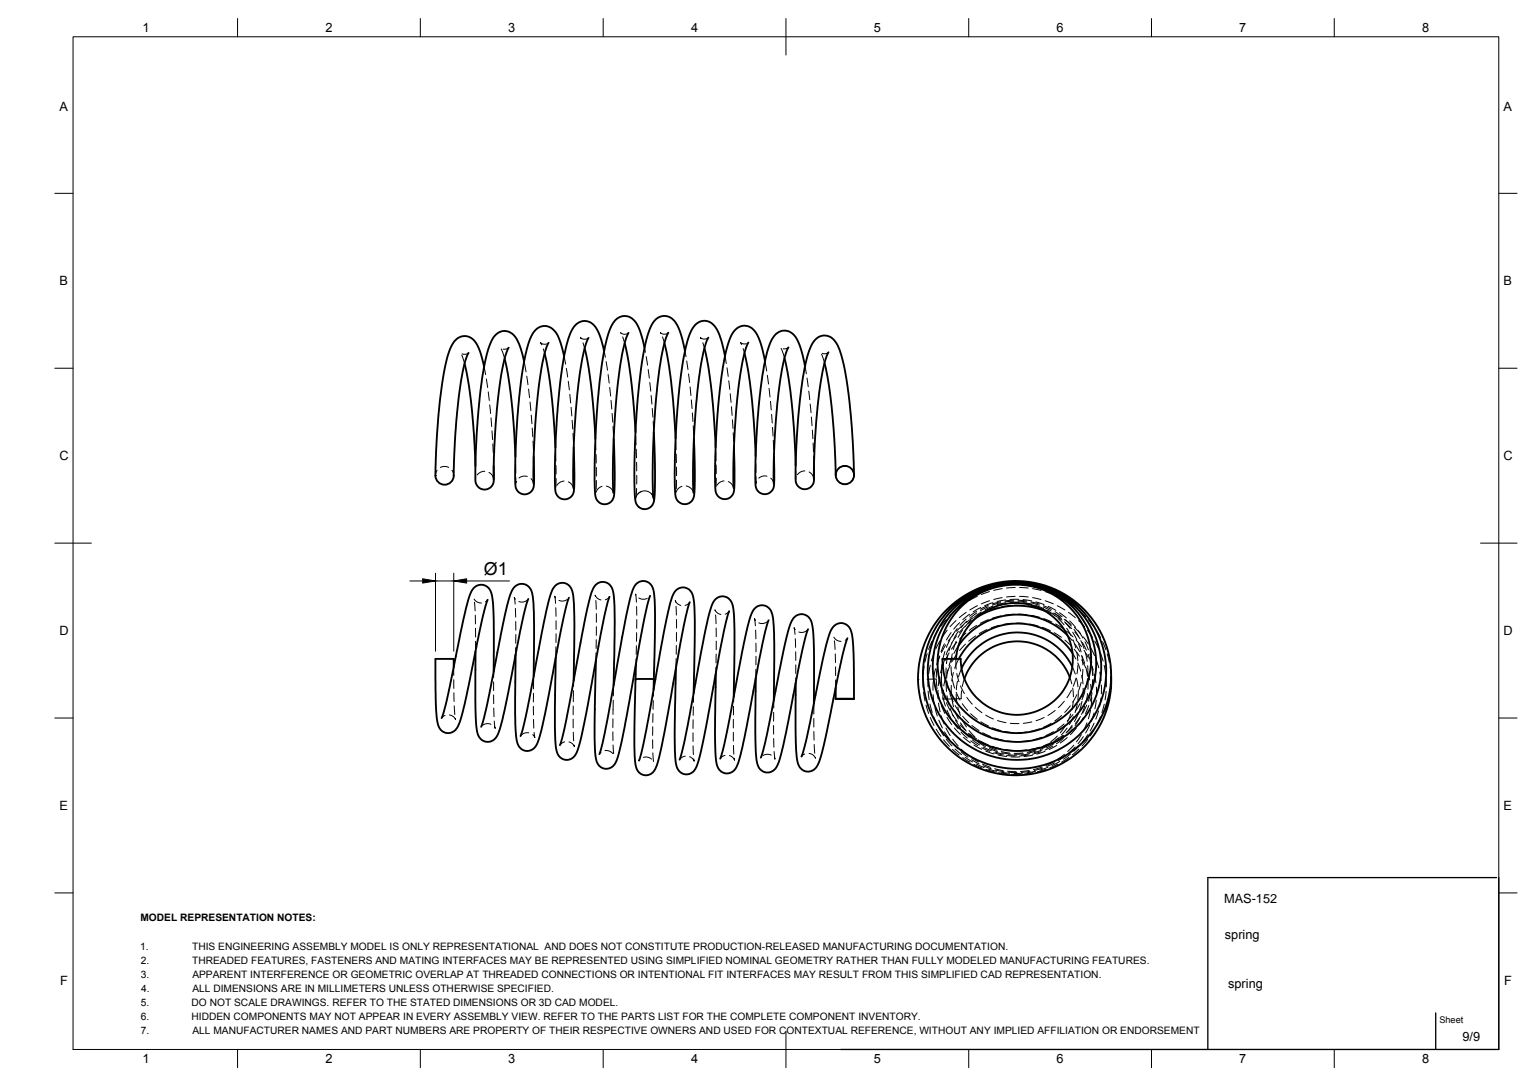
ISO-10303-21;
HEADER;
/* Generated by software containing ST-Developer
 * from STEP Tools, Inc. (www.steptools.com) 
 */

FILE_DESCRIPTION(
/* description */ ('STEP AP214'),
/* implementation_level */ '2;1');

FILE_NAME(
/* name */ 'spring.step',
/* time_stamp */ '2026-11-04T19:18:53-08:00',
/* author */ (''),
/* organization */ (''),
/* preprocessor_version */ 'ST-DEVELOPER v20.2',
/* originating_system */ 'Autodesk Translation Framework v15.17.0.0',
/* authorisation */ '');

FILE_SCHEMA (('AUTOMOTIVE_DESIGN { 1 0 10303 214 3 1 1 }'));
ENDSEC;

DATA;
#10=MECHANICAL_DESIGN_GEOMETRIC_PRESENTATION_REPRESENTATION('',(#80),#5942);
#55=B_SPLINE_CURVE_WITH_KNOTS('',3,(#2155,#2156,#2157,#2158,#2159,#2160,
#2161,#2162,#2163,#2164,#2165,#2166,#2167,#2168,#2169,#2170,#2171,#2172,
#2173,#2174,#2175,#2176,#2177,#2178,#2179,#2180,#2181,#2182,#2183,#2184,
#2185,#2186,#2187,#2188,#2189,#2190,#2191,#2192,#2193,#2194,#2195,#2196,
#2197,#2198,#2199,#2200,#2201,#2202,#2203,#2204,#2205,#2206,#2207,#2208,
#2209,#2210,#2211,#2212,#2213,#2214,#2215,#2216,#2217,#2218,#2219,#2220,
#2221,#2222,#2223,#2224,#2225,#2226,#2227,#2228,#2229,#2230,#2231,#2232,
#2233,#2234,#2235,#2236,#2237,#2238,#2239,#2240,#2241,#2242,#2243,#2244,
#2245,#2246,#2247,#2248,#2249,#2250,#2251,#2252,#2253,#2254,#2255,#2256,
#2257,#2258,#2259,#2260,#2261,#2262,#2263,#2264,#2265,#2266,#2267,#2268,
#2269,#2270,#2271,#2272,#2273,#2274,#2275,#2276,#2277,#2278,#2279,#2280,
#2281,#2282,#2283,#2284,#2285,#2286,#2287,#2288,#2289,#2290,#2291,#2292,
#2293,#2294,#2295,#2296,#2297,#2298,#2299,#2300,#2301,#2302,#2303,#2304,
#2305,#2306,#2307,#2308),.UNSPECIFIED.,.F.,.F.,(4,3,3,3,3,3,3,3,3,3,3,3,
3,3,3,3,3,3,3,3,3,3,3,3,3,3,3,3,3,3,3,3,3,3,3,3,3,3,3,3,3,3,3,3,3,3,3,3,
3,3,3,4),(8.16441129645516E-18,0.0155213821795324,0.0465641465385971,0.0776069108976618,
0.108649675256726,0.139692439615791,0.170735203974856,0.201777968333921,
0.232820732692985,0.26386349705205,0.294906261411162,0.325949025770274,
0.356991790129291,0.388034554488308,0.419077318847373,0.450120083206437,
0.46564146538597,0.481162847565502,0.496684229745034,0.512205611924566,
0.527726994104099,0.543248376283631,0.558769758463163,0.574291140642696,
0.589812522822228,0.605333905001761,0.620855287181293,0.636376669360825,
0.651898051540357,0.66741943371989,0.682940815899422,0.698462198078954,
0.713983580258487,0.729504962438019,0.745026344617551,0.760547726797084,
0.776069108976616,0.791590491156148,0.807111873335681,0.822633255515213,
0.838154637694745,0.853676019874278,0.86919740205381,0.884718784233342,
0.900240166412875,0.915761548592407,0.931282930771939,0.946804312951471,
0.973402156475736,0.986701078237868,0.993350539118934,0.993460673612188),
 .UNSPECIFIED.);
#56=B_SPLINE_CURVE_WITH_KNOTS('',3,(#2313,#2314,#2315,#2316,#2317,#2318,
#2319,#2320,#2321,#2322,#2323,#2324,#2325,#2326,#2327,#2328,#2329,#2330,
#2331,#2332,#2333,#2334,#2335,#2336,#2337,#2338,#2339,#2340,#2341,#2342,
#2343,#2344,#2345,#2346,#2347,#2348,#2349,#2350,#2351,#2352,#2353,#2354,
#2355,#2356,#2357,#2358,#2359,#2360,#2361,#2362,#2363,#2364,#2365,#2366,
#2367,#2368,#2369,#2370,#2371,#2372,#2373,#2374,#2375,#2376,#2377,#2378,
#2379,#2380,#2381,#2382,#2383,#2384,#2385,#2386,#2387,#2388,#2389,#2390,
#2391,#2392,#2393,#2394,#2395,#2396,#2397,#2398,#2399,#2400,#2401,#2402,
#2403,#2404,#2405,#2406,#2407,#2408,#2409,#2410,#2411,#2412,#2413,#2414,
#2415,#2416,#2417,#2418,#2419,#2420,#2421,#2422,#2423,#2424,#2425,#2426,
#2427,#2428,#2429,#2430,#2431,#2432,#2433,#2434,#2435,#2436,#2437,#2438,
#2439,#2440,#2441,#2442,#2443,#2444,#2445,#2446,#2447,#2448,#2449,#2450,
#2451,#2452,#2453,#2454,#2455,#2456,#2457,#2458,#2459,#2460,#2461,#2462,
#2463),.UNSPECIFIED.,.F.,.F.,(4,3,3,3,3,3,3,3,3,3,3,3,3,3,3,3,3,3,3,3,3,
3,3,3,3,3,3,3,3,3,3,3,3,3,3,3,3,3,3,3,3,3,3,3,3,3,3,3,3,3,4),(0.,0.0155213821795324,
0.0465641465385971,0.0776069108976618,0.108649675256726,0.139692439615791,
0.170735203974856,0.201777968333921,0.232820732692985,0.26386349705205,
0.294906261411162,0.325949025770274,0.356991790129291,0.388034554488308,
0.419077318847373,0.450120083206437,0.46564146538597,0.481162847565502,
0.496684229745034,0.512205611924566,0.527726994104099,0.543248376283631,
0.558769758463163,0.574291140642696,0.589812522822228,0.605333905001761,
0.620855287181293,0.636376669360825,0.651898051540357,0.66741943371989,
0.682940815899422,0.698462198078954,0.713983580258487,0.729504962438019,
0.745026344617551,0.760547726797084,0.776069108976616,0.791590491156148,
0.807111873335681,0.822633255515213,0.838154637694745,0.853676019874278,
0.86919740205381,0.884718784233342,0.900240166412875,0.915761548592407,
0.931282930771939,0.946804312951471,0.973402156475736,0.986701078237868,
0.993275477626297),.UNSPECIFIED.);
#57=B_SPLINE_CURVE_WITH_KNOTS('',3,(#3378,#3379,#3380,#3381,#3382,#3383,
#3384,#3385,#3386,#3387,#3388,#3389,#3390,#3391,#3392,#3393,#3394,#3395,
#3396,#3397,#3398,#3399,#3400,#3401,#3402,#3403,#3404,#3405,#3406,#3407,
#3408,#3409,#3410,#3411,#3412,#3413,#3414,#3415,#3416,#3417,#3418,#3419,
#3420,#3421,#3422,#3423,#3424,#3425,#3426,#3427,#3428,#3429,#3430,#3431,
#3432,#3433,#3434,#3435,#3436,#3437,#3438,#3439,#3440,#3441,#3442,#3443,
#3444,#3445,#3446,#3447,#3448,#3449,#3450,#3451,#3452,#3453,#3454,#3455,
#3456,#3457,#3458,#3459,#3460,#3461,#3462,#3463,#3464,#3465,#3466,#3467,
#3468,#3469,#3470,#3471,#3472,#3473,#3474,#3475,#3476,#3477,#3478,#3479,
#3480,#3481,#3482,#3483,#3484,#3485,#3486,#3487,#3488,#3489,#3490,#3491,
#3492,#3493,#3494,#3495,#3496,#3497,#3498,#3499,#3500,#3501,#3502,#3503,
#3504,#3505,#3506,#3507,#3508,#3509,#3510,#3511,#3512,#3513,#3514,#3515,
#3516,#3517,#3518,#3519,#3520,#3521,#3522,#3523,#3524,#3525,#3526,#3527,
#3528,#3529,#3530,#3531,#3532,#3533,#3534,#3535,#3536,#3537,#3538,#3539,
#3540,#3541,#3542,#3543,#3544,#3545,#3546,#3547,#3548,#3549,#3550,#3551,
#3552,#3553,#3554,#3555,#3556,#3557,#3558,#3559,#3560,#3561,#3562,#3563,
#3564,#3565,#3566,#3567,#3568,#3569,#3570),.UNSPECIFIED.,.F.,.F.,(4,3,3,
3,3,3,3,3,3,3,3,3,3,3,3,3,3,3,3,3,3,3,3,3,3,3,3,3,3,3,3,3,3,3,3,3,3,3,3,
3,3,3,3,3,3,3,3,3,3,3,3,3,3,3,3,3,3,3,3,3,3,3,3,3,4),(-3.92493609792139E-18,
0.015625,0.03125,0.046875,0.0625,0.078125,0.09375,0.109375,0.125,0.140625,
0.15625,0.171875,0.1875,0.203125,0.21875,0.234375,0.25,0.265625,0.28125,
0.296875,0.3125,0.328125,0.34375,0.359375,0.375,0.390625,0.40625,0.421875,
0.4375,0.453125,0.46875,0.484375,0.5,0.515625,0.53125,0.546875,0.5625,0.578125,
0.59375,0.609375,0.625,0.640625,0.65625,0.671875,0.6875,0.703125,0.71875,
0.734375,0.75,0.765625,0.78125,0.796875,0.8125,0.828125,0.84375,0.859375,
0.875,0.890625,0.90625,0.921875,0.9375,0.953125,0.96875,0.984375,1.),
 .UNSPECIFIED.);
#58=B_SPLINE_CURVE_WITH_KNOTS('',3,(#3572,#3573,#3574,#3575,#3576,#3577,
#3578,#3579,#3580,#3581,#3582,#3583,#3584,#3585,#3586,#3587,#3588,#3589,
#3590,#3591,#3592,#3593,#3594,#3595,#3596,#3597,#3598,#3599,#3600,#3601,
#3602,#3603,#3604,#3605,#3606,#3607,#3608,#3609,#3610,#3611,#3612,#3613,
#3614,#3615,#3616,#3617,#3618,#3619,#3620,#3621,#3622,#3623,#3624,#3625,
#3626,#3627,#3628,#3629,#3630,#3631,#3632,#3633,#3634,#3635,#3636,#3637,
#3638,#3639,#3640,#3641,#3642,#3643,#3644,#3645,#3646,#3647,#3648,#3649,
#3650,#3651,#3652,#3653,#3654,#3655,#3656,#3657,#3658,#3659,#3660,#3661,
#3662,#3663,#3664,#3665,#3666,#3667,#3668,#3669,#3670,#3671,#3672,#3673,
#3674,#3675,#3676,#3677,#3678,#3679,#3680,#3681,#3682,#3683,#3684,#3685,
#3686,#3687,#3688,#3689,#3690,#3691,#3692,#3693,#3694,#3695,#3696,#3697,
#3698,#3699,#3700,#3701,#3702,#3703,#3704,#3705,#3706,#3707,#3708,#3709,
#3710,#3711,#3712,#3713,#3714,#3715,#3716,#3717,#3718,#3719,#3720,#3721,
#3722,#3723,#3724,#3725,#3726,#3727,#3728,#3729,#3730,#3731,#3732,#3733,
#3734,#3735,#3736,#3737,#3738,#3739,#3740,#3741,#3742,#3743,#3744,#3745,
#3746,#3747,#3748,#3749,#3750,#3751,#3752,#3753,#3754,#3755,#3756,#3757,
#3758,#3759,#3760,#3761,#3762,#3763,#3764),.UNSPECIFIED.,.F.,.F.,(4,3,3,
3,3,3,3,3,3,3,3,3,3,3,3,3,3,3,3,3,3,3,3,3,3,3,3,3,3,3,3,3,3,3,3,3,3,3,3,
3,3,3,3,3,3,3,3,3,3,3,3,3,3,3,3,3,3,3,3,3,3,3,3,3,4),(0.,0.015625,0.03125,
0.046875,0.0625,0.078125,0.09375,0.109375,0.125,0.140625,0.15625,0.171875,
0.1875,0.203125,0.21875,0.234375,0.25,0.265625,0.28125,0.296875,0.3125,
0.328125,0.34375,0.359375,0.375,0.390625,0.40625,0.421875,0.4375,0.453125,
0.46875,0.484375,0.5,0.515625,0.53125,0.546875,0.5625,0.578125,0.59375,
0.609375,0.625,0.640625,0.65625,0.671875,0.6875,0.703125,0.71875,0.734375,
0.75,0.765625,0.78125,0.796875,0.8125,0.828125,0.84375,0.859375,0.875,0.890625,
0.90625,0.921875,0.9375,0.953125,0.96875,0.984375,1.),.UNSPECIFIED.);
#59=(
BOUNDED_SURFACE()
B_SPLINE_SURFACE(3,3,((#1423,#1424,#1425,#1426,#1427,#1428,#1429,#1430,
#1431,#1432,#1433,#1434,#1435,#1436,#1437,#1438,#1439,#1440,#1441,#1442,
#1443,#1444,#1445,#1446,#1447,#1448,#1449,#1450,#1451,#1452,#1453,#1454,
#1455,#1456,#1457,#1458,#1459,#1460,#1461,#1462,#1463,#1464,#1465,#1466,
#1467,#1468,#1469,#1470,#1471,#1472,#1473,#1474,#1475,#1476,#1477,#1478,
#1479,#1480,#1481,#1482,#1483,#1484,#1485,#1486,#1487,#1488,#1489,#1490,
#1491,#1492,#1493,#1494,#1495,#1496,#1497,#1498,#1499,#1500,#1501,#1502,
#1503,#1504,#1505,#1506,#1507,#1508,#1509,#1510,#1511,#1512,#1513,#1514,
#1515,#1516,#1517,#1518,#1519,#1520,#1521,#1522,#1523,#1524,#1525,#1526),
(#1527,#1528,#1529,#1530,#1531,#1532,#1533,#1534,#1535,#1536,#1537,#1538,
#1539,#1540,#1541,#1542,#1543,#1544,#1545,#1546,#1547,#1548,#1549,#1550,
#1551,#1552,#1553,#1554,#1555,#1556,#1557,#1558,#1559,#1560,#1561,#1562,
#1563,#1564,#1565,#1566,#1567,#1568,#1569,#1570,#1571,#1572,#1573,#1574,
#1575,#1576,#1577,#1578,#1579,#1580,#1581,#1582,#1583,#1584,#1585,#1586,
#1587,#1588,#1589,#1590,#1591,#1592,#1593,#1594,#1595,#1596,#1597,#1598,
#1599,#1600,#1601,#1602,#1603,#1604,#1605,#1606,#1607,#1608,#1609,#1610,
#1611,#1612,#1613,#1614,#1615,#1616,#1617,#1618,#1619,#1620,#1621,#1622,
#1623,#1624,#1625,#1626,#1627,#1628,#1629,#1630),(#1631,#1632,#1633,#1634,
#1635,#1636,#1637,#1638,#1639,#1640,#1641,#1642,#1643,#1644,#1645,#1646,
#1647,#1648,#1649,#1650,#1651,#1652,#1653,#1654,#1655,#1656,#1657,#1658,
#1659,#1660,#1661,#1662,#1663,#1664,#1665,#1666,#1667,#1668,#1669,#1670,
#1671,#1672,#1673,#1674,#1675,#1676,#1677,#1678,#1679,#1680,#1681,#1682,
#1683,#1684,#1685,#1686,#1687,#1688,#1689,#1690,#1691,#1692,#1693,#1694,
#1695,#1696,#1697,#1698,#1699,#1700,#1701,#1702,#1703,#1704,#1705,#1706,
#1707,#1708,#1709,#1710,#1711,#1712,#1713,#1714,#1715,#1716,#1717,#1718,
#1719,#1720,#1721,#1722,#1723,#1724,#1725,#1726,#1727,#1728,#1729,#1730,
#1731,#1732,#1733,#1734),(#1735,#1736,#1737,#1738,#1739,#1740,#1741,#1742,
#1743,#1744,#1745,#1746,#1747,#1748,#1749,#1750,#1751,#1752,#1753,#1754,
#1755,#1756,#1757,#1758,#1759,#1760,#1761,#1762,#1763,#1764,#1765,#1766,
#1767,#1768,#1769,#1770,#1771,#1772,#1773,#1774,#1775,#1776,#1777,#1778,
#1779,#1780,#1781,#1782,#1783,#1784,#1785,#1786,#1787,#1788,#1789,#1790,
#1791,#1792,#1793,#1794,#1795,#1796,#1797,#1798,#1799,#1800,#1801,#1802,
#1803,#1804,#1805,#1806,#1807,#1808,#1809,#1810,#1811,#1812,#1813,#1814,
#1815,#1816,#1817,#1818,#1819,#1820,#1821,#1822,#1823,#1824,#1825,#1826,
#1827,#1828,#1829,#1830,#1831,#1832,#1833,#1834,#1835,#1836,#1837,#1838),
(#1839,#1840,#1841,#1842,#1843,#1844,#1845,#1846,#1847,#1848,#1849,#1850,
#1851,#1852,#1853,#1854,#1855,#1856,#1857,#1858,#1859,#1860,#1861,#1862,
#1863,#1864,#1865,#1866,#1867,#1868,#1869,#1870,#1871,#1872,#1873,#1874,
#1875,#1876,#1877,#1878,#1879,#1880,#1881,#1882,#1883,#1884,#1885,#1886,
#1887,#1888,#1889,#1890,#1891,#1892,#1893,#1894,#1895,#1896,#1897,#1898,
#1899,#1900,#1901,#1902,#1903,#1904,#1905,#1906,#1907,#1908,#1909,#1910,
#1911,#1912,#1913,#1914,#1915,#1916,#1917,#1918,#1919,#1920,#1921,#1922,
#1923,#1924,#1925,#1926,#1927,#1928,#1929,#1930,#1931,#1932,#1933,#1934,
#1935,#1936,#1937,#1938,#1939,#1940,#1941,#1942),(#1943,#1944,#1945,#1946,
#1947,#1948,#1949,#1950,#1951,#1952,#1953,#1954,#1955,#1956,#1957,#1958,
#1959,#1960,#1961,#1962,#1963,#1964,#1965,#1966,#1967,#1968,#1969,#1970,
#1971,#1972,#1973,#1974,#1975,#1976,#1977,#1978,#1979,#1980,#1981,#1982,
#1983,#1984,#1985,#1986,#1987,#1988,#1989,#1990,#1991,#1992,#1993,#1994,
#1995,#1996,#1997,#1998,#1999,#2000,#2001,#2002,#2003,#2004,#2005,#2006,
#2007,#2008,#2009,#2010,#2011,#2012,#2013,#2014,#2015,#2016,#2017,#2018,
#2019,#2020,#2021,#2022,#2023,#2024,#2025,#2026,#2027,#2028,#2029,#2030,
#2031,#2032,#2033,#2034,#2035,#2036,#2037,#2038,#2039,#2040,#2041,#2042,
#2043,#2044,#2045,#2046),(#2047,#2048,#2049,#2050,#2051,#2052,#2053,#2054,
#2055,#2056,#2057,#2058,#2059,#2060,#2061,#2062,#2063,#2064,#2065,#2066,
#2067,#2068,#2069,#2070,#2071,#2072,#2073,#2074,#2075,#2076,#2077,#2078,
#2079,#2080,#2081,#2082,#2083,#2084,#2085,#2086,#2087,#2088,#2089,#2090,
#2091,#2092,#2093,#2094,#2095,#2096,#2097,#2098,#2099,#2100,#2101,#2102,
#2103,#2104,#2105,#2106,#2107,#2108,#2109,#2110,#2111,#2112,#2113,#2114,
#2115,#2116,#2117,#2118,#2119,#2120,#2121,#2122,#2123,#2124,#2125,#2126,
#2127,#2128,#2129,#2130,#2131,#2132,#2133,#2134,#2135,#2136,#2137,#2138,
#2139,#2140,#2141,#2142,#2143,#2144,#2145,#2146,#2147,#2148,#2149,#2150)),
 .UNSPECIFIED.,.T.,.F.,.F.)
B_SPLINE_SURFACE_WITH_KNOTS((4,3,4),(4,2,2,2,2,2,2,2,2,2,2,2,2,2,2,2,2,
2,2,2,2,2,2,2,2,2,2,2,2,2,2,2,2,2,2,2,2,2,2,2,2,2,2,2,2,2,2,2,2,2,2,4),
(0.,0.5,1.),(0.,0.0155213821795324,0.0465641465385971,0.0776069108976618,
0.108649675256726,0.139692439615791,0.170735203974856,0.201777968333921,
0.232820732692985,0.26386349705205,0.294906261411162,0.325949025770274,
0.356991790129291,0.388034554488308,0.419077318847373,0.450120083206437,
0.46564146538597,0.481162847565502,0.496684229745034,0.512205611924566,
0.527726994104099,0.543248376283631,0.558769758463163,0.574291140642696,
0.589812522822228,0.605333905001761,0.620855287181293,0.636376669360825,
0.651898051540357,0.66741943371989,0.682940815899422,0.698462198078954,
0.713983580258487,0.729504962438019,0.745026344617551,0.760547726797084,
0.776069108976616,0.791590491156148,0.807111873335681,0.822633255515213,
0.838154637694745,0.853676019874278,0.86919740205381,0.884718784233342,
0.900240166412875,0.915761548592407,0.931282930771939,0.946804312951471,
0.973402156475736,0.986701078237868,0.993350539118934,1.),.UNSPECIFIED.)
GEOMETRIC_REPRESENTATION_ITEM()
RATIONAL_B_SPLINE_SURFACE(((1.,1.,1.,1.,1.,1.,1.,1.,1.,1.,1.,1.,1.,1.,1.,
1.,1.,1.,1.,1.,1.,1.,1.,1.,1.,1.,1.,1.,1.,1.,1.,1.,1.,1.,1.,1.,1.,1.,1.,
1.,1.,1.,1.,1.,1.,1.,1.,1.,1.,1.,1.,1.,1.,1.,1.,1.,1.,1.,1.,1.,1.,1.,1.,
1.,1.,1.,1.,1.,1.,1.,1.,1.,1.,1.,1.,1.,1.,1.,1.,1.,1.,1.,1.,1.,1.,1.,1.,
1.,1.,1.,1.,1.,1.,1.,1.,1.,1.,1.,1.,1.,1.,1.,1.,1.),(0.333333333333333,
0.333333333333333,0.333333333333333,0.333333333333333,0.333333333333333,
0.333333333333333,0.333333333333333,0.333333333333333,0.333333333333333,
0.333333333333333,0.333333333333333,0.333333333333333,0.333333333333333,
0.333333333333333,0.333333333333333,0.333333333333333,0.333333333333333,
0.333333333333333,0.333333333333333,0.333333333333333,0.333333333333333,
0.333333333333333,0.333333333333333,0.333333333333333,0.333333333333333,
0.333333333333333,0.333333333333333,0.333333333333333,0.333333333333333,
0.333333333333333,0.333333333333333,0.333333333333333,0.333333333333333,
0.333333333333333,0.333333333333333,0.333333333333333,0.333333333333333,
0.333333333333333,0.333333333333333,0.333333333333333,0.333333333333333,
0.333333333333333,0.333333333333333,0.333333333333333,0.333333333333333,
0.333333333333333,0.333333333333333,0.333333333333333,0.333333333333333,
0.333333333333333,0.333333333333333,0.333333333333333,0.333333333333333,
0.333333333333333,0.333333333333333,0.333333333333333,0.333333333333333,
0.333333333333333,0.333333333333333,0.333333333333333,0.333333333333333,
0.333333333333333,0.333333333333333,0.333333333333333,0.333333333333333,
0.333333333333333,0.333333333333333,0.333333333333333,0.333333333333333,
0.333333333333333,0.333333333333333,0.333333333333333,0.333333333333333,
0.333333333333333,0.333333333333333,0.333333333333333,0.333333333333333,
0.333333333333333,0.333333333333333,0.333333333333333,0.333333333333333,
0.333333333333333,0.333333333333333,0.333333333333333,0.333333333333333,
0.333333333333333,0.333333333333333,0.333333333333333,0.333333333333333,
0.333333333333333,0.333333333333333,0.333333333333333,0.333333333333333,
0.333333333333333,0.333333333333333,0.333333333333333,0.333333333333333,
0.333333333333333,0.333333333333333,0.333333333333333,0.333333333333333,
0.333333333333333,0.333333333333333,0.333333333333333),(0.333333333333333,
0.333333333333333,0.333333333333333,0.333333333333333,0.333333333333333,
0.333333333333333,0.333333333333333,0.333333333333333,0.333333333333333,
0.333333333333333,0.333333333333333,0.333333333333333,0.333333333333333,
0.333333333333333,0.333333333333333,0.333333333333333,0.333333333333333,
0.333333333333333,0.333333333333333,0.333333333333333,0.333333333333333,
0.333333333333333,0.333333333333333,0.333333333333333,0.333333333333333,
0.333333333333333,0.333333333333333,0.333333333333333,0.333333333333333,
0.333333333333333,0.333333333333333,0.333333333333333,0.333333333333333,
0.333333333333333,0.333333333333333,0.333333333333333,0.333333333333333,
0.333333333333333,0.333333333333333,0.333333333333333,0.333333333333333,
0.333333333333333,0.333333333333333,0.333333333333333,0.333333333333333,
0.333333333333333,0.333333333333333,0.333333333333333,0.333333333333333,
0.333333333333333,0.333333333333333,0.333333333333333,0.333333333333333,
0.333333333333333,0.333333333333333,0.333333333333333,0.333333333333333,
0.333333333333333,0.333333333333333,0.333333333333333,0.333333333333333,
0.333333333333333,0.333333333333333,0.333333333333333,0.333333333333333,
0.333333333333333,0.333333333333333,0.333333333333333,0.333333333333333,
0.333333333333333,0.333333333333333,0.333333333333333,0.333333333333333,
0.333333333333333,0.333333333333333,0.333333333333333,0.333333333333333,
0.333333333333333,0.333333333333333,0.333333333333333,0.333333333333333,
0.333333333333333,0.333333333333333,0.333333333333333,0.333333333333333,
0.333333333333333,0.333333333333333,0.333333333333333,0.333333333333333,
0.333333333333333,0.333333333333333,0.333333333333333,0.333333333333333,
0.333333333333333,0.333333333333333,0.333333333333333,0.333333333333333,
0.333333333333333,0.333333333333333,0.333333333333333,0.333333333333333,
0.333333333333333,0.333333333333333,0.333333333333333),(1.,1.,1.,1.,1.,
1.,1.,1.,1.,1.,1.,1.,1.,1.,1.,1.,1.,1.,1.,1.,1.,1.,1.,1.,1.,1.,1.,1.,1.,
1.,1.,1.,1.,1.,1.,1.,1.,1.,1.,1.,1.,1.,1.,1.,1.,1.,1.,1.,1.,1.,1.,1.,1.,
1.,1.,1.,1.,1.,1.,1.,1.,1.,1.,1.,1.,1.,1.,1.,1.,1.,1.,1.,1.,1.,1.,1.,1.,
1.,1.,1.,1.,1.,1.,1.,1.,1.,1.,1.,1.,1.,1.,1.,1.,1.,1.,1.,1.,1.,1.,1.,1.,
1.,1.,1.),(0.333333333333333,0.333333333333333,0.333333333333333,0.333333333333333,
0.333333333333333,0.333333333333333,0.333333333333333,0.333333333333333,
0.333333333333333,0.333333333333333,0.333333333333333,0.333333333333333,
0.333333333333333,0.333333333333333,0.333333333333333,0.333333333333333,
0.333333333333333,0.333333333333333,0.333333333333333,0.333333333333333,
0.333333333333333,0.333333333333333,0.333333333333333,0.333333333333333,
0.333333333333333,0.333333333333333,0.333333333333333,0.333333333333333,
0.333333333333333,0.333333333333333,0.333333333333333,0.333333333333333,
0.333333333333333,0.333333333333333,0.333333333333333,0.333333333333333,
0.333333333333333,0.333333333333333,0.333333333333333,0.333333333333333,
0.333333333333333,0.333333333333333,0.333333333333333,0.333333333333333,
0.333333333333333,0.333333333333333,0.333333333333333,0.333333333333333,
0.333333333333333,0.333333333333333,0.333333333333333,0.333333333333333,
0.333333333333333,0.333333333333333,0.333333333333333,0.333333333333333,
0.333333333333333,0.333333333333333,0.333333333333333,0.333333333333333,
0.333333333333333,0.333333333333333,0.333333333333333,0.333333333333333,
0.333333333333333,0.333333333333333,0.333333333333333,0.333333333333333,
0.333333333333333,0.333333333333333,0.333333333333333,0.333333333333333,
0.333333333333333,0.333333333333333,0.333333333333333,0.333333333333333,
0.333333333333333,0.333333333333333,0.333333333333333,0.333333333333333,
0.333333333333333,0.333333333333333,0.333333333333333,0.333333333333333,
0.333333333333333,0.333333333333333,0.333333333333333,0.333333333333333,
0.333333333333333,0.333333333333333,0.333333333333333,0.333333333333333,
0.333333333333333,0.333333333333333,0.333333333333333,0.333333333333333,
0.333333333333333,0.333333333333333,0.333333333333333,0.333333333333333,
0.333333333333333,0.333333333333333,0.333333333333333,0.333333333333333),
(0.333333333333333,0.333333333333333,0.333333333333333,0.333333333333333,
0.333333333333333,0.333333333333333,0.333333333333333,0.333333333333333,
0.333333333333333,0.333333333333333,0.333333333333333,0.333333333333333,
0.333333333333333,0.333333333333333,0.333333333333333,0.333333333333333,
0.333333333333333,0.333333333333333,0.333333333333333,0.333333333333333,
0.333333333333333,0.333333333333333,0.333333333333333,0.333333333333333,
0.333333333333333,0.333333333333333,0.333333333333333,0.333333333333333,
0.333333333333333,0.333333333333333,0.333333333333333,0.333333333333333,
0.333333333333333,0.333333333333333,0.333333333333333,0.333333333333333,
0.333333333333333,0.333333333333333,0.333333333333333,0.333333333333333,
0.333333333333333,0.333333333333333,0.333333333333333,0.333333333333333,
0.333333333333333,0.333333333333333,0.333333333333333,0.333333333333333,
0.333333333333333,0.333333333333333,0.333333333333333,0.333333333333333,
0.333333333333333,0.333333333333333,0.333333333333333,0.333333333333333,
0.333333333333333,0.333333333333333,0.333333333333333,0.333333333333333,
0.333333333333333,0.333333333333333,0.333333333333333,0.333333333333333,
0.333333333333333,0.333333333333333,0.333333333333333,0.333333333333333,
0.333333333333333,0.333333333333333,0.333333333333333,0.333333333333333,
0.333333333333333,0.333333333333333,0.333333333333333,0.333333333333333,
0.333333333333333,0.333333333333333,0.333333333333333,0.333333333333333,
0.333333333333333,0.333333333333333,0.333333333333333,0.333333333333333,
0.333333333333333,0.333333333333333,0.333333333333333,0.333333333333333,
0.333333333333333,0.333333333333333,0.333333333333333,0.333333333333333,
0.333333333333333,0.333333333333333,0.333333333333333,0.333333333333333,
0.333333333333333,0.333333333333333,0.333333333333333,0.333333333333333,
0.333333333333333,0.333333333333333,0.333333333333333,0.333333333333333),
(1.,1.,1.,1.,1.,1.,1.,1.,1.,1.,1.,1.,1.,1.,1.,1.,1.,1.,1.,1.,1.,1.,1.,1.,
1.,1.,1.,1.,1.,1.,1.,1.,1.,1.,1.,1.,1.,1.,1.,1.,1.,1.,1.,1.,1.,1.,1.,1.,
1.,1.,1.,1.,1.,1.,1.,1.,1.,1.,1.,1.,1.,1.,1.,1.,1.,1.,1.,1.,1.,1.,1.,1.,
1.,1.,1.,1.,1.,1.,1.,1.,1.,1.,1.,1.,1.,1.,1.,1.,1.,1.,1.,1.,1.,1.,1.,1.,
1.,1.,1.,1.,1.,1.,1.,1.)))
REPRESENTATION_ITEM('')
SURFACE()
);
#60=(
BOUNDED_SURFACE()
B_SPLINE_SURFACE(3,3,((#2464,#2465,#2466,#2467,#2468,#2469,#2470,#2471,
#2472,#2473,#2474,#2475,#2476,#2477,#2478,#2479,#2480,#2481,#2482,#2483,
#2484,#2485,#2486,#2487,#2488,#2489,#2490,#2491,#2492,#2493,#2494,#2495,
#2496,#2497,#2498,#2499,#2500,#2501,#2502,#2503,#2504,#2505,#2506,#2507,
#2508,#2509,#2510,#2511,#2512,#2513,#2514,#2515,#2516,#2517,#2518,#2519,
#2520,#2521,#2522,#2523,#2524,#2525,#2526,#2527,#2528,#2529,#2530,#2531,
#2532,#2533,#2534,#2535,#2536,#2537,#2538,#2539,#2540,#2541,#2542,#2543,
#2544,#2545,#2546,#2547,#2548,#2549,#2550,#2551,#2552,#2553,#2554,#2555,
#2556,#2557,#2558,#2559,#2560,#2561,#2562,#2563,#2564,#2565,#2566,#2567,
#2568,#2569,#2570,#2571,#2572,#2573,#2574,#2575,#2576,#2577,#2578,#2579,
#2580,#2581,#2582,#2583,#2584,#2585,#2586,#2587,#2588,#2589,#2590,#2591,
#2592,#2593),(#2594,#2595,#2596,#2597,#2598,#2599,#2600,#2601,#2602,#2603,
#2604,#2605,#2606,#2607,#2608,#2609,#2610,#2611,#2612,#2613,#2614,#2615,
#2616,#2617,#2618,#2619,#2620,#2621,#2622,#2623,#2624,#2625,#2626,#2627,
#2628,#2629,#2630,#2631,#2632,#2633,#2634,#2635,#2636,#2637,#2638,#2639,
#2640,#2641,#2642,#2643,#2644,#2645,#2646,#2647,#2648,#2649,#2650,#2651,
#2652,#2653,#2654,#2655,#2656,#2657,#2658,#2659,#2660,#2661,#2662,#2663,
#2664,#2665,#2666,#2667,#2668,#2669,#2670,#2671,#2672,#2673,#2674,#2675,
#2676,#2677,#2678,#2679,#2680,#2681,#2682,#2683,#2684,#2685,#2686,#2687,
#2688,#2689,#2690,#2691,#2692,#2693,#2694,#2695,#2696,#2697,#2698,#2699,
#2700,#2701,#2702,#2703,#2704,#2705,#2706,#2707,#2708,#2709,#2710,#2711,
#2712,#2713,#2714,#2715,#2716,#2717,#2718,#2719,#2720,#2721,#2722,#2723),
(#2724,#2725,#2726,#2727,#2728,#2729,#2730,#2731,#2732,#2733,#2734,#2735,
#2736,#2737,#2738,#2739,#2740,#2741,#2742,#2743,#2744,#2745,#2746,#2747,
#2748,#2749,#2750,#2751,#2752,#2753,#2754,#2755,#2756,#2757,#2758,#2759,
#2760,#2761,#2762,#2763,#2764,#2765,#2766,#2767,#2768,#2769,#2770,#2771,
#2772,#2773,#2774,#2775,#2776,#2777,#2778,#2779,#2780,#2781,#2782,#2783,
#2784,#2785,#2786,#2787,#2788,#2789,#2790,#2791,#2792,#2793,#2794,#2795,
#2796,#2797,#2798,#2799,#2800,#2801,#2802,#2803,#2804,#2805,#2806,#2807,
#2808,#2809,#2810,#2811,#2812,#2813,#2814,#2815,#2816,#2817,#2818,#2819,
#2820,#2821,#2822,#2823,#2824,#2825,#2826,#2827,#2828,#2829,#2830,#2831,
#2832,#2833,#2834,#2835,#2836,#2837,#2838,#2839,#2840,#2841,#2842,#2843,
#2844,#2845,#2846,#2847,#2848,#2849,#2850,#2851,#2852,#2853),(#2854,#2855,
#2856,#2857,#2858,#2859,#2860,#2861,#2862,#2863,#2864,#2865,#2866,#2867,
#2868,#2869,#2870,#2871,#2872,#2873,#2874,#2875,#2876,#2877,#2878,#2879,
#2880,#2881,#2882,#2883,#2884,#2885,#2886,#2887,#2888,#2889,#2890,#2891,
#2892,#2893,#2894,#2895,#2896,#2897,#2898,#2899,#2900,#2901,#2902,#2903,
#2904,#2905,#2906,#2907,#2908,#2909,#2910,#2911,#2912,#2913,#2914,#2915,
#2916,#2917,#2918,#2919,#2920,#2921,#2922,#2923,#2924,#2925,#2926,#2927,
#2928,#2929,#2930,#2931,#2932,#2933,#2934,#2935,#2936,#2937,#2938,#2939,
#2940,#2941,#2942,#2943,#2944,#2945,#2946,#2947,#2948,#2949,#2950,#2951,
#2952,#2953,#2954,#2955,#2956,#2957,#2958,#2959,#2960,#2961,#2962,#2963,
#2964,#2965,#2966,#2967,#2968,#2969,#2970,#2971,#2972,#2973,#2974,#2975,
#2976,#2977,#2978,#2979,#2980,#2981,#2982,#2983),(#2984,#2985,#2986,#2987,
#2988,#2989,#2990,#2991,#2992,#2993,#2994,#2995,#2996,#2997,#2998,#2999,
#3000,#3001,#3002,#3003,#3004,#3005,#3006,#3007,#3008,#3009,#3010,#3011,
#3012,#3013,#3014,#3015,#3016,#3017,#3018,#3019,#3020,#3021,#3022,#3023,
#3024,#3025,#3026,#3027,#3028,#3029,#3030,#3031,#3032,#3033,#3034,#3035,
#3036,#3037,#3038,#3039,#3040,#3041,#3042,#3043,#3044,#3045,#3046,#3047,
#3048,#3049,#3050,#3051,#3052,#3053,#3054,#3055,#3056,#3057,#3058,#3059,
#3060,#3061,#3062,#3063,#3064,#3065,#3066,#3067,#3068,#3069,#3070,#3071,
#3072,#3073,#3074,#3075,#3076,#3077,#3078,#3079,#3080,#3081,#3082,#3083,
#3084,#3085,#3086,#3087,#3088,#3089,#3090,#3091,#3092,#3093,#3094,#3095,
#3096,#3097,#3098,#3099,#3100,#3101,#3102,#3103,#3104,#3105,#3106,#3107,
#3108,#3109,#3110,#3111,#3112,#3113),(#3114,#3115,#3116,#3117,#3118,#3119,
#3120,#3121,#3122,#3123,#3124,#3125,#3126,#3127,#3128,#3129,#3130,#3131,
#3132,#3133,#3134,#3135,#3136,#3137,#3138,#3139,#3140,#3141,#3142,#3143,
#3144,#3145,#3146,#3147,#3148,#3149,#3150,#3151,#3152,#3153,#3154,#3155,
#3156,#3157,#3158,#3159,#3160,#3161,#3162,#3163,#3164,#3165,#3166,#3167,
#3168,#3169,#3170,#3171,#3172,#3173,#3174,#3175,#3176,#3177,#3178,#3179,
#3180,#3181,#3182,#3183,#3184,#3185,#3186,#3187,#3188,#3189,#3190,#3191,
#3192,#3193,#3194,#3195,#3196,#3197,#3198,#3199,#3200,#3201,#3202,#3203,
#3204,#3205,#3206,#3207,#3208,#3209,#3210,#3211,#3212,#3213,#3214,#3215,
#3216,#3217,#3218,#3219,#3220,#3221,#3222,#3223,#3224,#3225,#3226,#3227,
#3228,#3229,#3230,#3231,#3232,#3233,#3234,#3235,#3236,#3237,#3238,#3239,
#3240,#3241,#3242,#3243),(#3244,#3245,#3246,#3247,#3248,#3249,#3250,#3251,
#3252,#3253,#3254,#3255,#3256,#3257,#3258,#3259,#3260,#3261,#3262,#3263,
#3264,#3265,#3266,#3267,#3268,#3269,#3270,#3271,#3272,#3273,#3274,#3275,
#3276,#3277,#3278,#3279,#3280,#3281,#3282,#3283,#3284,#3285,#3286,#3287,
#3288,#3289,#3290,#3291,#3292,#3293,#3294,#3295,#3296,#3297,#3298,#3299,
#3300,#3301,#3302,#3303,#3304,#3305,#3306,#3307,#3308,#3309,#3310,#3311,
#3312,#3313,#3314,#3315,#3316,#3317,#3318,#3319,#3320,#3321,#3322,#3323,
#3324,#3325,#3326,#3327,#3328,#3329,#3330,#3331,#3332,#3333,#3334,#3335,
#3336,#3337,#3338,#3339,#3340,#3341,#3342,#3343,#3344,#3345,#3346,#3347,
#3348,#3349,#3350,#3351,#3352,#3353,#3354,#3355,#3356,#3357,#3358,#3359,
#3360,#3361,#3362,#3363,#3364,#3365,#3366,#3367,#3368,#3369,#3370,#3371,
#3372,#3373)),.UNSPECIFIED.,.T.,.F.,.F.)
B_SPLINE_SURFACE_WITH_KNOTS((4,3,4),(4,2,2,2,2,2,2,2,2,2,2,2,2,2,2,2,2,
2,2,2,2,2,2,2,2,2,2,2,2,2,2,2,2,2,2,2,2,2,2,2,2,2,2,2,2,2,2,2,2,2,2,2,2,
2,2,2,2,2,2,2,2,2,2,2,4),(-6.51498550334715E-7,0.5,0.99999934850145),(0.,
0.015625,0.03125,0.046875,0.0625,0.078125,0.09375,0.109375,0.125,0.140625,
0.15625,0.171875,0.1875,0.203125,0.21875,0.234375,0.25,0.265625,0.28125,
0.296875,0.3125,0.328125,0.34375,0.359375,0.375,0.390625,0.40625,0.421875,
0.4375,0.453125,0.46875,0.484375,0.5,0.515625,0.53125,0.546875,0.5625,0.578125,
0.59375,0.609375,0.625,0.640625,0.65625,0.671875,0.6875,0.703125,0.71875,
0.734375,0.75,0.765625,0.78125,0.796875,0.8125,0.828125,0.84375,0.859375,
0.875,0.890625,0.90625,0.921875,0.9375,0.953125,0.96875,0.984375,1.),
 .UNSPECIFIED.)
GEOMETRIC_REPRESENTATION_ITEM()
RATIONAL_B_SPLINE_SURFACE(((0.999997394009194,0.999997394009194,0.999997394009194,
0.999997394009194,0.999997394009194,0.999997394009194,0.999997394009194,
0.999997394009194,0.999997394009194,0.999997394009194,0.999997394009194,
0.999997394009194,0.999997394009194,0.999997394009194,0.999997394009194,
0.999997394009194,0.999997394009194,0.999997394009194,0.999997394009194,
0.999997394009194,0.999997394009194,0.999997394009194,0.999997394009194,
0.999997394009194,0.999997394009194,0.999997394009194,0.999997394009194,
0.999997394009194,0.999997394009194,0.999997394009194,0.999997394009194,
0.999997394009194,0.999997394009194,0.999997394009194,0.999997394009194,
0.999997394009194,0.999997394009194,0.999997394009194,0.999997394009194,
0.999997394009194,0.999997394009194,0.999997394009194,0.999997394009194,
0.999997394009194,0.999997394009194,0.999997394009194,0.999997394009194,
0.999997394009194,0.999997394009194,0.999997394009194,0.999997394009194,
0.999997394009194,0.999997394009194,0.999997394009194,0.999997394009194,
0.999997394009194,0.999997394009194,0.999997394009194,0.999997394009194,
0.999997394009194,0.999997394009194,0.999997394009194,0.999997394009194,
0.999997394009194,0.999997394009194,0.999997394009194,0.999997394009194,
0.999997394009194,0.999997394009194,0.999997394009194,0.999997394009194,
0.999997394009194,0.999997394009194,0.999997394009194,0.999997394009194,
0.999997394009194,0.999997394009194,0.999997394009194,0.999997394009194,
0.999997394009194,0.999997394009194,0.999997394009194,0.999997394009194,
0.999997394009194,0.999997394009194,0.999997394009194,0.999997394009194,
0.999997394009194,0.999997394009194,0.999997394009194,0.999997394009194,
0.999997394009194,0.999997394009194,0.999997394009194,0.999997394009194,
0.999997394009194,0.999997394009194,0.999997394009194,0.999997394009194,
0.999997394009194,0.999997394009194,0.999997394009194,0.999997394009194,
0.999997394009194,0.999997394009194,0.999997394009194,0.999997394009194,
0.999997394009194,0.999997394009194,0.999997394009194,0.999997394009194,
0.999997394009194,0.999997394009194,0.999997394009194,0.999997394009194,
0.999997394009194,0.999997394009194,0.999997394009194,0.999997394009194,
0.999997394009194,0.999997394009194,0.999997394009194,0.999997394009194,
0.999997394009194,0.999997394009194,0.999997394009194,0.999997394009194,
0.999997394009194,0.999997394009194,0.999997394009194),(0.333333333333333,
0.333333333333333,0.333333333333333,0.333333333333333,0.333333333333333,
0.333333333333333,0.333333333333333,0.333333333333333,0.333333333333333,
0.333333333333333,0.333333333333333,0.333333333333333,0.333333333333333,
0.333333333333333,0.333333333333333,0.333333333333333,0.333333333333333,
0.333333333333333,0.333333333333333,0.333333333333333,0.333333333333333,
0.333333333333333,0.333333333333333,0.333333333333333,0.333333333333333,
0.333333333333333,0.333333333333333,0.333333333333333,0.333333333333333,
0.333333333333333,0.333333333333333,0.333333333333333,0.333333333333333,
0.333333333333333,0.333333333333333,0.333333333333333,0.333333333333333,
0.333333333333333,0.333333333333333,0.333333333333333,0.333333333333333,
0.333333333333333,0.333333333333333,0.333333333333333,0.333333333333333,
0.333333333333333,0.333333333333333,0.333333333333333,0.333333333333333,
0.333333333333333,0.333333333333333,0.333333333333333,0.333333333333333,
0.333333333333333,0.333333333333333,0.333333333333333,0.333333333333333,
0.333333333333333,0.333333333333333,0.333333333333333,0.333333333333333,
0.333333333333333,0.333333333333333,0.333333333333333,0.333333333333333,
0.333333333333333,0.333333333333333,0.333333333333333,0.333333333333333,
0.333333333333333,0.333333333333333,0.333333333333333,0.333333333333333,
0.333333333333333,0.333333333333333,0.333333333333333,0.333333333333333,
0.333333333333333,0.333333333333333,0.333333333333333,0.333333333333333,
0.333333333333333,0.333333333333333,0.333333333333333,0.333333333333333,
0.333333333333333,0.333333333333333,0.333333333333333,0.333333333333333,
0.333333333333333,0.333333333333333,0.333333333333333,0.333333333333333,
0.333333333333333,0.333333333333333,0.333333333333333,0.333333333333333,
0.333333333333333,0.333333333333333,0.333333333333333,0.333333333333333,
0.333333333333333,0.333333333333333,0.333333333333333,0.333333333333333,
0.333333333333333,0.333333333333333,0.333333333333333,0.333333333333333,
0.333333333333333,0.333333333333333,0.333333333333333,0.333333333333333,
0.333333333333333,0.333333333333333,0.333333333333333,0.333333333333333,
0.333333333333333,0.333333333333333,0.333333333333333,0.333333333333333,
0.333333333333333,0.333333333333333,0.333333333333333,0.333333333333333,
0.333333333333333,0.333333333333333,0.333333333333333,0.333333333333333,
0.333333333333333),(0.333333333333333,0.333333333333333,0.333333333333333,
0.333333333333333,0.333333333333333,0.333333333333333,0.333333333333333,
0.333333333333333,0.333333333333333,0.333333333333333,0.333333333333333,
0.333333333333333,0.333333333333333,0.333333333333333,0.333333333333333,
0.333333333333333,0.333333333333333,0.333333333333333,0.333333333333333,
0.333333333333333,0.333333333333333,0.333333333333333,0.333333333333333,
0.333333333333333,0.333333333333333,0.333333333333333,0.333333333333333,
0.333333333333333,0.333333333333333,0.333333333333333,0.333333333333333,
0.333333333333333,0.333333333333333,0.333333333333333,0.333333333333333,
0.333333333333333,0.333333333333333,0.333333333333333,0.333333333333333,
0.333333333333333,0.333333333333333,0.333333333333333,0.333333333333333,
0.333333333333333,0.333333333333333,0.333333333333333,0.333333333333333,
0.333333333333333,0.333333333333333,0.333333333333333,0.333333333333333,
0.333333333333333,0.333333333333333,0.333333333333333,0.333333333333333,
0.333333333333333,0.333333333333333,0.333333333333333,0.333333333333333,
0.333333333333333,0.333333333333333,0.333333333333333,0.333333333333333,
0.333333333333333,0.333333333333333,0.333333333333333,0.333333333333333,
0.333333333333333,0.333333333333333,0.333333333333333,0.333333333333333,
0.333333333333333,0.333333333333333,0.333333333333333,0.333333333333333,
0.333333333333333,0.333333333333333,0.333333333333333,0.333333333333333,
0.333333333333333,0.333333333333333,0.333333333333333,0.333333333333333,
0.333333333333333,0.333333333333333,0.333333333333333,0.333333333333333,
0.333333333333333,0.333333333333333,0.333333333333333,0.333333333333333,
0.333333333333333,0.333333333333333,0.333333333333333,0.333333333333333,
0.333333333333333,0.333333333333333,0.333333333333333,0.333333333333333,
0.333333333333333,0.333333333333333,0.333333333333333,0.333333333333333,
0.333333333333333,0.333333333333333,0.333333333333333,0.333333333333333,
0.333333333333333,0.333333333333333,0.333333333333333,0.333333333333333,
0.333333333333333,0.333333333333333,0.333333333333333,0.333333333333333,
0.333333333333333,0.333333333333333,0.333333333333333,0.333333333333333,
0.333333333333333,0.333333333333333,0.333333333333333,0.333333333333333,
0.333333333333333,0.333333333333333,0.333333333333333,0.333333333333333,
0.333333333333333,0.333333333333333,0.333333333333333),(1.,1.,1.,1.,1.,
1.,1.,1.,1.,1.,1.,1.,1.,1.,1.,1.,1.,1.,1.,1.,1.,1.,1.,1.,1.,1.,1.,1.,1.,
1.,1.,1.,1.,1.,1.,1.,1.,1.,1.,1.,1.,1.,1.,1.,1.,1.,1.,1.,1.,1.,1.,1.,1.,
1.,1.,1.,1.,1.,1.,1.,1.,1.,1.,1.,1.,1.,1.,1.,1.,1.,1.,1.,1.,1.,1.,1.,1.,
1.,1.,1.,1.,1.,1.,1.,1.,1.,1.,1.,1.,1.,1.,1.,1.,1.,1.,1.,1.,1.,1.,1.,1.,
1.,1.,1.,1.,1.,1.,1.,1.,1.,1.,1.,1.,1.,1.,1.,1.,1.,1.,1.,1.,1.,1.,1.,1.,
1.,1.,1.,1.,1.),(0.333334201998067,0.333334201998067,0.333334201998067,
0.333334201998067,0.333334201998067,0.333334201998067,0.333334201998067,
0.333334201998067,0.333334201998067,0.333334201998067,0.333334201998067,
0.333334201998067,0.333334201998067,0.333334201998067,0.333334201998067,
0.333334201998067,0.333334201998067,0.333334201998067,0.333334201998067,
0.333334201998067,0.333334201998067,0.333334201998067,0.333334201998067,
0.333334201998067,0.333334201998067,0.333334201998067,0.333334201998067,
0.333334201998067,0.333334201998067,0.333334201998067,0.333334201998067,
0.333334201998067,0.333334201998067,0.333334201998067,0.333334201998067,
0.333334201998067,0.333334201998067,0.333334201998067,0.333334201998067,
0.333334201998067,0.333334201998067,0.333334201998067,0.333334201998067,
0.333334201998067,0.333334201998067,0.333334201998067,0.333334201998067,
0.333334201998067,0.333334201998067,0.333334201998067,0.333334201998067,
0.333334201998067,0.333334201998067,0.333334201998067,0.333334201998067,
0.333334201998067,0.333334201998067,0.333334201998067,0.333334201998067,
0.333334201998067,0.333334201998067,0.333334201998067,0.333334201998067,
0.333334201998067,0.333334201998067,0.333334201998067,0.333334201998067,
0.333334201998067,0.333334201998067,0.333334201998067,0.333334201998067,
0.333334201998067,0.333334201998067,0.333334201998067,0.333334201998067,
0.333334201998067,0.333334201998067,0.333334201998067,0.333334201998067,
0.333334201998067,0.333334201998067,0.333334201998067,0.333334201998067,
0.333334201998067,0.333334201998067,0.333334201998067,0.333334201998067,
0.333334201998067,0.333334201998067,0.333334201998067,0.333334201998067,
0.333334201998067,0.333334201998067,0.333334201998067,0.333334201998067,
0.333334201998067,0.333334201998067,0.333334201998067,0.333334201998067,
0.333334201998067,0.333334201998067,0.333334201998067,0.333334201998067,
0.333334201998067,0.333334201998067,0.333334201998067,0.333334201998067,
0.333334201998067,0.333334201998067,0.333334201998067,0.333334201998067,
0.333334201998067,0.333334201998067,0.333334201998067,0.333334201998067,
0.333334201998067,0.333334201998067,0.333334201998067,0.333334201998067,
0.333334201998067,0.333334201998067,0.333334201998067,0.333334201998067,
0.333334201998067,0.333334201998067,0.333334201998067,0.333334201998067,
0.333334201998067,0.333334201998067,0.333334201998067),(0.333333333334465,
0.333333333334465,0.333333333334465,0.333333333334465,0.333333333334465,
0.333333333334465,0.333333333334465,0.333333333334465,0.333333333334465,
0.333333333334465,0.333333333334465,0.333333333334465,0.333333333334465,
0.333333333334465,0.333333333334465,0.333333333334465,0.333333333334465,
0.333333333334465,0.333333333334465,0.333333333334465,0.333333333334465,
0.333333333334465,0.333333333334465,0.333333333334465,0.333333333334465,
0.333333333334465,0.333333333334465,0.333333333334465,0.333333333334465,
0.333333333334465,0.333333333334465,0.333333333334465,0.333333333334465,
0.333333333334465,0.333333333334465,0.333333333334465,0.333333333334465,
0.333333333334465,0.333333333334465,0.333333333334465,0.333333333334465,
0.333333333334465,0.333333333334465,0.333333333334465,0.333333333334465,
0.333333333334465,0.333333333334465,0.333333333334465,0.333333333334465,
0.333333333334465,0.333333333334465,0.333333333334465,0.333333333334465,
0.333333333334465,0.333333333334465,0.333333333334465,0.333333333334465,
0.333333333334465,0.333333333334465,0.333333333334465,0.333333333334465,
0.333333333334465,0.333333333334465,0.333333333334465,0.333333333334465,
0.333333333334465,0.333333333334465,0.333333333334465,0.333333333334465,
0.333333333334465,0.333333333334465,0.333333333334465,0.333333333334465,
0.333333333334465,0.333333333334465,0.333333333334465,0.333333333334465,
0.333333333334465,0.333333333334465,0.333333333334465,0.333333333334465,
0.333333333334465,0.333333333334465,0.333333333334465,0.333333333334465,
0.333333333334465,0.333333333334465,0.333333333334465,0.333333333334465,
0.333333333334465,0.333333333334465,0.333333333334465,0.333333333334465,
0.333333333334465,0.333333333334465,0.333333333334465,0.333333333334465,
0.333333333334465,0.333333333334465,0.333333333334465,0.333333333334465,
0.333333333334465,0.333333333334465,0.333333333334465,0.333333333334465,
0.333333333334465,0.333333333334465,0.333333333334465,0.333333333334465,
0.333333333334465,0.333333333334465,0.333333333334465,0.333333333334465,
0.333333333334465,0.333333333334465,0.333333333334465,0.333333333334465,
0.333333333334465,0.333333333334465,0.333333333334465,0.333333333334465,
0.333333333334465,0.333333333334465,0.333333333334465,0.333333333334465,
0.333333333334465,0.333333333334465,0.333333333334465,0.333333333334465,
0.333333333334465),(0.999997394009194,0.999997394009194,0.999997394009194,
0.999997394009194,0.999997394009194,0.999997394009194,0.999997394009194,
0.999997394009194,0.999997394009194,0.999997394009194,0.999997394009194,
0.999997394009194,0.999997394009194,0.999997394009194,0.999997394009194,
0.999997394009194,0.999997394009194,0.999997394009194,0.999997394009194,
0.999997394009194,0.999997394009194,0.999997394009194,0.999997394009194,
0.999997394009194,0.999997394009194,0.999997394009194,0.999997394009194,
0.999997394009194,0.999997394009194,0.999997394009194,0.999997394009194,
0.999997394009194,0.999997394009194,0.999997394009194,0.999997394009194,
0.999997394009194,0.999997394009194,0.999997394009194,0.999997394009194,
0.999997394009194,0.999997394009194,0.999997394009194,0.999997394009194,
0.999997394009194,0.999997394009194,0.999997394009194,0.999997394009194,
0.999997394009194,0.999997394009194,0.999997394009194,0.999997394009194,
0.999997394009194,0.999997394009194,0.999997394009194,0.999997394009194,
0.999997394009194,0.999997394009194,0.999997394009194,0.999997394009194,
0.999997394009194,0.999997394009194,0.999997394009194,0.999997394009194,
0.999997394009194,0.999997394009194,0.999997394009194,0.999997394009194,
0.999997394009194,0.999997394009194,0.999997394009194,0.999997394009194,
0.999997394009194,0.999997394009194,0.999997394009194,0.999997394009194,
0.999997394009194,0.999997394009194,0.999997394009194,0.999997394009194,
0.999997394009194,0.999997394009194,0.999997394009194,0.999997394009194,
0.999997394009194,0.999997394009194,0.999997394009194,0.999997394009194,
0.999997394009194,0.999997394009194,0.999997394009194,0.999997394009194,
0.999997394009194,0.999997394009194,0.999997394009194,0.999997394009194,
0.999997394009194,0.999997394009194,0.999997394009194,0.999997394009194,
0.999997394009194,0.999997394009194,0.999997394009194,0.999997394009194,
0.999997394009194,0.999997394009194,0.999997394009194,0.999997394009194,
0.999997394009194,0.999997394009194,0.999997394009194,0.999997394009194,
0.999997394009194,0.999997394009194,0.999997394009194,0.999997394009194,
0.999997394009194,0.999997394009194,0.999997394009194,0.999997394009194,
0.999997394009194,0.999997394009194,0.999997394009194,0.999997394009194,
0.999997394009194,0.999997394009194,0.999997394009194,0.999997394009194,
0.999997394009194,0.999997394009194,0.999997394009194)))
REPRESENTATION_ITEM('')
SURFACE()
);
#61=(
BOUNDED_SURFACE()
B_SPLINE_SURFACE(3,3,((#3765,#3766,#3767,#3768,#3769,#3770,#3771,#3772,
#3773,#3774,#3775,#3776,#3777,#3778,#3779,#3780,#3781,#3782,#3783,#3784,
#3785,#3786,#3787,#3788,#3789,#3790,#3791,#3792,#3793,#3794,#3795,#3796,
#3797,#3798,#3799,#3800,#3801,#3802,#3803,#3804,#3805,#3806,#3807,#3808,
#3809,#3810,#3811,#3812,#3813,#3814,#3815,#3816,#3817,#3818,#3819,#3820,
#3821,#3822,#3823,#3824,#3825,#3826,#3827,#3828,#3829,#3830,#3831,#3832,
#3833,#3834,#3835,#3836,#3837,#3838,#3839,#3840,#3841,#3842,#3843,#3844,
#3845,#3846,#3847,#3848,#3849,#3850,#3851,#3852,#3853,#3854,#3855,#3856,
#3857,#3858,#3859,#3860,#3861,#3862,#3863,#3864,#3865,#3866,#3867,#3868,
#3869,#3870,#3871,#3872,#3873,#3874,#3875,#3876,#3877,#3878,#3879,#3880,
#3881,#3882,#3883,#3884,#3885,#3886,#3887,#3888,#3889,#3890,#3891,#3892,
#3893,#3894),(#3895,#3896,#3897,#3898,#3899,#3900,#3901,#3902,#3903,#3904,
#3905,#3906,#3907,#3908,#3909,#3910,#3911,#3912,#3913,#3914,#3915,#3916,
#3917,#3918,#3919,#3920,#3921,#3922,#3923,#3924,#3925,#3926,#3927,#3928,
#3929,#3930,#3931,#3932,#3933,#3934,#3935,#3936,#3937,#3938,#3939,#3940,
#3941,#3942,#3943,#3944,#3945,#3946,#3947,#3948,#3949,#3950,#3951,#3952,
#3953,#3954,#3955,#3956,#3957,#3958,#3959,#3960,#3961,#3962,#3963,#3964,
#3965,#3966,#3967,#3968,#3969,#3970,#3971,#3972,#3973,#3974,#3975,#3976,
#3977,#3978,#3979,#3980,#3981,#3982,#3983,#3984,#3985,#3986,#3987,#3988,
#3989,#3990,#3991,#3992,#3993,#3994,#3995,#3996,#3997,#3998,#3999,#4000,
#4001,#4002,#4003,#4004,#4005,#4006,#4007,#4008,#4009,#4010,#4011,#4012,
#4013,#4014,#4015,#4016,#4017,#4018,#4019,#4020,#4021,#4022,#4023,#4024),
(#4025,#4026,#4027,#4028,#4029,#4030,#4031,#4032,#4033,#4034,#4035,#4036,
#4037,#4038,#4039,#4040,#4041,#4042,#4043,#4044,#4045,#4046,#4047,#4048,
#4049,#4050,#4051,#4052,#4053,#4054,#4055,#4056,#4057,#4058,#4059,#4060,
#4061,#4062,#4063,#4064,#4065,#4066,#4067,#4068,#4069,#4070,#4071,#4072,
#4073,#4074,#4075,#4076,#4077,#4078,#4079,#4080,#4081,#4082,#4083,#4084,
#4085,#4086,#4087,#4088,#4089,#4090,#4091,#4092,#4093,#4094,#4095,#4096,
#4097,#4098,#4099,#4100,#4101,#4102,#4103,#4104,#4105,#4106,#4107,#4108,
#4109,#4110,#4111,#4112,#4113,#4114,#4115,#4116,#4117,#4118,#4119,#4120,
#4121,#4122,#4123,#4124,#4125,#4126,#4127,#4128,#4129,#4130,#4131,#4132,
#4133,#4134,#4135,#4136,#4137,#4138,#4139,#4140,#4141,#4142,#4143,#4144,
#4145,#4146,#4147,#4148,#4149,#4150,#4151,#4152,#4153,#4154),(#4155,#4156,
#4157,#4158,#4159,#4160,#4161,#4162,#4163,#4164,#4165,#4166,#4167,#4168,
#4169,#4170,#4171,#4172,#4173,#4174,#4175,#4176,#4177,#4178,#4179,#4180,
#4181,#4182,#4183,#4184,#4185,#4186,#4187,#4188,#4189,#4190,#4191,#4192,
#4193,#4194,#4195,#4196,#4197,#4198,#4199,#4200,#4201,#4202,#4203,#4204,
#4205,#4206,#4207,#4208,#4209,#4210,#4211,#4212,#4213,#4214,#4215,#4216,
#4217,#4218,#4219,#4220,#4221,#4222,#4223,#4224,#4225,#4226,#4227,#4228,
#4229,#4230,#4231,#4232,#4233,#4234,#4235,#4236,#4237,#4238,#4239,#4240,
#4241,#4242,#4243,#4244,#4245,#4246,#4247,#4248,#4249,#4250,#4251,#4252,
#4253,#4254,#4255,#4256,#4257,#4258,#4259,#4260,#4261,#4262,#4263,#4264,
#4265,#4266,#4267,#4268,#4269,#4270,#4271,#4272,#4273,#4274,#4275,#4276,
#4277,#4278,#4279,#4280,#4281,#4282,#4283,#4284),(#4285,#4286,#4287,#4288,
#4289,#4290,#4291,#4292,#4293,#4294,#4295,#4296,#4297,#4298,#4299,#4300,
#4301,#4302,#4303,#4304,#4305,#4306,#4307,#4308,#4309,#4310,#4311,#4312,
#4313,#4314,#4315,#4316,#4317,#4318,#4319,#4320,#4321,#4322,#4323,#4324,
#4325,#4326,#4327,#4328,#4329,#4330,#4331,#4332,#4333,#4334,#4335,#4336,
#4337,#4338,#4339,#4340,#4341,#4342,#4343,#4344,#4345,#4346,#4347,#4348,
#4349,#4350,#4351,#4352,#4353,#4354,#4355,#4356,#4357,#4358,#4359,#4360,
#4361,#4362,#4363,#4364,#4365,#4366,#4367,#4368,#4369,#4370,#4371,#4372,
#4373,#4374,#4375,#4376,#4377,#4378,#4379,#4380,#4381,#4382,#4383,#4384,
#4385,#4386,#4387,#4388,#4389,#4390,#4391,#4392,#4393,#4394,#4395,#4396,
#4397,#4398,#4399,#4400,#4401,#4402,#4403,#4404,#4405,#4406,#4407,#4408,
#4409,#4410,#4411,#4412,#4413,#4414),(#4415,#4416,#4417,#4418,#4419,#4420,
#4421,#4422,#4423,#4424,#4425,#4426,#4427,#4428,#4429,#4430,#4431,#4432,
#4433,#4434,#4435,#4436,#4437,#4438,#4439,#4440,#4441,#4442,#4443,#4444,
#4445,#4446,#4447,#4448,#4449,#4450,#4451,#4452,#4453,#4454,#4455,#4456,
#4457,#4458,#4459,#4460,#4461,#4462,#4463,#4464,#4465,#4466,#4467,#4468,
#4469,#4470,#4471,#4472,#4473,#4474,#4475,#4476,#4477,#4478,#4479,#4480,
#4481,#4482,#4483,#4484,#4485,#4486,#4487,#4488,#4489,#4490,#4491,#4492,
#4493,#4494,#4495,#4496,#4497,#4498,#4499,#4500,#4501,#4502,#4503,#4504,
#4505,#4506,#4507,#4508,#4509,#4510,#4511,#4512,#4513,#4514,#4515,#4516,
#4517,#4518,#4519,#4520,#4521,#4522,#4523,#4524,#4525,#4526,#4527,#4528,
#4529,#4530,#4531,#4532,#4533,#4534,#4535,#4536,#4537,#4538,#4539,#4540,
#4541,#4542,#4543,#4544),(#4545,#4546,#4547,#4548,#4549,#4550,#4551,#4552,
#4553,#4554,#4555,#4556,#4557,#4558,#4559,#4560,#4561,#4562,#4563,#4564,
#4565,#4566,#4567,#4568,#4569,#4570,#4571,#4572,#4573,#4574,#4575,#4576,
#4577,#4578,#4579,#4580,#4581,#4582,#4583,#4584,#4585,#4586,#4587,#4588,
#4589,#4590,#4591,#4592,#4593,#4594,#4595,#4596,#4597,#4598,#4599,#4600,
#4601,#4602,#4603,#4604,#4605,#4606,#4607,#4608,#4609,#4610,#4611,#4612,
#4613,#4614,#4615,#4616,#4617,#4618,#4619,#4620,#4621,#4622,#4623,#4624,
#4625,#4626,#4627,#4628,#4629,#4630,#4631,#4632,#4633,#4634,#4635,#4636,
#4637,#4638,#4639,#4640,#4641,#4642,#4643,#4644,#4645,#4646,#4647,#4648,
#4649,#4650,#4651,#4652,#4653,#4654,#4655,#4656,#4657,#4658,#4659,#4660,
#4661,#4662,#4663,#4664,#4665,#4666,#4667,#4668,#4669,#4670,#4671,#4672,
#4673,#4674)),.UNSPECIFIED.,.T.,.F.,.F.)
B_SPLINE_SURFACE_WITH_KNOTS((4,3,4),(4,2,2,2,2,2,2,2,2,2,2,2,2,2,2,2,2,
2,2,2,2,2,2,2,2,2,2,2,2,2,2,2,2,2,2,2,2,2,2,2,2,2,2,2,2,2,2,2,2,2,2,2,2,
2,2,2,2,2,2,2,2,2,2,2,4),(0.499999335657285,1.,1.49999933565728),(0.,0.015625,
0.03125,0.046875,0.0625,0.078125,0.09375,0.109375,0.125,0.140625,0.15625,
0.171875,0.1875,0.203125,0.21875,0.234375,0.25,0.265625,0.28125,0.296875,
0.3125,0.328125,0.34375,0.359375,0.375,0.390625,0.40625,0.421875,0.4375,
0.453125,0.46875,0.484375,0.5,0.515625,0.53125,0.546875,0.5625,0.578125,
0.59375,0.609375,0.625,0.640625,0.65625,0.671875,0.6875,0.703125,0.71875,
0.734375,0.75,0.765625,0.78125,0.796875,0.8125,0.828125,0.84375,0.859375,
0.875,0.890625,0.90625,0.921875,0.9375,0.953125,0.96875,0.984375,1.),
 .UNSPECIFIED.)
GEOMETRIC_REPRESENTATION_ITEM()
RATIONAL_B_SPLINE_SURFACE(((0.999997342632669,0.999997342632669,0.999997342632669,
0.999997342632669,0.999997342632669,0.999997342632669,0.999997342632669,
0.999997342632669,0.999997342632669,0.999997342632669,0.999997342632669,
0.999997342632669,0.999997342632669,0.999997342632669,0.999997342632669,
0.999997342632669,0.999997342632669,0.999997342632669,0.999997342632669,
0.999997342632669,0.999997342632669,0.999997342632669,0.999997342632669,
0.999997342632669,0.999997342632669,0.999997342632669,0.999997342632669,
0.999997342632669,0.999997342632669,0.999997342632669,0.999997342632669,
0.999997342632669,0.999997342632669,0.999997342632669,0.999997342632669,
0.999997342632669,0.999997342632669,0.999997342632669,0.999997342632669,
0.999997342632669,0.999997342632669,0.999997342632669,0.999997342632669,
0.999997342632669,0.999997342632669,0.999997342632669,0.999997342632669,
0.999997342632669,0.999997342632669,0.999997342632669,0.999997342632669,
0.999997342632669,0.999997342632669,0.999997342632669,0.999997342632669,
0.999997342632669,0.999997342632669,0.999997342632669,0.999997342632669,
0.999997342632669,0.999997342632669,0.999997342632669,0.999997342632669,
0.999997342632669,0.999997342632669,0.999997342632669,0.999997342632669,
0.999997342632669,0.999997342632669,0.999997342632669,0.999997342632669,
0.999997342632669,0.999997342632669,0.999997342632669,0.999997342632669,
0.999997342632669,0.999997342632669,0.999997342632669,0.999997342632669,
0.999997342632669,0.999997342632669,0.999997342632669,0.999997342632669,
0.999997342632669,0.999997342632669,0.999997342632669,0.999997342632669,
0.999997342632669,0.999997342632669,0.999997342632669,0.999997342632669,
0.999997342632669,0.999997342632669,0.999997342632669,0.999997342632669,
0.999997342632669,0.999997342632669,0.999997342632669,0.999997342632669,
0.999997342632669,0.999997342632669,0.999997342632669,0.999997342632669,
0.999997342632669,0.999997342632669,0.999997342632669,0.999997342632669,
0.999997342632669,0.999997342632669,0.999997342632669,0.999997342632669,
0.999997342632669,0.999997342632669,0.999997342632669,0.999997342632669,
0.999997342632669,0.999997342632669,0.999997342632669,0.999997342632669,
0.999997342632669,0.999997342632669,0.999997342632669,0.999997342632669,
0.999997342632669,0.999997342632669,0.999997342632669,0.999997342632669,
0.999997342632669,0.999997342632669,0.999997342632669),(0.333333333333333,
0.333333333333333,0.333333333333333,0.333333333333333,0.333333333333333,
0.333333333333333,0.333333333333333,0.333333333333333,0.333333333333333,
0.333333333333333,0.333333333333333,0.333333333333333,0.333333333333333,
0.333333333333333,0.333333333333333,0.333333333333333,0.333333333333333,
0.333333333333333,0.333333333333333,0.333333333333333,0.333333333333333,
0.333333333333333,0.333333333333333,0.333333333333333,0.333333333333333,
0.333333333333333,0.333333333333333,0.333333333333333,0.333333333333333,
0.333333333333333,0.333333333333333,0.333333333333333,0.333333333333333,
0.333333333333333,0.333333333333333,0.333333333333333,0.333333333333333,
0.333333333333333,0.333333333333333,0.333333333333333,0.333333333333333,
0.333333333333333,0.333333333333333,0.333333333333333,0.333333333333333,
0.333333333333333,0.333333333333333,0.333333333333333,0.333333333333333,
0.333333333333333,0.333333333333333,0.333333333333333,0.333333333333333,
0.333333333333333,0.333333333333333,0.333333333333333,0.333333333333333,
0.333333333333333,0.333333333333333,0.333333333333333,0.333333333333333,
0.333333333333333,0.333333333333333,0.333333333333333,0.333333333333333,
0.333333333333333,0.333333333333333,0.333333333333333,0.333333333333333,
0.333333333333333,0.333333333333333,0.333333333333333,0.333333333333333,
0.333333333333333,0.333333333333333,0.333333333333333,0.333333333333333,
0.333333333333333,0.333333333333333,0.333333333333333,0.333333333333333,
0.333333333333333,0.333333333333333,0.333333333333333,0.333333333333333,
0.333333333333333,0.333333333333333,0.333333333333333,0.333333333333333,
0.333333333333333,0.333333333333333,0.333333333333333,0.333333333333333,
0.333333333333333,0.333333333333333,0.333333333333333,0.333333333333333,
0.333333333333333,0.333333333333333,0.333333333333333,0.333333333333333,
0.333333333333333,0.333333333333333,0.333333333333333,0.333333333333333,
0.333333333333333,0.333333333333333,0.333333333333333,0.333333333333333,
0.333333333333333,0.333333333333333,0.333333333333333,0.333333333333333,
0.333333333333333,0.333333333333333,0.333333333333333,0.333333333333333,
0.333333333333333,0.333333333333333,0.333333333333333,0.333333333333333,
0.333333333333333,0.333333333333333,0.333333333333333,0.333333333333333,
0.333333333333333,0.333333333333333,0.333333333333333,0.333333333333333,
0.333333333333333),(0.333333333333333,0.333333333333333,0.333333333333333,
0.333333333333333,0.333333333333333,0.333333333333333,0.333333333333333,
0.333333333333333,0.333333333333333,0.333333333333333,0.333333333333333,
0.333333333333333,0.333333333333333,0.333333333333333,0.333333333333333,
0.333333333333333,0.333333333333333,0.333333333333333,0.333333333333333,
0.333333333333333,0.333333333333333,0.333333333333333,0.333333333333333,
0.333333333333333,0.333333333333333,0.333333333333333,0.333333333333333,
0.333333333333333,0.333333333333333,0.333333333333333,0.333333333333333,
0.333333333333333,0.333333333333333,0.333333333333333,0.333333333333333,
0.333333333333333,0.333333333333333,0.333333333333333,0.333333333333333,
0.333333333333333,0.333333333333333,0.333333333333333,0.333333333333333,
0.333333333333333,0.333333333333333,0.333333333333333,0.333333333333333,
0.333333333333333,0.333333333333333,0.333333333333333,0.333333333333333,
0.333333333333333,0.333333333333333,0.333333333333333,0.333333333333333,
0.333333333333333,0.333333333333333,0.333333333333333,0.333333333333333,
0.333333333333333,0.333333333333333,0.333333333333333,0.333333333333333,
0.333333333333333,0.333333333333333,0.333333333333333,0.333333333333333,
0.333333333333333,0.333333333333333,0.333333333333333,0.333333333333333,
0.333333333333333,0.333333333333333,0.333333333333333,0.333333333333333,
0.333333333333333,0.333333333333333,0.333333333333333,0.333333333333333,
0.333333333333333,0.333333333333333,0.333333333333333,0.333333333333333,
0.333333333333333,0.333333333333333,0.333333333333333,0.333333333333333,
0.333333333333333,0.333333333333333,0.333333333333333,0.333333333333333,
0.333333333333333,0.333333333333333,0.333333333333333,0.333333333333333,
0.333333333333333,0.333333333333333,0.333333333333333,0.333333333333333,
0.333333333333333,0.333333333333333,0.333333333333333,0.333333333333333,
0.333333333333333,0.333333333333333,0.333333333333333,0.333333333333333,
0.333333333333333,0.333333333333333,0.333333333333333,0.333333333333333,
0.333333333333333,0.333333333333333,0.333333333333333,0.333333333333333,
0.333333333333333,0.333333333333333,0.333333333333333,0.333333333333333,
0.333333333333333,0.333333333333333,0.333333333333333,0.333333333333333,
0.333333333333333,0.333333333333333,0.333333333333333,0.333333333333333,
0.333333333333333,0.333333333333333,0.333333333333333),(1.,1.,1.,1.,1.,
1.,1.,1.,1.,1.,1.,1.,1.,1.,1.,1.,1.,1.,1.,1.,1.,1.,1.,1.,1.,1.,1.,1.,1.,
1.,1.,1.,1.,1.,1.,1.,1.,1.,1.,1.,1.,1.,1.,1.,1.,1.,1.,1.,1.,1.,1.,1.,1.,
1.,1.,1.,1.,1.,1.,1.,1.,1.,1.,1.,1.,1.,1.,1.,1.,1.,1.,1.,1.,1.,1.,1.,1.,
1.,1.,1.,1.,1.,1.,1.,1.,1.,1.,1.,1.,1.,1.,1.,1.,1.,1.,1.,1.,1.,1.,1.,1.,
1.,1.,1.,1.,1.,1.,1.,1.,1.,1.,1.,1.,1.,1.,1.,1.,1.,1.,1.,1.,1.,1.,1.,1.,
1.,1.,1.,1.,1.),(0.333334219123621,0.333334219123621,0.333334219123621,
0.333334219123621,0.333334219123621,0.333334219123621,0.333334219123621,
0.333334219123621,0.333334219123621,0.333334219123621,0.333334219123621,
0.333334219123621,0.333334219123621,0.333334219123621,0.333334219123621,
0.333334219123621,0.333334219123621,0.333334219123621,0.333334219123621,
0.333334219123621,0.333334219123621,0.333334219123621,0.333334219123621,
0.333334219123621,0.333334219123621,0.333334219123621,0.333334219123621,
0.333334219123621,0.333334219123621,0.333334219123621,0.333334219123621,
0.333334219123621,0.333334219123621,0.333334219123621,0.333334219123621,
0.333334219123621,0.333334219123621,0.333334219123621,0.333334219123621,
0.333334219123621,0.333334219123621,0.333334219123621,0.333334219123621,
0.333334219123621,0.333334219123621,0.333334219123621,0.333334219123621,
0.333334219123621,0.333334219123621,0.333334219123621,0.333334219123621,
0.333334219123621,0.333334219123621,0.333334219123621,0.333334219123621,
0.333334219123621,0.333334219123621,0.333334219123621,0.333334219123621,
0.333334219123621,0.333334219123621,0.333334219123621,0.333334219123621,
0.333334219123621,0.333334219123621,0.333334219123621,0.333334219123621,
0.333334219123621,0.333334219123621,0.333334219123621,0.333334219123621,
0.333334219123621,0.333334219123621,0.333334219123621,0.333334219123621,
0.333334219123621,0.333334219123621,0.333334219123621,0.333334219123621,
0.333334219123621,0.333334219123621,0.333334219123621,0.333334219123621,
0.333334219123621,0.333334219123621,0.333334219123621,0.333334219123621,
0.333334219123621,0.333334219123621,0.333334219123621,0.333334219123621,
0.333334219123621,0.333334219123621,0.333334219123621,0.333334219123621,
0.333334219123621,0.333334219123621,0.333334219123621,0.333334219123621,
0.333334219123621,0.333334219123621,0.333334219123621,0.333334219123621,
0.333334219123621,0.333334219123621,0.333334219123621,0.333334219123621,
0.333334219123621,0.333334219123621,0.333334219123621,0.333334219123621,
0.333334219123621,0.333334219123621,0.333334219123621,0.333334219123621,
0.333334219123621,0.333334219123621,0.333334219123621,0.333334219123621,
0.333334219123621,0.333334219123621,0.333334219123621,0.333334219123621,
0.333334219123621,0.333334219123621,0.333334219123621,0.333334219123621,
0.333334219123621,0.333334219123621,0.333334219123621),(0.33333333333451,
0.33333333333451,0.33333333333451,0.33333333333451,0.33333333333451,0.33333333333451,
0.33333333333451,0.33333333333451,0.33333333333451,0.33333333333451,0.33333333333451,
0.33333333333451,0.33333333333451,0.33333333333451,0.33333333333451,0.33333333333451,
0.33333333333451,0.33333333333451,0.33333333333451,0.33333333333451,0.33333333333451,
0.33333333333451,0.33333333333451,0.33333333333451,0.33333333333451,0.33333333333451,
0.33333333333451,0.33333333333451,0.33333333333451,0.33333333333451,0.33333333333451,
0.33333333333451,0.33333333333451,0.33333333333451,0.33333333333451,0.33333333333451,
0.33333333333451,0.33333333333451,0.33333333333451,0.33333333333451,0.33333333333451,
0.33333333333451,0.33333333333451,0.33333333333451,0.33333333333451,0.33333333333451,
0.33333333333451,0.33333333333451,0.33333333333451,0.33333333333451,0.33333333333451,
0.33333333333451,0.33333333333451,0.33333333333451,0.33333333333451,0.33333333333451,
0.33333333333451,0.33333333333451,0.33333333333451,0.33333333333451,0.33333333333451,
0.33333333333451,0.33333333333451,0.33333333333451,0.33333333333451,0.33333333333451,
0.33333333333451,0.33333333333451,0.33333333333451,0.33333333333451,0.33333333333451,
0.33333333333451,0.33333333333451,0.33333333333451,0.33333333333451,0.33333333333451,
0.33333333333451,0.33333333333451,0.33333333333451,0.33333333333451,0.33333333333451,
0.33333333333451,0.33333333333451,0.33333333333451,0.33333333333451,0.33333333333451,
0.33333333333451,0.33333333333451,0.33333333333451,0.33333333333451,0.33333333333451,
0.33333333333451,0.33333333333451,0.33333333333451,0.33333333333451,0.33333333333451,
0.33333333333451,0.33333333333451,0.33333333333451,0.33333333333451,0.33333333333451,
0.33333333333451,0.33333333333451,0.33333333333451,0.33333333333451,0.33333333333451,
0.33333333333451,0.33333333333451,0.33333333333451,0.33333333333451,0.33333333333451,
0.33333333333451,0.33333333333451,0.33333333333451,0.33333333333451,0.33333333333451,
0.33333333333451,0.33333333333451,0.33333333333451,0.33333333333451,0.33333333333451,
0.33333333333451,0.33333333333451,0.33333333333451,0.33333333333451,0.33333333333451,
0.33333333333451,0.33333333333451,0.33333333333451,0.33333333333451),(0.999997342632669,
0.999997342632669,0.999997342632669,0.999997342632669,0.999997342632669,
0.999997342632669,0.999997342632669,0.999997342632669,0.999997342632669,
0.999997342632669,0.999997342632669,0.999997342632669,0.999997342632669,
0.999997342632669,0.999997342632669,0.999997342632669,0.999997342632669,
0.999997342632669,0.999997342632669,0.999997342632669,0.999997342632669,
0.999997342632669,0.999997342632669,0.999997342632669,0.999997342632669,
0.999997342632669,0.999997342632669,0.999997342632669,0.999997342632669,
0.999997342632669,0.999997342632669,0.999997342632669,0.999997342632669,
0.999997342632669,0.999997342632669,0.999997342632669,0.999997342632669,
0.999997342632669,0.999997342632669,0.999997342632669,0.999997342632669,
0.999997342632669,0.999997342632669,0.999997342632669,0.999997342632669,
0.999997342632669,0.999997342632669,0.999997342632669,0.999997342632669,
0.999997342632669,0.999997342632669,0.999997342632669,0.999997342632669,
0.999997342632669,0.999997342632669,0.999997342632669,0.999997342632669,
0.999997342632669,0.999997342632669,0.999997342632669,0.999997342632669,
0.999997342632669,0.999997342632669,0.999997342632669,0.999997342632669,
0.999997342632669,0.999997342632669,0.999997342632669,0.999997342632669,
0.999997342632669,0.999997342632669,0.999997342632669,0.999997342632669,
0.999997342632669,0.999997342632669,0.999997342632669,0.999997342632669,
0.999997342632669,0.999997342632669,0.999997342632669,0.999997342632669,
0.999997342632669,0.999997342632669,0.999997342632669,0.999997342632669,
0.999997342632669,0.999997342632669,0.999997342632669,0.999997342632669,
0.999997342632669,0.999997342632669,0.999997342632669,0.999997342632669,
0.999997342632669,0.999997342632669,0.999997342632669,0.999997342632669,
0.999997342632669,0.999997342632669,0.999997342632669,0.999997342632669,
0.999997342632669,0.999997342632669,0.999997342632669,0.999997342632669,
0.999997342632669,0.999997342632669,0.999997342632669,0.999997342632669,
0.999997342632669,0.999997342632669,0.999997342632669,0.999997342632669,
0.999997342632669,0.999997342632669,0.999997342632669,0.999997342632669,
0.999997342632669,0.999997342632669,0.999997342632669,0.999997342632669,
0.999997342632669,0.999997342632669,0.999997342632669,0.999997342632669,
0.999997342632669,0.999997342632669,0.999997342632669,0.999997342632669,
0.999997342632669)))
REPRESENTATION_ITEM('')
SURFACE()
);
#62=(
BOUNDED_SURFACE()
B_SPLINE_SURFACE(3,3,((#4678,#4679,#4680,#4681,#4682,#4683,#4684,#4685,
#4686,#4687,#4688,#4689,#4690,#4691,#4692,#4693,#4694,#4695,#4696,#4697,
#4698,#4699,#4700,#4701,#4702,#4703,#4704,#4705,#4706,#4707,#4708,#4709,
#4710,#4711,#4712,#4713,#4714,#4715,#4716,#4717,#4718,#4719,#4720,#4721,
#4722,#4723,#4724,#4725,#4726,#4727,#4728,#4729,#4730,#4731,#4732,#4733,
#4734,#4735,#4736,#4737,#4738,#4739,#4740,#4741,#4742,#4743,#4744,#4745,
#4746,#4747,#4748,#4749,#4750,#4751,#4752,#4753,#4754,#4755,#4756,#4757,
#4758,#4759,#4760,#4761,#4762,#4763,#4764,#4765,#4766,#4767,#4768,#4769,
#4770,#4771,#4772,#4773,#4774,#4775,#4776,#4777,#4778,#4779,#4780,#4781),
(#4782,#4783,#4784,#4785,#4786,#4787,#4788,#4789,#4790,#4791,#4792,#4793,
#4794,#4795,#4796,#4797,#4798,#4799,#4800,#4801,#4802,#4803,#4804,#4805,
#4806,#4807,#4808,#4809,#4810,#4811,#4812,#4813,#4814,#4815,#4816,#4817,
#4818,#4819,#4820,#4821,#4822,#4823,#4824,#4825,#4826,#4827,#4828,#4829,
#4830,#4831,#4832,#4833,#4834,#4835,#4836,#4837,#4838,#4839,#4840,#4841,
#4842,#4843,#4844,#4845,#4846,#4847,#4848,#4849,#4850,#4851,#4852,#4853,
#4854,#4855,#4856,#4857,#4858,#4859,#4860,#4861,#4862,#4863,#4864,#4865,
#4866,#4867,#4868,#4869,#4870,#4871,#4872,#4873,#4874,#4875,#4876,#4877,
#4878,#4879,#4880,#4881,#4882,#4883,#4884,#4885),(#4886,#4887,#4888,#4889,
#4890,#4891,#4892,#4893,#4894,#4895,#4896,#4897,#4898,#4899,#4900,#4901,
#4902,#4903,#4904,#4905,#4906,#4907,#4908,#4909,#4910,#4911,#4912,#4913,
#4914,#4915,#4916,#4917,#4918,#4919,#4920,#4921,#4922,#4923,#4924,#4925,
#4926,#4927,#4928,#4929,#4930,#4931,#4932,#4933,#4934,#4935,#4936,#4937,
#4938,#4939,#4940,#4941,#4942,#4943,#4944,#4945,#4946,#4947,#4948,#4949,
#4950,#4951,#4952,#4953,#4954,#4955,#4956,#4957,#4958,#4959,#4960,#4961,
#4962,#4963,#4964,#4965,#4966,#4967,#4968,#4969,#4970,#4971,#4972,#4973,
#4974,#4975,#4976,#4977,#4978,#4979,#4980,#4981,#4982,#4983,#4984,#4985,
#4986,#4987,#4988,#4989),(#4990,#4991,#4992,#4993,#4994,#4995,#4996,#4997,
#4998,#4999,#5000,#5001,#5002,#5003,#5004,#5005,#5006,#5007,#5008,#5009,
#5010,#5011,#5012,#5013,#5014,#5015,#5016,#5017,#5018,#5019,#5020,#5021,
#5022,#5023,#5024,#5025,#5026,#5027,#5028,#5029,#5030,#5031,#5032,#5033,
#5034,#5035,#5036,#5037,#5038,#5039,#5040,#5041,#5042,#5043,#5044,#5045,
#5046,#5047,#5048,#5049,#5050,#5051,#5052,#5053,#5054,#5055,#5056,#5057,
#5058,#5059,#5060,#5061,#5062,#5063,#5064,#5065,#5066,#5067,#5068,#5069,
#5070,#5071,#5072,#5073,#5074,#5075,#5076,#5077,#5078,#5079,#5080,#5081,
#5082,#5083,#5084,#5085,#5086,#5087,#5088,#5089,#5090,#5091,#5092,#5093),
(#5094,#5095,#5096,#5097,#5098,#5099,#5100,#5101,#5102,#5103,#5104,#5105,
#5106,#5107,#5108,#5109,#5110,#5111,#5112,#5113,#5114,#5115,#5116,#5117,
#5118,#5119,#5120,#5121,#5122,#5123,#5124,#5125,#5126,#5127,#5128,#5129,
#5130,#5131,#5132,#5133,#5134,#5135,#5136,#5137,#5138,#5139,#5140,#5141,
#5142,#5143,#5144,#5145,#5146,#5147,#5148,#5149,#5150,#5151,#5152,#5153,
#5154,#5155,#5156,#5157,#5158,#5159,#5160,#5161,#5162,#5163,#5164,#5165,
#5166,#5167,#5168,#5169,#5170,#5171,#5172,#5173,#5174,#5175,#5176,#5177,
#5178,#5179,#5180,#5181,#5182,#5183,#5184,#5185,#5186,#5187,#5188,#5189,
#5190,#5191,#5192,#5193,#5194,#5195,#5196,#5197),(#5198,#5199,#5200,#5201,
#5202,#5203,#5204,#5205,#5206,#5207,#5208,#5209,#5210,#5211,#5212,#5213,
#5214,#5215,#5216,#5217,#5218,#5219,#5220,#5221,#5222,#5223,#5224,#5225,
#5226,#5227,#5228,#5229,#5230,#5231,#5232,#5233,#5234,#5235,#5236,#5237,
#5238,#5239,#5240,#5241,#5242,#5243,#5244,#5245,#5246,#5247,#5248,#5249,
#5250,#5251,#5252,#5253,#5254,#5255,#5256,#5257,#5258,#5259,#5260,#5261,
#5262,#5263,#5264,#5265,#5266,#5267,#5268,#5269,#5270,#5271,#5272,#5273,
#5274,#5275,#5276,#5277,#5278,#5279,#5280,#5281,#5282,#5283,#5284,#5285,
#5286,#5287,#5288,#5289,#5290,#5291,#5292,#5293,#5294,#5295,#5296,#5297,
#5298,#5299,#5300,#5301),(#5302,#5303,#5304,#5305,#5306,#5307,#5308,#5309,
#5310,#5311,#5312,#5313,#5314,#5315,#5316,#5317,#5318,#5319,#5320,#5321,
#5322,#5323,#5324,#5325,#5326,#5327,#5328,#5329,#5330,#5331,#5332,#5333,
#5334,#5335,#5336,#5337,#5338,#5339,#5340,#5341,#5342,#5343,#5344,#5345,
#5346,#5347,#5348,#5349,#5350,#5351,#5352,#5353,#5354,#5355,#5356,#5357,
#5358,#5359,#5360,#5361,#5362,#5363,#5364,#5365,#5366,#5367,#5368,#5369,
#5370,#5371,#5372,#5373,#5374,#5375,#5376,#5377,#5378,#5379,#5380,#5381,
#5382,#5383,#5384,#5385,#5386,#5387,#5388,#5389,#5390,#5391,#5392,#5393,
#5394,#5395,#5396,#5397,#5398,#5399,#5400,#5401,#5402,#5403,#5404,#5405),
(#5406,#5407,#5408,#5409,#5410,#5411,#5412,#5413,#5414,#5415,#5416,#5417,
#5418,#5419,#5420,#5421,#5422,#5423,#5424,#5425,#5426,#5427,#5428,#5429,
#5430,#5431,#5432,#5433,#5434,#5435,#5436,#5437,#5438,#5439,#5440,#5441,
#5442,#5443,#5444,#5445,#5446,#5447,#5448,#5449,#5450,#5451,#5452,#5453,
#5454,#5455,#5456,#5457,#5458,#5459,#5460,#5461,#5462,#5463,#5464,#5465,
#5466,#5467,#5468,#5469,#5470,#5471,#5472,#5473,#5474,#5475,#5476,#5477,
#5478,#5479,#5480,#5481,#5482,#5483,#5484,#5485,#5486,#5487,#5488,#5489,
#5490,#5491,#5492,#5493,#5494,#5495,#5496,#5497,#5498,#5499,#5500,#5501,
#5502,#5503,#5504,#5505,#5506,#5507,#5508,#5509),(#5510,#5511,#5512,#5513,
#5514,#5515,#5516,#5517,#5518,#5519,#5520,#5521,#5522,#5523,#5524,#5525,
#5526,#5527,#5528,#5529,#5530,#5531,#5532,#5533,#5534,#5535,#5536,#5537,
#5538,#5539,#5540,#5541,#5542,#5543,#5544,#5545,#5546,#5547,#5548,#5549,
#5550,#5551,#5552,#5553,#5554,#5555,#5556,#5557,#5558,#5559,#5560,#5561,
#5562,#5563,#5564,#5565,#5566,#5567,#5568,#5569,#5570,#5571,#5572,#5573,
#5574,#5575,#5576,#5577,#5578,#5579,#5580,#5581,#5582,#5583,#5584,#5585,
#5586,#5587,#5588,#5589,#5590,#5591,#5592,#5593,#5594,#5595,#5596,#5597,
#5598,#5599,#5600,#5601,#5602,#5603,#5604,#5605,#5606,#5607,#5608,#5609,
#5610,#5611,#5612,#5613),(#5614,#5615,#5616,#5617,#5618,#5619,#5620,#5621,
#5622,#5623,#5624,#5625,#5626,#5627,#5628,#5629,#5630,#5631,#5632,#5633,
#5634,#5635,#5636,#5637,#5638,#5639,#5640,#5641,#5642,#5643,#5644,#5645,
#5646,#5647,#5648,#5649,#5650,#5651,#5652,#5653,#5654,#5655,#5656,#5657,
#5658,#5659,#5660,#5661,#5662,#5663,#5664,#5665,#5666,#5667,#5668,#5669,
#5670,#5671,#5672,#5673,#5674,#5675,#5676,#5677,#5678,#5679,#5680,#5681,
#5682,#5683,#5684,#5685,#5686,#5687,#5688,#5689,#5690,#5691,#5692,#5693,
#5694,#5695,#5696,#5697,#5698,#5699,#5700,#5701,#5702,#5703,#5704,#5705,
#5706,#5707,#5708,#5709,#5710,#5711,#5712,#5713,#5714,#5715,#5716,#5717)),
 .UNSPECIFIED.,.T.,.F.,.F.)
B_SPLINE_SURFACE_WITH_KNOTS((4,3,3,4),(4,2,2,2,2,2,2,2,2,2,2,2,2,2,2,2,
2,2,2,2,2,2,2,2,2,2,2,2,2,2,2,2,2,2,2,2,2,2,2,2,2,2,2,2,2,2,2,2,2,2,2,4),
(0.499980401958503,0.5,1.,1.4999804019585),(0.,0.0155213821795324,0.0465641465385971,
0.0776069108976618,0.108649675256726,0.139692439615791,0.170735203974856,
0.201777968333921,0.232820732692985,0.26386349705205,0.294906261411162,
0.325949025770274,0.356991790129291,0.388034554488308,0.419077318847373,
0.450120083206437,0.46564146538597,0.481162847565502,0.496684229745034,
0.512205611924566,0.527726994104099,0.543248376283631,0.558769758463163,
0.574291140642696,0.589812522822228,0.605333905001761,0.620855287181293,
0.636376669360825,0.651898051540357,0.66741943371989,0.682940815899422,
0.698462198078954,0.713983580258487,0.729504962438019,0.745026344617551,
0.760547726797084,0.776069108976616,0.791590491156148,0.807111873335681,
0.822633255515213,0.838154637694745,0.853676019874278,0.86919740205381,
0.884718784233342,0.900240166412875,0.915761548592407,0.931282930771939,
0.946804312951471,0.973402156475736,0.986701078237868,0.993350539118934,
1.),.UNSPECIFIED.)
GEOMETRIC_REPRESENTATION_ITEM()
RATIONAL_B_SPLINE_SURFACE(((0.999921610906677,0.999921610906677,0.999921610906677,
0.999921610906677,0.999921610906677,0.999921610906677,0.999921610906677,
0.999921610906677,0.999921610906677,0.999921610906677,0.999921610906677,
0.999921610906677,0.999921610906677,0.999921610906677,0.999921610906677,
0.999921610906677,0.999921610906677,0.999921610906677,0.999921610906677,
0.999921610906677,0.999921610906677,0.999921610906677,0.999921610906677,
0.999921610906677,0.999921610906677,0.999921610906677,0.999921610906677,
0.999921610906677,0.999921610906677,0.999921610906677,0.999921610906677,
0.999921610906677,0.999921610906677,0.999921610906677,0.999921610906677,
0.999921610906677,0.999921610906677,0.999921610906677,0.999921610906677,
0.999921610906677,0.999921610906677,0.999921610906677,0.999921610906677,
0.999921610906677,0.999921610906677,0.999921610906677,0.999921610906677,
0.999921610906677,0.999921610906677,0.999921610906677,0.999921610906677,
0.999921610906677,0.999921610906677,0.999921610906677,0.999921610906677,
0.999921610906677,0.999921610906677,0.999921610906677,0.999921610906677,
0.999921610906677,0.999921610906677,0.999921610906677,0.999921610906677,
0.999921610906677,0.999921610906677,0.999921610906677,0.999921610906677,
0.999921610906677,0.999921610906677,0.999921610906677,0.999921610906677,
0.999921610906677,0.999921610906677,0.999921610906677,0.999921610906677,
0.999921610906677,0.999921610906677,0.999921610906677,0.999921610906677,
0.999921610906677,0.999921610906677,0.999921610906677,0.999921610906677,
0.999921610906677,0.999921610906677,0.999921610906677,0.999921610906677,
0.999921610906677,0.999921610906677,0.999921610906677,0.999921610906677,
0.999921610906677,0.999921610906677,0.999921610906677,0.999921610906677,
0.999921610906677,0.999921610906677,0.999921610906677,0.999921610906677,
0.999921610906677,0.999921610906677,0.999921610906677,0.999921610906677,
0.999921610906677),(0.999947739580229,0.999947739580229,0.999947739580229,
0.999947739580229,0.999947739580229,0.999947739580229,0.999947739580229,
0.999947739580229,0.999947739580229,0.999947739580229,0.999947739580229,
0.999947739580229,0.999947739580229,0.999947739580229,0.999947739580229,
0.999947739580229,0.999947739580229,0.999947739580229,0.999947739580229,
0.999947739580229,0.999947739580229,0.999947739580229,0.999947739580229,
0.999947739580229,0.999947739580229,0.999947739580229,0.999947739580229,
0.999947739580229,0.999947739580229,0.999947739580229,0.999947739580229,
0.999947739580229,0.999947739580229,0.999947739580229,0.999947739580229,
0.999947739580229,0.999947739580229,0.999947739580229,0.999947739580229,
0.999947739580229,0.999947739580229,0.999947739580229,0.999947739580229,
0.999947739580229,0.999947739580229,0.999947739580229,0.999947739580229,
0.999947739580229,0.999947739580229,0.999947739580229,0.999947739580229,
0.999947739580229,0.999947739580229,0.999947739580229,0.999947739580229,
0.999947739580229,0.999947739580229,0.999947739580229,0.999947739580229,
0.999947739580229,0.999947739580229,0.999947739580229,0.999947739580229,
0.999947739580229,0.999947739580229,0.999947739580229,0.999947739580229,
0.999947739580229,0.999947739580229,0.999947739580229,0.999947739580229,
0.999947739580229,0.999947739580229,0.999947739580229,0.999947739580229,
0.999947739580229,0.999947739580229,0.999947739580229,0.999947739580229,
0.999947739580229,0.999947739580229,0.999947739580229,0.999947739580229,
0.999947739580229,0.999947739580229,0.999947739580229,0.999947739580229,
0.999947739580229,0.999947739580229,0.999947739580229,0.999947739580229,
0.999947739580229,0.999947739580229,0.999947739580229,0.999947739580229,
0.999947739580229,0.999947739580229,0.999947739580229,0.999947739580229,
0.999947739580229,0.999947739580229,0.999947739580229,0.999947739580229,
0.999947739580229),(0.999973869278004,0.999973869278004,0.999973869278004,
0.999973869278004,0.999973869278004,0.999973869278004,0.999973869278004,
0.999973869278004,0.999973869278004,0.999973869278004,0.999973869278004,
0.999973869278004,0.999973869278004,0.999973869278004,0.999973869278004,
0.999973869278004,0.999973869278004,0.999973869278004,0.999973869278004,
0.999973869278004,0.999973869278004,0.999973869278004,0.999973869278004,
0.999973869278004,0.999973869278004,0.999973869278004,0.999973869278004,
0.999973869278004,0.999973869278004,0.999973869278004,0.999973869278004,
0.999973869278004,0.999973869278004,0.999973869278004,0.999973869278004,
0.999973869278004,0.999973869278004,0.999973869278004,0.999973869278004,
0.999973869278004,0.999973869278004,0.999973869278004,0.999973869278004,
0.999973869278004,0.999973869278004,0.999973869278004,0.999973869278004,
0.999973869278004,0.999973869278004,0.999973869278004,0.999973869278004,
0.999973869278004,0.999973869278004,0.999973869278004,0.999973869278004,
0.999973869278004,0.999973869278004,0.999973869278004,0.999973869278004,
0.999973869278004,0.999973869278004,0.999973869278004,0.999973869278004,
0.999973869278004,0.999973869278004,0.999973869278004,0.999973869278004,
0.999973869278004,0.999973869278004,0.999973869278004,0.999973869278004,
0.999973869278004,0.999973869278004,0.999973869278004,0.999973869278004,
0.999973869278004,0.999973869278004,0.999973869278004,0.999973869278004,
0.999973869278004,0.999973869278004,0.999973869278004,0.999973869278004,
0.999973869278004,0.999973869278004,0.999973869278004,0.999973869278004,
0.999973869278004,0.999973869278004,0.999973869278004,0.999973869278004,
0.999973869278004,0.999973869278004,0.999973869278004,0.999973869278004,
0.999973869278004,0.999973869278004,0.999973869278004,0.999973869278004,
0.999973869278004,0.999973869278004,0.999973869278004,0.999973869278004,
0.999973869278004),(1.,1.,1.,1.,1.,1.,1.,1.,1.,1.,1.,1.,1.,1.,1.,1.,1.,
1.,1.,1.,1.,1.,1.,1.,1.,1.,1.,1.,1.,1.,1.,1.,1.,1.,1.,1.,1.,1.,1.,1.,1.,
1.,1.,1.,1.,1.,1.,1.,1.,1.,1.,1.,1.,1.,1.,1.,1.,1.,1.,1.,1.,1.,1.,1.,1.,
1.,1.,1.,1.,1.,1.,1.,1.,1.,1.,1.,1.,1.,1.,1.,1.,1.,1.,1.,1.,1.,1.,1.,1.,
1.,1.,1.,1.,1.,1.,1.,1.,1.,1.,1.,1.,1.,1.,1.),(0.333333333333333,0.333333333333333,
0.333333333333333,0.333333333333333,0.333333333333333,0.333333333333333,
0.333333333333333,0.333333333333333,0.333333333333333,0.333333333333333,
0.333333333333333,0.333333333333333,0.333333333333333,0.333333333333333,
0.333333333333333,0.333333333333333,0.333333333333333,0.333333333333333,
0.333333333333333,0.333333333333333,0.333333333333333,0.333333333333333,
0.333333333333333,0.333333333333333,0.333333333333333,0.333333333333333,
0.333333333333333,0.333333333333333,0.333333333333333,0.333333333333333,
0.333333333333333,0.333333333333333,0.333333333333333,0.333333333333333,
0.333333333333333,0.333333333333333,0.333333333333333,0.333333333333333,
0.333333333333333,0.333333333333333,0.333333333333333,0.333333333333333,
0.333333333333333,0.333333333333333,0.333333333333333,0.333333333333333,
0.333333333333333,0.333333333333333,0.333333333333333,0.333333333333333,
0.333333333333333,0.333333333333333,0.333333333333333,0.333333333333333,
0.333333333333333,0.333333333333333,0.333333333333333,0.333333333333333,
0.333333333333333,0.333333333333333,0.333333333333333,0.333333333333333,
0.333333333333333,0.333333333333333,0.333333333333333,0.333333333333333,
0.333333333333333,0.333333333333333,0.333333333333333,0.333333333333333,
0.333333333333333,0.333333333333333,0.333333333333333,0.333333333333333,
0.333333333333333,0.333333333333333,0.333333333333333,0.333333333333333,
0.333333333333333,0.333333333333333,0.333333333333333,0.333333333333333,
0.333333333333333,0.333333333333333,0.333333333333333,0.333333333333333,
0.333333333333333,0.333333333333333,0.333333333333333,0.333333333333333,
0.333333333333333,0.333333333333333,0.333333333333333,0.333333333333333,
0.333333333333333,0.333333333333333,0.333333333333333,0.333333333333333,
0.333333333333333,0.333333333333333,0.333333333333333,0.333333333333333,
0.333333333333333,0.333333333333333),(0.333333333333333,0.333333333333333,
0.333333333333333,0.333333333333333,0.333333333333333,0.333333333333333,
0.333333333333333,0.333333333333333,0.333333333333333,0.333333333333333,
0.333333333333333,0.333333333333333,0.333333333333333,0.333333333333333,
0.333333333333333,0.333333333333333,0.333333333333333,0.333333333333333,
0.333333333333333,0.333333333333333,0.333333333333333,0.333333333333333,
0.333333333333333,0.333333333333333,0.333333333333333,0.333333333333333,
0.333333333333333,0.333333333333333,0.333333333333333,0.333333333333333,
0.333333333333333,0.333333333333333,0.333333333333333,0.333333333333333,
0.333333333333333,0.333333333333333,0.333333333333333,0.333333333333333,
0.333333333333333,0.333333333333333,0.333333333333333,0.333333333333333,
0.333333333333333,0.333333333333333,0.333333333333333,0.333333333333333,
0.333333333333333,0.333333333333333,0.333333333333333,0.333333333333333,
0.333333333333333,0.333333333333333,0.333333333333333,0.333333333333333,
0.333333333333333,0.333333333333333,0.333333333333333,0.333333333333333,
0.333333333333333,0.333333333333333,0.333333333333333,0.333333333333333,
0.333333333333333,0.333333333333333,0.333333333333333,0.333333333333333,
0.333333333333333,0.333333333333333,0.333333333333333,0.333333333333333,
0.333333333333333,0.333333333333333,0.333333333333333,0.333333333333333,
0.333333333333333,0.333333333333333,0.333333333333333,0.333333333333333,
0.333333333333333,0.333333333333333,0.333333333333333,0.333333333333333,
0.333333333333333,0.333333333333333,0.333333333333333,0.333333333333333,
0.333333333333333,0.333333333333333,0.333333333333333,0.333333333333333,
0.333333333333333,0.333333333333333,0.333333333333333,0.333333333333333,
0.333333333333333,0.333333333333333,0.333333333333333,0.333333333333333,
0.333333333333333,0.333333333333333,0.333333333333333,0.333333333333333,
0.333333333333333,0.333333333333333),(1.,1.,1.,1.,1.,1.,1.,1.,1.,1.,1.,
1.,1.,1.,1.,1.,1.,1.,1.,1.,1.,1.,1.,1.,1.,1.,1.,1.,1.,1.,1.,1.,1.,1.,1.,
1.,1.,1.,1.,1.,1.,1.,1.,1.,1.,1.,1.,1.,1.,1.,1.,1.,1.,1.,1.,1.,1.,1.,1.,
1.,1.,1.,1.,1.,1.,1.,1.,1.,1.,1.,1.,1.,1.,1.,1.,1.,1.,1.,1.,1.,1.,1.,1.,
1.,1.,1.,1.,1.,1.,1.,1.,1.,1.,1.,1.,1.,1.,1.,1.,1.,1.,1.,1.,1.),(0.33335946405533,
0.33335946405533,0.33335946405533,0.33335946405533,0.33335946405533,0.33335946405533,
0.33335946405533,0.33335946405533,0.33335946405533,0.33335946405533,0.33335946405533,
0.33335946405533,0.33335946405533,0.33335946405533,0.33335946405533,0.33335946405533,
0.33335946405533,0.33335946405533,0.33335946405533,0.33335946405533,0.33335946405533,
0.33335946405533,0.33335946405533,0.33335946405533,0.33335946405533,0.33335946405533,
0.33335946405533,0.33335946405533,0.33335946405533,0.33335946405533,0.33335946405533,
0.33335946405533,0.33335946405533,0.33335946405533,0.33335946405533,0.33335946405533,
0.33335946405533,0.33335946405533,0.33335946405533,0.33335946405533,0.33335946405533,
0.33335946405533,0.33335946405533,0.33335946405533,0.33335946405533,0.33335946405533,
0.33335946405533,0.33335946405533,0.33335946405533,0.33335946405533,0.33335946405533,
0.33335946405533,0.33335946405533,0.33335946405533,0.33335946405533,0.33335946405533,
0.33335946405533,0.33335946405533,0.33335946405533,0.33335946405533,0.33335946405533,
0.33335946405533,0.33335946405533,0.33335946405533,0.33335946405533,0.33335946405533,
0.33335946405533,0.33335946405533,0.33335946405533,0.33335946405533,0.33335946405533,
0.33335946405533,0.33335946405533,0.33335946405533,0.33335946405533,0.33335946405533,
0.33335946405533,0.33335946405533,0.33335946405533,0.33335946405533,0.33335946405533,
0.33335946405533,0.33335946405533,0.33335946405533,0.33335946405533,0.33335946405533,
0.33335946405533,0.33335946405533,0.33335946405533,0.33335946405533,0.33335946405533,
0.33335946405533,0.33335946405533,0.33335946405533,0.33335946405533,0.33335946405533,
0.33335946405533,0.33335946405533,0.33335946405533,0.33335946405533,0.33335946405533,
0.33335946405533,0.33335946405533,0.33335946405533),(0.333333334357555,
0.333333334357555,0.333333334357555,0.333333334357555,0.333333334357555,
0.333333334357555,0.333333334357555,0.333333334357555,0.333333334357555,
0.333333334357555,0.333333334357555,0.333333334357555,0.333333334357555,
0.333333334357555,0.333333334357555,0.333333334357555,0.333333334357555,
0.333333334357555,0.333333334357555,0.333333334357555,0.333333334357555,
0.333333334357555,0.333333334357555,0.333333334357555,0.333333334357555,
0.333333334357555,0.333333334357555,0.333333334357555,0.333333334357555,
0.333333334357555,0.333333334357555,0.333333334357555,0.333333334357555,
0.333333334357555,0.333333334357555,0.333333334357555,0.333333334357555,
0.333333334357555,0.333333334357555,0.333333334357555,0.333333334357555,
0.333333334357555,0.333333334357555,0.333333334357555,0.333333334357555,
0.333333334357555,0.333333334357555,0.333333334357555,0.333333334357555,
0.333333334357555,0.333333334357555,0.333333334357555,0.333333334357555,
0.333333334357555,0.333333334357555,0.333333334357555,0.333333334357555,
0.333333334357555,0.333333334357555,0.333333334357555,0.333333334357555,
0.333333334357555,0.333333334357555,0.333333334357555,0.333333334357555,
0.333333334357555,0.333333334357555,0.333333334357555,0.333333334357555,
0.333333334357555,0.333333334357555,0.333333334357555,0.333333334357555,
0.333333334357555,0.333333334357555,0.333333334357555,0.333333334357555,
0.333333334357555,0.333333334357555,0.333333334357555,0.333333334357555,
0.333333334357555,0.333333334357555,0.333333334357555,0.333333334357555,
0.333333334357555,0.333333334357555,0.333333334357555,0.333333334357555,
0.333333334357555,0.333333334357555,0.333333334357555,0.333333334357555,
0.333333334357555,0.333333334357555,0.333333334357555,0.333333334357555,
0.333333334357555,0.333333334357555,0.333333334357555,0.333333334357555,
0.333333334357555,0.333333334357555,0.333333334357555),(0.999921610906677,
0.999921610906677,0.999921610906677,0.999921610906677,0.999921610906677,
0.999921610906677,0.999921610906677,0.999921610906677,0.999921610906677,
0.999921610906677,0.999921610906677,0.999921610906677,0.999921610906677,
0.999921610906677,0.999921610906677,0.999921610906677,0.999921610906677,
0.999921610906677,0.999921610906677,0.999921610906677,0.999921610906677,
0.999921610906677,0.999921610906677,0.999921610906677,0.999921610906677,
0.999921610906677,0.999921610906677,0.999921610906677,0.999921610906677,
0.999921610906677,0.999921610906677,0.999921610906677,0.999921610906677,
0.999921610906677,0.999921610906677,0.999921610906677,0.999921610906677,
0.999921610906677,0.999921610906677,0.999921610906677,0.999921610906677,
0.999921610906677,0.999921610906677,0.999921610906677,0.999921610906677,
0.999921610906677,0.999921610906677,0.999921610906677,0.999921610906677,
0.999921610906677,0.999921610906677,0.999921610906677,0.999921610906677,
0.999921610906677,0.999921610906677,0.999921610906677,0.999921610906677,
0.999921610906677,0.999921610906677,0.999921610906677,0.999921610906677,
0.999921610906677,0.999921610906677,0.999921610906677,0.999921610906677,
0.999921610906677,0.999921610906677,0.999921610906677,0.999921610906677,
0.999921610906677,0.999921610906677,0.999921610906677,0.999921610906677,
0.999921610906677,0.999921610906677,0.999921610906677,0.999921610906677,
0.999921610906677,0.999921610906677,0.999921610906677,0.999921610906677,
0.999921610906677,0.999921610906677,0.999921610906677,0.999921610906677,
0.999921610906677,0.999921610906677,0.999921610906677,0.999921610906677,
0.999921610906677,0.999921610906677,0.999921610906677,0.999921610906677,
0.999921610906677,0.999921610906677,0.999921610906677,0.999921610906677,
0.999921610906677,0.999921610906677,0.999921610906677,0.999921610906677,
0.999921610906677,0.999921610906677,0.999921610906677)))
REPRESENTATION_ITEM('')
SURFACE()
);
#66=SHAPE_REPRESENTATION_RELATIONSHIP('SRR','None',#5977,#73);
#73=ADVANCED_BREP_SHAPE_REPRESENTATION('',(#87),#5937);
#80=STYLED_ITEM('',(#6021),#87);
#87=MANIFOLD_SOLID_BREP('Body1',#927);
#104=PLANE('',#1037);
#105=PLANE('',#1039);
#148=FACE_OUTER_BOUND('',#204,.T.);
#149=FACE_OUTER_BOUND('',#205,.T.);
#150=FACE_OUTER_BOUND('',#206,.T.);
#151=FACE_OUTER_BOUND('',#207,.T.);
#152=FACE_OUTER_BOUND('',#208,.T.);
#153=FACE_OUTER_BOUND('',#209,.T.);
#204=EDGE_LOOP('',(#658,#659,#660,#661,#662));
#205=EDGE_LOOP('',(#663,#664,#665,#666,#667));
#206=EDGE_LOOP('',(#668,#669,#670,#671,#672));
#207=EDGE_LOOP('',(#673,#674));
#208=EDGE_LOOP('',(#675,#676,#677,#678,#679));
#209=EDGE_LOOP('',(#680,#681));
#420=CIRCLE('',#1030,0.5);
#421=CIRCLE('',#1031,0.5);
#422=CIRCLE('',#1032,0.5);
#423=CIRCLE('',#1033,0.5);
#424=CIRCLE('',#1034,0.5);
#425=CIRCLE('',#1035,0.5);
#426=CIRCLE('',#1036,0.5);
#427=CIRCLE('',#1038,0.5);
#452=VERTEX_POINT('',#2151);
#453=VERTEX_POINT('',#2152);
#454=VERTEX_POINT('',#2154);
#455=VERTEX_POINT('',#2309);
#456=VERTEX_POINT('',#2311);
#457=VERTEX_POINT('',#3374);
#458=VERTEX_POINT('',#3375);
#459=VERTEX_POINT('',#3377);
#532=EDGE_CURVE('',#452,#453,#420,.T.);
#533=EDGE_CURVE('',#453,#454,#55,.T.);
#534=EDGE_CURVE('',#454,#455,#421,.T.);
#535=EDGE_CURVE('',#455,#456,#422,.T.);
#536=EDGE_CURVE('',#452,#456,#56,.T.);
#537=EDGE_CURVE('',#457,#458,#423,.T.);
#538=EDGE_CURVE('',#458,#459,#57,.T.);
#539=EDGE_CURVE('',#456,#459,#424,.T.);
#540=EDGE_CURVE('',#457,#455,#58,.T.);
#541=EDGE_CURVE('',#458,#457,#425,.T.);
#542=EDGE_CURVE('',#459,#454,#426,.T.);
#543=EDGE_CURVE('',#453,#452,#427,.T.);
#658=ORIENTED_EDGE('',*,*,#532,.T.);
#659=ORIENTED_EDGE('',*,*,#533,.T.);
#660=ORIENTED_EDGE('',*,*,#534,.T.);
#661=ORIENTED_EDGE('',*,*,#535,.T.);
#662=ORIENTED_EDGE('',*,*,#536,.F.);
#663=ORIENTED_EDGE('',*,*,#537,.T.);
#664=ORIENTED_EDGE('',*,*,#538,.T.);
#665=ORIENTED_EDGE('',*,*,#539,.F.);
#666=ORIENTED_EDGE('',*,*,#535,.F.);
#667=ORIENTED_EDGE('',*,*,#540,.F.);
#668=ORIENTED_EDGE('',*,*,#538,.F.);
#669=ORIENTED_EDGE('',*,*,#541,.T.);
#670=ORIENTED_EDGE('',*,*,#540,.T.);
#671=ORIENTED_EDGE('',*,*,#534,.F.);
#672=ORIENTED_EDGE('',*,*,#542,.F.);
#673=ORIENTED_EDGE('',*,*,#537,.F.);
#674=ORIENTED_EDGE('',*,*,#541,.F.);
#675=ORIENTED_EDGE('',*,*,#533,.F.);
#676=ORIENTED_EDGE('',*,*,#543,.T.);
#677=ORIENTED_EDGE('',*,*,#536,.T.);
#678=ORIENTED_EDGE('',*,*,#539,.T.);
#679=ORIENTED_EDGE('',*,*,#542,.T.);
#680=ORIENTED_EDGE('',*,*,#532,.F.);
#681=ORIENTED_EDGE('',*,*,#543,.F.);
#879=ADVANCED_FACE('',(#148),#59,.T.);
#880=ADVANCED_FACE('',(#149),#60,.T.);
#881=ADVANCED_FACE('',(#150),#61,.T.);
#882=ADVANCED_FACE('',(#151),#104,.F.);
#883=ADVANCED_FACE('',(#152),#62,.T.);
#884=ADVANCED_FACE('',(#153),#105,.F.);
#927=CLOSED_SHELL('',(#879,#880,#881,#882,#883,#884));
#1029=AXIS2_PLACEMENT_3D('',#1422,#1153,#1154);
#1030=AXIS2_PLACEMENT_3D('',#2153,#1155,#1156);
#1031=AXIS2_PLACEMENT_3D('',#2310,#1157,#1158);
#1032=AXIS2_PLACEMENT_3D('',#2312,#1159,#1160);
#1033=AXIS2_PLACEMENT_3D('',#3376,#1161,#1162);
#1034=AXIS2_PLACEMENT_3D('',#3571,#1163,#1164);
#1035=AXIS2_PLACEMENT_3D('',#4675,#1165,#1166);
#1036=AXIS2_PLACEMENT_3D('',#4676,#1167,#1168);
#1037=AXIS2_PLACEMENT_3D('',#4677,#1169,#1170);
#1038=AXIS2_PLACEMENT_3D('',#5718,#1171,#1172);
#1039=AXIS2_PLACEMENT_3D('',#5719,#1173,#1174);
#1153=DIRECTION('axis',(0.,0.,1.));
#1154=DIRECTION('refdir',(1.,0.,0.));
#1155=DIRECTION('center_axis',(-0.0122214764460586,-0.994958909981894,-0.0995359380380735));
#1156=DIRECTION('ref_axis',(2.2423307198858E-17,0.0995433724380481,-0.995033224070262));
#1157=DIRECTION('center_axis',(-0.0122214764459953,0.994958909981895,0.0995359380380777));
#1158=DIRECTION('ref_axis',(-6.9485554107327E-15,-0.0995433724380523,0.995033224070262));
#1159=DIRECTION('center_axis',(-0.0122214764459953,0.994958909981895,0.0995359380380777));
#1160=DIRECTION('ref_axis',(-6.9485554107327E-15,-0.0995433724380523,0.995033224070262));
#1161=DIRECTION('center_axis',(-0.0122214764460684,0.994958909981894,0.0995359380380777));
#1162=DIRECTION('ref_axis',(-1.06054523794617E-17,-0.0995433724380524,0.995033224070262));
#1163=DIRECTION('center_axis',(-0.0122214764459953,0.994958909981895,0.0995359380380777));
#1164=DIRECTION('ref_axis',(-6.9485554107327E-15,-0.0995433724380523,0.995033224070262));
#1165=DIRECTION('center_axis',(-0.0122214764460684,0.994958909981894,0.0995359380380777));
#1166=DIRECTION('ref_axis',(-1.06054523794617E-17,-0.0995433724380524,0.995033224070262));
#1167=DIRECTION('center_axis',(-0.0122214764459953,0.994958909981895,0.0995359380380777));
#1168=DIRECTION('ref_axis',(-6.9485554107327E-15,-0.0995433724380523,0.995033224070262));
#1169=DIRECTION('center_axis',(-0.0122214764460684,0.994958909981894,0.0995359380380777));
#1170=DIRECTION('ref_axis',(-6.86173012619271E-20,-0.0995433724380523,0.995033224070262));
#1171=DIRECTION('center_axis',(-0.0122214764460586,-0.994958909981894,-0.0995359380380735));
#1172=DIRECTION('ref_axis',(2.2423307198858E-17,0.0995433724380481,-0.995033224070262));
#1173=DIRECTION('center_axis',(-0.0122214764460586,-0.994958909981894,-0.0995359380380735));
#1174=DIRECTION('ref_axis',(-8.78275546101855E-20,0.0995433724380481,-0.995033224070262));
#1422=CARTESIAN_POINT('',(0.,0.,0.));
#1423=CARTESIAN_POINT('Ctrl Pts',(-3.5,-27.1131792176833,21.5024833879649));
#1424=CARTESIAN_POINT('Ctrl Pts',(-3.51479119919922,-27.6859453885664,21.4451837185487));
#1425=CARTESIAN_POINT('Ctrl Pts',(-3.3869826954375,-28.2639018202575,21.3878808596267));
#1426=CARTESIAN_POINT('Ctrl Pts',(-2.61104013965461,-29.8091522948055,21.2159741435134));
#1427=CARTESIAN_POINT('Ctrl Pts',(-1.55527081107218,-30.5598658867912,21.1013735009366));
#1428=CARTESIAN_POINT('Ctrl Pts',(0.7596584103706,-30.8465909355752,20.8721694081605));
#1429=CARTESIAN_POINT('Ctrl Pts',(1.98433800521209,-30.3798149635844,20.7575670418755));
#1430=CARTESIAN_POINT('Ctrl Pts',(3.52578602540974,-28.5931135200025,20.5283676296524));
#1431=CARTESIAN_POINT('Ctrl Pts',(3.8208190800791,-27.3005795704328,20.4137635916772));
#1432=CARTESIAN_POINT('Ctrl Pts',(3.18340034511317,-25.0004020130352,20.1845686868986));
#1433=CARTESIAN_POINT('Ctrl Pts',(2.26172892311522,-24.0264166801336,20.0699630275308));
#1434=CARTESIAN_POINT('Ctrl Pts',(-0.0310075805132356,-23.2709470686081,
19.840772464982));
#1435=CARTESIAN_POINT('Ctrl Pts',(-1.36774615552683,-23.4993356660845,19.7261652328664));
#1436=CARTESIAN_POINT('Ctrl Pts',(-3.29044999554861,-25.003443698954,19.4969788547815));
#1437=CARTESIAN_POINT('Ctrl Pts',(-3.84882652597964,-26.255889878113,19.3823700969656));
#1438=CARTESIAN_POINT('Ctrl Pts',(-3.66341653596594,-28.7171925636406,19.1531877526223));
#1439=CARTESIAN_POINT('Ctrl Pts',(-2.92366288113256,-29.8898022514147,19.0385775146034));
#1440=CARTESIAN_POINT('Ctrl Pts',(-0.750050065449063,-31.1155888685023,
18.8093990599493));
#1441=CARTESIAN_POINT('Ctrl Pts',(0.651110587682156,-31.1517796318851,18.6947873857344));
#1442=CARTESIAN_POINT('Ctrl Pts',(2.90172211077653,-30.0124147872479,18.4656126830036));
#1443=CARTESIAN_POINT('Ctrl Pts',(3.71853772096227,-28.8547645355866,18.3509996151738));
#1444=CARTESIAN_POINT('Ctrl Pts',(4.02392234264642,-26.3233804905586,18.1218285325501));
#1445=CARTESIAN_POINT('Ctrl Pts',(3.50918503257104,-24.9871031169595,18.0072141122992));
#1446=CARTESIAN_POINT('Ctrl Pts',(1.55288051607053,-23.3098136929698,17.7780465236243));
#1447=CARTESIAN_POINT('Ctrl Pts',(0.140896517323791,-22.9926200323223,17.6634307908027));
#1448=CARTESIAN_POINT('Ctrl Pts',(-2.36650964254058,-23.6955465860942,17.4342665752667));
#1449=CARTESIAN_POINT('Ctrl Pts',(-3.42532249325332,-24.7042160076948,17.319649568463));
#1450=CARTESIAN_POINT('Ctrl Pts',(-4.24151789226149,-27.205672166438,17.0904886102752));
#1451=CARTESIAN_POINT('Ctrl Pts',(-3.98794903777075,-28.6613021650618,16.9758703668355));
#1452=CARTESIAN_POINT('Ctrl Pts',(-2.34405122024042,-30.7505189403242,16.7467125550671));
#1453=CARTESIAN_POINT('Ctrl Pts',(-0.978754765971974,-31.3540484715026,
16.6320931111307));
#1454=CARTESIAN_POINT('Ctrl Pts',(1.02933886603348,-31.1972354808515,16.460227032321));
#1455=CARTESIAN_POINT('Ctrl Pts',(1.68709482472537,-30.9779968406706,16.4029168679907));
#1456=CARTESIAN_POINT('Ctrl Pts',(2.8240837151474,-30.2508925065775,16.2883402228593));
#1457=CARTESIAN_POINT('Ctrl Pts',(3.30314935266293,-29.7448544918448,16.2310297714992));
#1458=CARTESIAN_POINT('Ctrl Pts',(3.96627580118359,-28.5616040731508,16.116453854622));
#1459=CARTESIAN_POINT('Ctrl Pts',(4.15104388235541,-27.8860791480164,16.0591431204344));
#1460=CARTESIAN_POINT('Ctrl Pts',(4.17802239058402,-26.5231491652539,15.9445679195579));
#1461=CARTESIAN_POINT('Ctrl Pts',(4.02164463287101,-25.836899273559,15.8872569066736));
#1462=CARTESIAN_POINT('Ctrl Pts',(3.39969277305442,-24.6162176795914,15.7726824098211));
#1463=CARTESIAN_POINT('Ctrl Pts',(2.9359020278153,-24.0821430128742,15.7153711223063));
#1464=CARTESIAN_POINT('Ctrl Pts',(1.80627259289743,-23.295059368917,15.6007973177115));
#1465=CARTESIAN_POINT('Ctrl Pts',(1.14217129355625,-23.0415308728188,15.5434857595736));
#1466=CARTESIAN_POINT('Ctrl Pts',(-0.231877317222814,-22.8792861228552,
15.4289126357253));
#1467=CARTESIAN_POINT('Ctrl Pts',(-0.940537550161687,-22.9692999005262,
15.3716008109));
#1468=CARTESIAN_POINT('Ctrl Pts',(-2.23508230276584,-23.4765970744679,15.2570283565139));
#1469=CARTESIAN_POINT('Ctrl Pts',(-2.82042721228882,-23.8921601369938,15.1997162688729));
#1470=CARTESIAN_POINT('Ctrl Pts',(-3.72724254909164,-24.9550994865649,15.0851444728953));
#1471=CARTESIAN_POINT('Ctrl Pts',(-4.04904226418634,-25.6007082903028,15.0278321262568));
#1472=CARTESIAN_POINT('Ctrl Pts',(-4.34898179372202,-26.9722920315092,14.913260977831));
#1473=CARTESIAN_POINT('Ctrl Pts',(-4.32823823833014,-27.696864249156,14.8559483759565));
#1474=CARTESIAN_POINT('Ctrl Pts',(-3.94416673686108,-29.0543767984046,14.741377864454));
#1475=CARTESIAN_POINT('Ctrl Pts',(-3.58247834736109,-29.6866038630478,14.684065011041));
#1476=CARTESIAN_POINT('Ctrl Pts',(-2.59897553580158,-30.7075411869121,14.5694951260371));
#1477=CARTESIAN_POINT('Ctrl Pts',(-1.97893887953295,-31.0963900092535,14.5121820247212));
#1478=CARTESIAN_POINT('Ctrl Pts',(-0.62377058727827,-31.5350735702099,14.3976127560067));
#1479=CARTESIAN_POINT('Ctrl Pts',(0.109859887125028,-31.5858618602476,14.3402994103674));
#1480=CARTESIAN_POINT('Ctrl Pts',(1.51846868411767,-31.3325375520331,14.2257307479178));
#1481=CARTESIAN_POINT('Ctrl Pts',(2.19257064211805,-31.0299670824768,14.1684171614822));
#1482=CARTESIAN_POINT('Ctrl Pts',(3.32065975230898,-30.1381775844584,14.0538490954731));
#1483=CARTESIAN_POINT('Ctrl Pts',(3.77459621319051,-29.5507269915758,13.9965352717156));
#1484=CARTESIAN_POINT('Ctrl Pts',(4.35164549000208,-28.2261503388289,13.8819677925012));
#1485=CARTESIAN_POINT('Ctrl Pts',(4.47554085920862,-27.4906059318028,13.8246537348364));
#1486=CARTESIAN_POINT('Ctrl Pts',(4.35932633846837,-26.043646007592,13.7100868329779));
#1487=CARTESIAN_POINT('Ctrl Pts',(4.1206457473642,-25.3332578752253,13.6527725447744));
#1488=CARTESIAN_POINT('Ctrl Pts',(3.33223129728641,-24.106308328171,13.5382062109767));
#1489=CARTESIAN_POINT('Ctrl Pts',(2.78423731477771,-23.5899834651597,13.4808916955503));
#1490=CARTESIAN_POINT('Ctrl Pts',(1.50450674316234,-22.8764080003258,13.3663259207328));
#1491=CARTESIAN_POINT('Ctrl Pts',(0.774413779611081,-22.6785518889991,13.309011181339));
#1492=CARTESIAN_POINT('Ctrl Pts',(-0.69739330426496,-22.6525522223851,13.1944459565731));
#1493=CARTESIAN_POINT('Ctrl Pts',(-1.43794247925327,-22.8231062186778,13.1371309964266));
#1494=CARTESIAN_POINT('Ctrl Pts',(-2.7541948376007,-23.4972409646481,13.0225663129528));
#1495=CARTESIAN_POINT('Ctrl Pts',(-3.32948087019843,-23.9991290609593,12.9652511352145));
#1496=CARTESIAN_POINT('Ctrl Pts',(-4.17626345911414,-25.2198325829076,12.8506869844455));
#1497=CARTESIAN_POINT('Ctrl Pts',(-4.4481843446811,-25.936961310921,12.7933715922294));
#1498=CARTESIAN_POINT('Ctrl Pts',(-4.62015665278908,-27.4194785452993,12.6788079657272));
#1499=CARTESIAN_POINT('Ctrl Pts',(-4.52137115313415,-28.183579240772,12.621492362104));
#1500=CARTESIAN_POINT('Ctrl Pts',(-3.97152663554103,-29.5783806208201,12.5069292515898));
#1501=CARTESIAN_POINT('Ctrl Pts',(-3.5220951227733,-30.2084906103522,12.4496134395774));
#1502=CARTESIAN_POINT('Ctrl Pts',(-2.37437165907619,-31.183679244984,12.3350508369351));
#1503=CARTESIAN_POINT('Ctrl Pts',(-1.67779038310627,-31.5289988293348,12.277734819509));
#1504=CARTESIAN_POINT('Ctrl Pts',(-0.199197333900588,-31.8492812709321,
12.1631727167557));
#1505=CARTESIAN_POINT('Ctrl Pts',(0.581419535730091,-31.825256919753,12.1058564968451));
#1506=CARTESIAN_POINT('Ctrl Pts',(2.04290487097247,-31.4086885823989,11.9912948861633));
#1507=CARTESIAN_POINT('Ctrl Pts',(2.72301785637377,-31.017689933097,11.9339784666505));
#1508=CARTESIAN_POINT('Ctrl Pts',(3.82034316796606,-29.9565159886648,11.8194173403514));
#1509=CARTESIAN_POINT('Ctrl Pts',(4.23761275995296,-29.2880562452814,11.7621007240815));
#1510=CARTESIAN_POINT('Ctrl Pts',(4.70706068115205,-27.8283747226536,11.6475400746183));
#1511=CARTESIAN_POINT('Ctrl Pts',(4.76009229327592,-27.0386382546772,11.5902232643864));
#1512=CARTESIAN_POINT('Ctrl Pts',(4.48463927434238,-25.5233462828554,11.4756630843606));
#1513=CARTESIAN_POINT('Ctrl Pts',(4.15760185288866,-24.7987006850272,11.4183460829245));
#1514=CARTESIAN_POINT('Ctrl Pts',(3.19600835697949,-23.5869462478655,11.3037863650511));
#1515=CARTESIAN_POINT('Ctrl Pts',(2.56315379146772,-23.099962191222,11.2464691751292));
#1516=CARTESIAN_POINT('Ctrl Pts',(1.13757263913847,-22.4820219779078,11.1319099122695));
#1517=CARTESIAN_POINT('Ctrl Pts',(0.346404347142174,-22.3503795041057,11.0745925365344));
#1518=CARTESIAN_POINT('Ctrl Pts',(-1.76387591167285,-22.5237230755283,10.9191576492385));
#1519=CARTESIAN_POINT('Ctrl Pts',(-3.04213419140331,-23.2249589278969,10.8209586709532));
#1520=CARTESIAN_POINT('Ctrl Pts',(-4.26287386638314,-24.8351878142477,10.6736877485838));
#1521=CARTESIAN_POINT('Ctrl Pts',(-4.55417709738229,-25.4602183705301,10.6246080237907));
#1522=CARTESIAN_POINT('Ctrl Pts',(-4.78298015330037,-26.4482305165422,10.5509677380958));
#1523=CARTESIAN_POINT('Ctrl Pts',(-4.82497450026767,-26.7858033043513,10.5264227857054));
#1524=CARTESIAN_POINT('Ctrl Pts',(-4.83612470074125,-27.4630368812996,10.4773448839533));
#1525=CARTESIAN_POINT('Ctrl Pts',(-4.81152195248019,-27.8040996825675,10.4527957512917));
#1526=CARTESIAN_POINT('Ctrl Pts',(-4.7966595069499,-28.1445096413087,10.4282516293878));
#1527=CARTESIAN_POINT('Ctrl Pts',(-2.50007468503219,-27.1253399927944,21.5012668209833));
#1528=CARTESIAN_POINT('Ctrl Pts',(-2.51283639211379,-27.5313396040275,21.4450628827391));
#1529=CARTESIAN_POINT('Ctrl Pts',(-2.42258993385229,-27.9512582892639,21.3862340567569));
#1530=CARTESIAN_POINT('Ctrl Pts',(-1.87705908045303,-29.0525304994187,21.2178402639005));
#1531=CARTESIAN_POINT('Ctrl Pts',(-1.11370965992309,-29.6026650811217,21.1000517830227));
#1532=CARTESIAN_POINT('Ctrl Pts',(0.538323541218874,-29.815954615602,20.8754777398045));
#1533=CARTESIAN_POINT('Ctrl Pts',(1.43377361752959,-29.4808752026413,20.7577246144251));
#1534=CARTESIAN_POINT('Ctrl Pts',(2.54587760682549,-28.2045638431909,20.5331025971331));
#1535=CARTESIAN_POINT('Ctrl Pts',(2.76750114097136,-27.2589325509883,20.4153840366144));
#1536=CARTESIAN_POINT('Ctrl Pts',(2.31593508025811,-25.5993026196536,20.1907150274047));
#1537=CARTESIAN_POINT('Ctrl Pts',(1.6419110691535,-24.8790793164352,20.0730302677181));
#1538=CARTESIAN_POINT('Ctrl Pts',(-0.0149683894611636,-24.3249408654976,
19.8483152194252));
#1539=CARTESIAN_POINT('Ctrl Pts',(-1.00313453278291,-24.4884039772537,19.7306635219149));
#1540=CARTESIAN_POINT('Ctrl Pts',(-2.4051781686742,-25.5756604965874,19.5059033598245));
#1541=CARTESIAN_POINT('Ctrl Pts',(-2.82388459307759,-26.5022176830049,19.3882840101185));
#1542=CARTESIAN_POINT('Ctrl Pts',(-2.69582100380578,-28.2990165041629,19.1634796322399));
#1543=CARTESIAN_POINT('Ctrl Pts',(-2.14943180799116,-29.1744485529642,19.0458919391655));
#1544=CARTESIAN_POINT('Ctrl Pts',(-0.560198814082305,-30.0787479984767,
18.8210442180266));
#1545=CARTESIAN_POINT('Ctrl Pts',(0.486450458466467,-30.1106125532363,18.7034875125573));
#1546=CARTESIAN_POINT('Ctrl Pts',(2.14509782251475,-29.2785424876867,18.478597295444));
#1547=CARTESIAN_POINT('Ctrl Pts',(2.76136687700576,-28.4132455801264,18.3610709299044));
#1548=CARTESIAN_POINT('Ctrl Pts',(2.99339233231008,-26.5447839295675,18.1361390401663));
#1549=CARTESIAN_POINT('Ctrl Pts',(2.61031700332953,-25.5376669816206,18.0186423872216));
#1550=CARTESIAN_POINT('Ctrl Pts',(1.16446086543928,-24.2896610973114,17.7936696249626));
#1551=CARTESIAN_POINT('Ctrl Pts',(0.09930017734222,-24.0458624466996,17.6762020766647));
#1552=CARTESIAN_POINT('Ctrl Pts',(-1.7675888393034,-24.5628529769143,17.4511892199568));
#1553=CARTESIAN_POINT('Ctrl Pts',(-2.57270112799042,-25.3239325128253,17.333750187231));
#1554=CARTESIAN_POINT('Ctrl Pts',(-3.18765925209663,-27.1895201174977,17.1086979919401));
#1555=CARTESIAN_POINT('Ctrl Pts',(-2.99900529386622,-28.296664824665,16.991286903718));
#1556=CARTESIAN_POINT('Ctrl Pts',(-1.77201713798893,-29.8653042054102,16.7661961054407));
#1557=CARTESIAN_POINT('Ctrl Pts',(-0.732529681096322,-30.3292078520877,
16.6488124076455));
#1558=CARTESIAN_POINT('Ctrl Pts',(0.777221611436293,-30.2154776693097,16.4799658932922));
#1559=CARTESIAN_POINT('Ctrl Pts',(1.28140778933044,-30.049082741554,16.4212841687898));
#1560=CARTESIAN_POINT('Ctrl Pts',(2.13894102609193,-29.5039217906006,16.3087104851517));
#1561=CARTESIAN_POINT('Ctrl Pts',(2.50748319588252,-29.1168780348298,16.2500354076075));
#1562=CARTESIAN_POINT('Ctrl Pts',(3.00992376655387,-28.2258212672248,16.1374524690789));
#1563=CARTESIAN_POINT('Ctrl Pts',(3.15331377168557,-27.7073372554579,16.0787839738266));
#1564=CARTESIAN_POINT('Ctrl Pts',(3.17632285443344,-26.6778431099855,15.9661918649761));
#1565=CARTESIAN_POINT('Ctrl Pts',(3.05748130255417,-26.1495930224966,15.9075298882322));
#1566=CARTESIAN_POINT('Ctrl Pts',(2.58921125566468,-25.2248424296844,15.7949286927493));
#1567=CARTESIAN_POINT('Ctrl Pts',(2.2330033354922,-24.8124137254194,15.7362731716848));
#1568=CARTESIAN_POINT('Ctrl Pts',(1.37840967612313,-24.2138679666298,15.6236629718413));
#1569=CARTESIAN_POINT('Ctrl Pts',(0.866528503509928,-24.0169055865723,15.5650138445848));
#1570=CARTESIAN_POINT('Ctrl Pts',(-0.176086822448727,-23.8912812923305,
15.4523947217693));
#1571=CARTESIAN_POINT('Ctrl Pts',(-0.723839333138843,-23.9594255922406,
15.3937519273021));
#1572=CARTESIAN_POINT('Ctrl Pts',(-1.70882778077597,-24.342780211676,15.2811239616996));
#1573=CARTESIAN_POINT('Ctrl Pts',(-2.16257723397831,-24.6632061601177,15.2224874398782));
#1574=CARTESIAN_POINT('Ctrl Pts',(-2.85481959844414,-25.4709142401168,15.1098507107457));
#1575=CARTESIAN_POINT('Ctrl Pts',(-3.10541208162622,-25.9705887465318,15.0512204022701));
#1576=CARTESIAN_POINT('Ctrl Pts',(-3.33643491243401,-27.0159322908697,14.9385749877282));
#1577=CARTESIAN_POINT('Ctrl Pts',(-3.3216858471879,-27.578238681535,14.8799508342142));
#1578=CARTESIAN_POINT('Ctrl Pts',(-3.03062657946405,-28.6155506117409,14.7672968113139));
#1579=CARTESIAN_POINT('Ctrl Pts',(-2.75071538543883,-29.1075013221103,14.7086787551844));
#1580=CARTESIAN_POINT('Ctrl Pts',(-2.00018375681689,-29.8898980947296,14.5960162000601));
#1581=CARTESIAN_POINT('Ctrl Pts',(-1.51839135128136,-30.1935863948407,14.5374041844901));
#1582=CARTESIAN_POINT('Ctrl Pts',(-0.481129998089667,-30.5317228493949,
14.4247331723202));
#1583=CARTESIAN_POINT('Ctrl Pts',(0.0904391347614876,-30.5725753124629,
14.3661271413499));
#1584=CARTESIAN_POINT('Ctrl Pts',(1.17128619067979,-30.3804399078241,14.2534477461713));
#1585=CARTESIAN_POINT('Ctrl Pts',(1.69778284783799,-30.1455013508672,14.1948476446037));
#1586=CARTESIAN_POINT('Ctrl Pts',(2.56566196202055,-29.4621820446215,14.0821599397072));
#1587=CARTESIAN_POINT('Ctrl Pts',(2.9213066794093,-29.0039557713287,14.0235657131016));
#1588=CARTESIAN_POINT('Ctrl Pts',(3.36714885804308,-27.9858932409967,13.9108697706508));
#1589=CARTESIAN_POINT('Ctrl Pts',(3.46527617925812,-27.4106453730656,13.8522813653494));
#1590=CARTESIAN_POINT('Ctrl Pts',(3.37784082869232,-26.295852639153,13.7395772567127));
#1591=CARTESIAN_POINT('Ctrl Pts',(3.19199787774012,-25.7389764859617,13.6809946198038));
#1592=CARTESIAN_POINT('Ctrl Pts',(2.58554795284393,-24.7913997988873,13.5682824152982));
#1593=CARTESIAN_POINT('Ctrl Pts',(2.15651559470711,-24.3855495363483,13.5097054945602));
#1594=CARTESIAN_POINT('Ctrl Pts',(1.16895684306617,-23.832575565039,13.3969852638233));
#1595=CARTESIAN_POINT('Ctrl Pts',(0.595852596233928,-23.6760691824297,13.3384140077367));
#1596=CARTESIAN_POINT('Ctrl Pts',(-0.542579588650037,-23.6539742782162,
13.225685819334));
#1597=CARTESIAN_POINT('Ctrl Pts',(-1.1251889792854,-23.7869913050767,13.1671201771495));
#1598=CARTESIAN_POINT('Ctrl Pts',(-2.14559645901048,-24.3074163661573,13.054384098833));
#1599=CARTESIAN_POINT('Ctrl Pts',(-2.59929053184396,-24.7017492310162,12.9958240204473));
#1600=CARTESIAN_POINT('Ctrl Pts',(-3.25762576760017,-25.647434253134,12.8830801191498));
#1601=CARTESIAN_POINT('Ctrl Pts',(-3.47301577972443,-26.2123929560692,12.824525555112));
#1602=CARTESIAN_POINT('Ctrl Pts',(-3.60843998708556,-27.363536579556,12.7117738969421));
#1603=CARTESIAN_POINT('Ctrl Pts',(-3.53153182161548,-27.9667909104199,12.6532247984982));
#1604=CARTESIAN_POINT('Ctrl Pts',(-3.10566528390168,-29.0521245514136,12.5404654486599));
#1605=CARTESIAN_POINT('Ctrl Pts',(-2.75134896750393,-29.5506975660807,12.4819217677002));
#1606=CARTESIAN_POINT('Ctrl Pts',(-1.85884518892285,-30.3114094990717,12.369154790682));
#1607=CARTESIAN_POINT('Ctrl Pts',(-1.30815106795505,-30.5855637052752,12.3106164797331));
#1608=CARTESIAN_POINT('Ctrl Pts',(-0.155741001580881,-30.8370096520725,
12.1978419391373));
#1609=CARTESIAN_POINT('Ctrl Pts',(0.462671842753837,-30.8189948910673,12.1393089513662));
#1610=CARTESIAN_POINT('Ctrl Pts',(1.60404657876531,-30.4954824535707,12.0265269100757));
#1611=CARTESIAN_POINT('Ctrl Pts',(2.14394545222966,-30.1862453058223,11.9679991992472));
#1612=CARTESIAN_POINT('Ctrl Pts',(3.0028316585045,-29.3580377153228,11.8552097193461));
#1613=CARTESIAN_POINT('Ctrl Pts',(3.33498881469216,-28.8277788561896,11.7966872398373));
#1614=CARTESIAN_POINT('Ctrl Pts',(3.70397767040327,-27.685950722295,11.6838903826651));
#1615=CARTESIAN_POINT('Ctrl Pts',(3.74709584473805,-27.0582142459975,11.6253730894484));
#1616=CARTESIAN_POINT('Ctrl Pts',(3.5328841786163,-25.8705936164613,11.5125689155825));
#1617=CARTESIAN_POINT('Ctrl Pts',(3.2734696560962,-25.2934880851587,11.4540567642246));
#1618=CARTESIAN_POINT('Ctrl Pts',(2.520349254524,-24.3418377285451,11.3412453335038));
#1619=CARTESIAN_POINT('Ctrl Pts',(2.01668017794548,-23.9530915623133,11.2827382801346));
#1620=CARTESIAN_POINT('Ctrl Pts',(0.897564453532843,-23.4662627472373,11.1699196516999));
#1621=CARTESIAN_POINT('Ctrl Pts',(0.266632689637674,-23.3603587008251,11.111417653014));
#1622=CARTESIAN_POINT('Ctrl Pts',(-1.39308043271686,-23.4945707094314,10.9583341865454));
#1623=CARTESIAN_POINT('Ctrl Pts',(-2.41051507768367,-24.0480090686017,10.8592926132578));
#1624=CARTESIAN_POINT('Ctrl Pts',(-3.38001927688757,-25.3235976874956,10.712152032226));
#1625=CARTESIAN_POINT('Ctrl Pts',(-3.61034539690739,-25.8164734424502,10.6637184246244));
#1626=CARTESIAN_POINT('Ctrl Pts',(-3.7931173904721,-26.6014371673577,10.589901366163));
#1627=CARTESIAN_POINT('Ctrl Pts',(-3.82668517274698,-26.8694485711687,10.565370259987));
#1628=CARTESIAN_POINT('Ctrl Pts',(-3.83611228951587,-27.4039358312353,10.517059613737));
#1629=CARTESIAN_POINT('Ctrl Pts',(-3.81313732847822,-27.7633656624966,10.4924048684869));
#1630=CARTESIAN_POINT('Ctrl Pts',(-3.79827488294779,-28.1037756212366,10.4678607465822));
#1631=CARTESIAN_POINT('Ctrl Pts',(-2.50007468503219,-27.2248833652324,22.4963000450535));
#1632=CARTESIAN_POINT('Ctrl Pts',(-2.4973230516022,-27.6307229864326,22.4401121123047));
#1633=CARTESIAN_POINT('Ctrl Pts',(-2.3900690404148,-28.0461795533903,22.3813056708375));
#1634=CARTESIAN_POINT('Ctrl Pts',(-1.80410662012797,-29.1255019961691,22.2129753102057));
#1635=CARTESIAN_POINT('Ctrl Pts',(-1.01989116822409,-29.6445438741314,22.0952214478198));
#1636=CARTESIAN_POINT('Ctrl Pts',(0.638667716265594,-29.7975756887231,21.8707222568133));
#1637=CARTESIAN_POINT('Ctrl Pts',(1.52050852311385,-29.42808298243,21.7530071973406));
#1638=CARTESIAN_POINT('Ctrl Pts',(2.58730699957112,-28.1125682867517,21.5284506711618));
#1639=CARTESIAN_POINT('Ctrl Pts',(2.77328137790538,-27.1587131575376,21.4107735199278));
#1640=CARTESIAN_POINT('Ctrl Pts',(2.26433740680624,-25.5138475614163,21.1861609869398));
#1641=CARTESIAN_POINT('Ctrl Pts',(1.56360921374272,-24.8180370750652,21.0685208793189));
#1642=CARTESIAN_POINT('Ctrl Pts',(-0.113585913522054,-24.3188787500937,
20.8438536227986));
#1643=CARTESIAN_POINT('Ctrl Pts',(-1.09686428893776,-24.5178009465808,20.7262497228448));
#1644=CARTESIAN_POINT('Ctrl Pts',(-2.46563320123022,-25.6525768382252,20.5015289835988));
#1645=CARTESIAN_POINT('Ctrl Pts',(-2.85270548558921,-26.5950753813576,20.3839604828611));
#1646=CARTESIAN_POINT('Ctrl Pts',(-2.66720295546915,-28.3916002393823,20.1591874603215));
#1647=CARTESIAN_POINT('Ctrl Pts',(-2.09003931759816,-29.2502156366228,20.0416535766241));
#1648=CARTESIAN_POINT('Ctrl Pts',(-0.468609715717802,-30.1076026169081,
19.8168294314625));
#1649=CARTESIAN_POINT('Ctrl Pts',(0.581641933078928,-30.1049235048463,19.6993294077519));
#1650=CARTESIAN_POINT('Ctrl Pts',(2.22027058723989,-29.2201403231244,19.4744552627731));
#1651=CARTESIAN_POINT('Ctrl Pts',(2.81040201556557,-28.3324660884538,19.3569883662253));
#1652=CARTESIAN_POINT('Ctrl Pts',(2.98817347828617,-26.4505240261162,19.1320653083975));
#1653=CARTESIAN_POINT('Ctrl Pts',(2.57213067357672,-25.4521246224307,19.0146308292871));
#1654=CARTESIAN_POINT('Ctrl Pts',(1.08461238202261,-24.2407098526991,18.7896599110507));
#1655=CARTESIAN_POINT('Ctrl Pts',(0.00799178041480618,-24.0287177017401,
18.6722571617048));
#1656=CARTESIAN_POINT('Ctrl Pts',(-1.85263633527269,-24.6003741985188,18.4472394027778));
#1657=CARTESIAN_POINT('Ctrl Pts',(-2.63825121549225,-25.388732377058,18.3298677169699));
#1658=CARTESIAN_POINT('Ctrl Pts',(-3.205081356731,-27.2801569719116,18.1048041047243));
#1659=CARTESIAN_POINT('Ctrl Pts',(-2.9831649376875,-28.3867672345334,17.9874628367108));
#1660=CARTESIAN_POINT('Ctrl Pts',(-1.70783979269738,-29.9307710004345,17.7623543286427));
#1661=CARTESIAN_POINT('Ctrl Pts',(-0.650024237860058,-30.3672113434981,
17.6450428520577));
#1662=CARTESIAN_POINT('Ctrl Pts',(0.865186630000211,-30.2134208155298,17.4761784953134));
#1663=CARTESIAN_POINT('Ctrl Pts',(1.36725623215089,-30.0318398410671,17.4175337661475));
#1664=CARTESIAN_POINT('Ctrl Pts',(2.21566236248619,-29.4614040789813,17.304946706094));
#1665=CARTESIAN_POINT('Ctrl Pts',(2.57530571424416,-29.0619405854776,17.2463091979379));
#1666=CARTESIAN_POINT('Ctrl Pts',(3.05800073394719,-28.1527721613655,17.1337114265062));
#1667=CARTESIAN_POINT('Ctrl Pts',(3.1877871455815,-27.6274487856325,17.0750810662931));
#1668=CARTESIAN_POINT('Ctrl Pts',(3.18497727452253,-26.5910785688795,16.9624726925251));
#1669=CARTESIAN_POINT('Ctrl Pts',(3.05096295225393,-26.0630919115944,16.9038494082137));
#1670=CARTESIAN_POINT('Ctrl Pts',(2.55669827095366,-25.144200958879,16.7912305397785));
#1671=CARTESIAN_POINT('Ctrl Pts',(2.18722058458361,-24.7390313387568,16.732614260404));
#1672=CARTESIAN_POINT('Ctrl Pts',(1.31236252412446,-24.1576827525991,16.6199850030865));
#1673=CARTESIAN_POINT('Ctrl Pts',(0.792130109930538,-23.9732737150518,16.561375658774));
#1674=CARTESIAN_POINT('Ctrl Pts',(-0.260444433079681,-23.8722198598602,
16.4487361169824));
#1675=CARTESIAN_POINT('Ctrl Pts',(-0.809754840681111,-23.9553140876739,
16.3901336388362));
#1676=CARTESIAN_POINT('Ctrl Pts',(-1.79218414638217,-24.3649938942232,16.2774839153377));
#1677=CARTESIAN_POINT('Ctrl Pts',(-2.24038399479556,-24.6993401595432,16.2188882354581));
#1678=CARTESIAN_POINT('Ctrl Pts',(-2.91818815440847,-25.529137615882,16.1062284316294));
#1679=CARTESIAN_POINT('Ctrl Pts',(-3.15743206857856,-26.0385320297141,16.0476394830881));
#1680=CARTESIAN_POINT('Ctrl Pts',(-3.3654714364124,-27.0967271438523,15.9349696987346));
#1681=CARTESIAN_POINT('Ctrl Pts',(-3.33619825815045,-27.662358669908,15.8763874156349));
#1682=CARTESIAN_POINT('Ctrl Pts',(-3.01887060851525,-28.7004015301552,15.7637077490722));
#1683=CARTESIAN_POINT('Ctrl Pts',(-2.72459263582721,-29.188559158675,15.7051320664418));
#1684=CARTESIAN_POINT('Ctrl Pts',(-1.9504930567998,-29.9594480905514,15.5924426146465));
#1685=CARTESIAN_POINT('Ctrl Pts',(-1.45776997299186,-30.2531292770361,15.5338734683806));
#1686=CARTESIAN_POINT('Ctrl Pts',(-0.404990234426755,-30.5701818753113,
15.4211743269738));
#1687=CARTESIAN_POINT('Ctrl Pts',(0.171595902055322,-30.5971301657918,15.3626116539469));
#1688=CARTESIAN_POINT('Ctrl Pts',(1.25641083541538,-30.379164019775,15.2499029170041));
#1689=CARTESIAN_POINT('Ctrl Pts',(1.78089508984846,-30.1296184738905,15.1913466549704));
#1690=CARTESIAN_POINT('Ctrl Pts',(2.64032744040503,-29.4216132578738,15.07862841543));
#1691=CARTESIAN_POINT('Ctrl Pts',(2.98742402928102,-28.951416043259,15.0200785030053));
#1692=CARTESIAN_POINT('Ctrl Pts',(3.41436537442326,-27.9154253975122,14.9073508523134));
#1693=CARTESIAN_POINT('Ctrl Pts',(3.49939161592954,-27.3335641004151,14.8488072290052));
#1694=CARTESIAN_POINT('Ctrl Pts',(3.38693299773095,-26.2116611333541,14.7360702574282));
#1695=CARTESIAN_POINT('Ctrl Pts',(3.18644882156979,-25.6550153663941,14.6775328635923));
#1696=CARTESIAN_POINT('Ctrl Pts',(2.5545653302512,-24.712735350079,14.5647866600073));
#1697=CARTESIAN_POINT('Ctrl Pts',(2.11270270631046,-24.3138769369602,14.5062554367953));
#1698=CARTESIAN_POINT('Ctrl Pts',(1.10509122951777,-23.7773695884842,14.3935000890219));
#1699=CARTESIAN_POINT('Ctrl Pts',(0.523891228402976,-23.6329909911365,14.3349749783932));
#1700=CARTESIAN_POINT('Ctrl Pts',(-0.624659171511437,-23.6347573525544,
14.2222105728532));
#1701=CARTESIAN_POINT('Ctrl Pts',(-1.20879903018357,-23.7822465505066,14.1636915176313));
#1702=CARTESIAN_POINT('Ctrl Pts',(-2.22710672018521,-24.328477425712,14.0509181395924));
#1703=CARTESIAN_POINT('Ctrl Pts',(-2.67544143431689,-24.7363107813614,13.99240508335));
#1704=CARTESIAN_POINT('Ctrl Pts',(-3.31996060297977,-25.7038637739138,13.879622816927));
#1705=CARTESIAN_POINT('Ctrl Pts',(-3.52435156498093,-26.2782694012189,13.821115703984));
#1706=CARTESIAN_POINT('Ctrl Pts',(-3.63741165163986,-27.4423671822191,13.7083246321569));
#1707=CARTESIAN_POINT('Ctrl Pts',(-3.54639862955187,-28.0488697379073,13.6498234076231));
#1708=CARTESIAN_POINT('Ctrl Pts',(-3.09472995624812,-29.1353049846404,13.5370236121474));
#1709=CARTESIAN_POINT('Ctrl Pts',(-2.72643785221591,-29.6302056579101,13.4785282218764));
#1710=CARTESIAN_POINT('Ctrl Pts',(-1.81058044300674,-30.3799313917062,13.3657197834808));
#1711=CARTESIAN_POINT('Ctrl Pts',(-1.24923466426418,-30.6443543382562,13.3072301740502));
#1712=CARTESIAN_POINT('Ctrl Pts',(-0.0812416818551773,-30.8752452508522,
13.1944131722907));
#1713=CARTESIAN_POINT('Ctrl Pts',(0.542072912261212,-30.8436839153864,13.1359292910085));
#1714=CARTESIAN_POINT('Ctrl Pts',(1.68771332512077,-30.4947449192179,13.0231038044166));
#1715=CARTESIAN_POINT('Ctrl Pts',(2.22565936133885,-30.1712550743319,12.9646255992779));
#1716=CARTESIAN_POINT('Ctrl Pts',(3.07652976944644,-29.3185537876298,12.8517917053114));
#1717=CARTESIAN_POINT('Ctrl Pts',(3.40034470317039,-28.7765983337464,12.7933191250111));
#1718=CARTESIAN_POINT('Ctrl Pts',(3.75087283940905,-27.6167979591164,12.6804769000917));
#1719=CARTESIAN_POINT('Ctrl Pts',(3.78118424110462,-26.9825905474799,12.6220098940059));
#1720=CARTESIAN_POINT('Ctrl Pts',(3.54228501118274,-25.7876184262315,12.5091594135308));
#1721=CARTESIAN_POINT('Ctrl Pts',(3.26854034758218,-25.2107358862553,12.4506979317093));
#1722=CARTESIAN_POINT('Ctrl Pts',(2.49014343782273,-24.2640304588299,12.337839270068));
#1723=CARTESIAN_POINT('Ctrl Pts',(1.97390393644558,-23.8821352485647,12.2793832632066));
#1724=CARTESIAN_POINT('Ctrl Pts',(0.834695096751776,-23.4114174957062,12.1665164938306));
#1725=CARTESIAN_POINT('Ctrl Pts',(0.195826419298673,-23.3174103743359,12.108065913277));
#1726=CARTESIAN_POINT('Ctrl Pts',(-1.47788831221255,-23.4836403788777,11.9549159128501));
#1727=CARTESIAN_POINT('Ctrl Pts',(-2.49444407803175,-24.0624268927996,11.8559193209146));
#1728=CARTESIAN_POINT('Ctrl Pts',(-3.44927812351996,-25.3687964002138,11.7087911217838));
#1729=CARTESIAN_POINT('Ctrl Pts',(-3.67294914345905,-25.8708468387751,11.6603404761587));
#1730=CARTESIAN_POINT('Ctrl Pts',(-3.84264473622583,-26.6669563054752,11.5865392576738));
#1731=CARTESIAN_POINT('Ctrl Pts',(-3.87152605079722,-26.9382169121315,11.5620098124717));
#1732=CARTESIAN_POINT('Ctrl Pts',(-3.87149305127384,-27.4782945532475,11.5136784821176));
#1733=CARTESIAN_POINT('Ctrl Pts',(-3.84967986989137,-27.8368197194528,11.4890337583855));
#1734=CARTESIAN_POINT('Ctrl Pts',(-3.83481742436109,-28.1772296781916,11.4644896364825));
#1735=CARTESIAN_POINT('Ctrl Pts',(-3.5,-27.2127225901214,22.4975166120351));
#1736=CARTESIAN_POINT('Ctrl Pts',(-3.49927785868713,-27.7853287709716,22.4402329481162));
#1737=CARTESIAN_POINT('Ctrl Pts',(-3.35446180200001,-28.3588230843844,22.3829524737063));
#1738=CARTESIAN_POINT('Ctrl Pts',(-2.53808767932955,-29.8821237915549,22.2111091898206));
#1739=CARTESIAN_POINT('Ctrl Pts',(-1.46145231937317,-30.6017446798008,22.0965431657326));
#1740=CARTESIAN_POINT('Ctrl Pts',(0.860002585417323,-30.8282120086964,21.8674139251703));
#1741=CARTESIAN_POINT('Ctrl Pts',(2.07107291079633,-30.3270227433741,21.752849624791));
#1742=CARTESIAN_POINT('Ctrl Pts',(3.56721541815537,-28.5011179635623,21.5237157036811));
#1743=CARTESIAN_POINT('Ctrl Pts',(3.82659931701312,-27.20036017698,21.4091530749885));
#1744=CARTESIAN_POINT('Ctrl Pts',(3.13180267166131,-24.9149469548,21.1800146464357));
#1745=CARTESIAN_POINT('Ctrl Pts',(2.18342706770339,-23.9653744387647,21.0654536391327));
#1746=CARTESIAN_POINT('Ctrl Pts',(-0.129625104573071,-23.2648849532031,
20.8363108683544));
#1747=CARTESIAN_POINT('Ctrl Pts',(-1.46147591168062,-23.5287326354126,20.7217514337973));
#1748=CARTESIAN_POINT('Ctrl Pts',(-3.35090502810569,-25.0803600405907,20.4926044785548));
#1749=CARTESIAN_POINT('Ctrl Pts',(-3.87764741849126,-26.3487475764667,20.3780465697071));
#1750=CARTESIAN_POINT('Ctrl Pts',(-3.63479848762931,-28.8097762988588,20.148895580705));
#1751=CARTESIAN_POINT('Ctrl Pts',(-2.86427039073957,-29.9655693350743,20.0343391520621));
#1752=CARTESIAN_POINT('Ctrl Pts',(-0.65846096708456,-31.1444434869326,19.8051842733852));
#1753=CARTESIAN_POINT('Ctrl Pts',(0.74630206229462,-31.1460905834951,19.6906292809279));
#1754=CARTESIAN_POINT('Ctrl Pts',(2.97689487550167,-29.9540126226856,19.4614706503338));
#1755=CARTESIAN_POINT('Ctrl Pts',(3.76757285952208,-28.7739850439139,19.3469170514958));
#1756=CARTESIAN_POINT('Ctrl Pts',(4.0187034886225,-26.2291205871072,19.1177548007802));
#1757=CARTESIAN_POINT('Ctrl Pts',(3.47099870281935,-24.9015607577697,19.0032025543658));
#1758=CARTESIAN_POINT('Ctrl Pts',(1.47303203265274,-23.2608624483575,18.7740368097113));
#1759=CARTESIAN_POINT('Ctrl Pts',(0.0495881203952384,-22.9754752873616,
18.6594858758451));
#1760=CARTESIAN_POINT('Ctrl Pts',(-2.45155713850874,-23.7330678076998,18.4303167580854));
#1761=CARTESIAN_POINT('Ctrl Pts',(-3.49087258075457,-24.7690158719264,18.3157670982032));
#1762=CARTESIAN_POINT('Ctrl Pts',(-4.25893999689643,-27.296309020853,18.0865947230583));
#1763=CARTESIAN_POINT('Ctrl Pts',(-3.97210868158914,-28.7514045749302,17.9720462998272));
#1764=CARTESIAN_POINT('Ctrl Pts',(-2.27987387495177,-30.8159857353485,17.7428707782702));
#1765=CARTESIAN_POINT('Ctrl Pts',(-0.896249322735714,-31.3920519629118,
17.6283235555406));
#1766=CARTESIAN_POINT('Ctrl Pts',(1.11730388459739,-31.1951786270721,17.4564396343434));
#1767=CARTESIAN_POINT('Ctrl Pts',(1.77294326754581,-30.9607539401843,17.3991664653485));
#1768=CARTESIAN_POINT('Ctrl Pts',(2.90080505154166,-30.2083747949576,17.2845764438015));
#1769=CARTESIAN_POINT('Ctrl Pts',(3.37097187102428,-29.6899170424932,17.2273035618313));
#1770=CARTESIAN_POINT('Ctrl Pts',(4.01435276857721,-28.4885549672909,17.1127128120475));
#1771=CARTESIAN_POINT('Ctrl Pts',(4.18551725625119,-27.8061906781911,17.0554402129015));
#1772=CARTESIAN_POINT('Ctrl Pts',(4.18667681067326,-26.4363846241478,16.9408487471063));
#1773=CARTESIAN_POINT('Ctrl Pts',(4.01512628257138,-25.7503981626563,16.8835764266556));
#1774=CARTESIAN_POINT('Ctrl Pts',(3.3671797883428,-24.5355762087865,16.7689842568497));
#1775=CARTESIAN_POINT('Ctrl Pts',(2.89011927690729,-24.0087606262116,16.7117122110268));
#1776=CARTESIAN_POINT('Ctrl Pts',(1.74022544089816,-23.2388741548863,16.5971193489555));
#1777=CARTESIAN_POINT('Ctrl Pts',(1.06777289997686,-22.997899001297,16.5398475737628));
#1778=CARTESIAN_POINT('Ctrl Pts',(-0.316234927853767,-22.8602246903861,
16.4252540309383));
#1779=CARTESIAN_POINT('Ctrl Pts',(-1.02645305770396,-22.9651883959601,16.3679825224341));
#1780=CARTESIAN_POINT('Ctrl Pts',(-2.31843866837204,-23.4988107570144,16.253388310152));
#1781=CARTESIAN_POINT('Ctrl Pts',(-2.89823397310667,-23.9282941364198,16.196117064454));
#1782=CARTESIAN_POINT('Ctrl Pts',(-3.79061110505536,-25.0133228623296,16.0815221937778));
#1783=CARTESIAN_POINT('Ctrl Pts',(-4.10106225113868,-25.6686515734845,16.0242512070742));
#1784=CARTESIAN_POINT('Ctrl Pts',(-4.37801831770041,-27.0530868844925,15.909655688838));
#1785=CARTESIAN_POINT('Ctrl Pts',(-4.34275064929299,-27.7809842375283,15.8523849573772));
#1786=CARTESIAN_POINT('Ctrl Pts',(-3.93241076591198,-29.1392277168195,15.7377888022123));
#1787=CARTESIAN_POINT('Ctrl Pts',(-3.55635559774948,-29.7676616996119,15.6805183222975));
#1788=CARTESIAN_POINT('Ctrl Pts',(-2.5492848357845,-30.7770911827345,15.5659215406245));
#1789=CARTESIAN_POINT('Ctrl Pts',(-1.91831750124282,-31.1559328914483,15.508651308613));
#1790=CARTESIAN_POINT('Ctrl Pts',(-0.547630823615979,-31.573532596127,15.3940539106591));
#1791=CARTESIAN_POINT('Ctrl Pts',(0.191016654419482,-31.6104167135759,15.3367839229662));
#1792=CARTESIAN_POINT('Ctrl Pts',(1.60359332885263,-31.3312616639846,15.2221859187487));
#1793=CARTESIAN_POINT('Ctrl Pts',(2.27568288412789,-31.0140842055001,15.1649161718489));
#1794=CARTESIAN_POINT('Ctrl Pts',(3.39532523069409,-30.0976087977106,15.0503175711959));
#1795=CARTESIAN_POINT('Ctrl Pts',(3.84071356306253,-29.4981872635055,14.9930480616187));
#1796=CARTESIAN_POINT('Ctrl Pts',(4.39886200638194,-28.1556824953451,14.8784488741645));
#1797=CARTESIAN_POINT('Ctrl Pts',(4.50965629588013,-27.4135246591517,14.821179598491));
#1798=CARTESIAN_POINT('Ctrl Pts',(4.36841850750692,-25.9594545017938,14.7065798336947));
#1799=CARTESIAN_POINT('Ctrl Pts',(4.11509669119356,-25.2492967556584,14.649310788563));
#1800=CARTESIAN_POINT('Ctrl Pts',(3.301248674694,-24.027643879362,14.5347104556859));
#1801=CARTESIAN_POINT('Ctrl Pts',(2.7404244263817,-23.5183108657722,14.4774416377848));
#1802=CARTESIAN_POINT('Ctrl Pts',(1.44064112961331,-22.8212020237703,14.3628407459321));
#1803=CARTESIAN_POINT('Ctrl Pts',(0.702452411780137,-22.6354736977066,14.3055721519949));
#1804=CARTESIAN_POINT('Ctrl Pts',(-0.779472887126354,-22.6333352967227,
14.190970710093));
#1805=CARTESIAN_POINT('Ctrl Pts',(-1.52155253015143,-22.8183614641083,14.1337023369077));
#1806=CARTESIAN_POINT('Ctrl Pts',(-2.83570509877543,-23.5183020242021,14.0191003537129));
#1807=CARTESIAN_POINT('Ctrl Pts',(-3.40563177267265,-24.0336906113064,13.9618321981179));
#1808=CARTESIAN_POINT('Ctrl Pts',(-4.23859829449245,-25.2762621036854,13.8472296822221));
#1809=CARTESIAN_POINT('Ctrl Pts',(-4.49952012993745,-26.0028377560707,13.7899617411021));
#1810=CARTESIAN_POINT('Ctrl Pts',(-4.64912831734354,-27.4983091479623,13.6753587009413));
#1811=CARTESIAN_POINT('Ctrl Pts',(-4.53623796107103,-28.2656580682614,13.6180909712297));
#1812=CARTESIAN_POINT('Ctrl Pts',(-3.96059130788698,-29.6615610540449,13.5034874150766));
#1813=CARTESIAN_POINT('Ctrl Pts',(-3.49718400748527,-30.2879987021829,13.4462198937543));
#1814=CARTESIAN_POINT('Ctrl Pts',(-2.32610691316009,-31.2522011376172,13.3316158297333));
#1815=CARTESIAN_POINT('Ctrl Pts',(-1.61887397941475,-31.5877894623157,13.2743485138248));
#1816=CARTESIAN_POINT('Ctrl Pts',(-0.124698014175552,-31.8875168697119,
13.1597439499104));
#1817=CARTESIAN_POINT('Ctrl Pts',(0.660820605236803,-31.8499459440715,13.1024768364861));
#1818=CARTESIAN_POINT('Ctrl Pts',(2.12657161732859,-31.4079510480467,12.9878717805055));
#1819=CARTESIAN_POINT('Ctrl Pts',(2.8047317654823,-31.0026997016065,12.9306048666812));
#1820=CARTESIAN_POINT('Ctrl Pts',(3.89404127890867,-29.9170320609718,12.8159993263168));
#1821=CARTESIAN_POINT('Ctrl Pts',(4.30296864843086,-29.2368757228388,12.7587326092554));
#1822=CARTESIAN_POINT('Ctrl Pts',(4.75395585015817,-27.7592219594744,12.6441265920449));
#1823=CARTESIAN_POINT('Ctrl Pts',(4.79418068964257,-26.9630145561609,12.5868600689426));
#1824=CARTESIAN_POINT('Ctrl Pts',(4.49404010690874,-25.4403710926243,12.4722535823103));
#1825=CARTESIAN_POINT('Ctrl Pts',(4.15267254437464,-24.7159484861244,12.4149872504092));
#1826=CARTESIAN_POINT('Ctrl Pts',(3.16580254027823,-23.5091389781496,12.3003803016153));
#1827=CARTESIAN_POINT('Ctrl Pts',(2.52037754996715,-23.0290058774741,12.2431141582025));
#1828=CARTESIAN_POINT('Ctrl Pts',(1.07470328235808,-22.427176726376,12.1285067543989));
#1829=CARTESIAN_POINT('Ctrl Pts',(0.275598076802496,-22.3074311776151,12.0712407967975));
#1830=CARTESIAN_POINT('Ctrl Pts',(-1.84868379116737,-22.5127927449768,11.9157393755432));
#1831=CARTESIAN_POINT('Ctrl Pts',(-3.12606319175256,-23.2393767520925,11.8175853786087));
#1832=CARTESIAN_POINT('Ctrl Pts',(-4.33213271301493,-24.880386526967,11.6703268381421));
#1833=CARTESIAN_POINT('Ctrl Pts',(-4.61678084393395,-25.5145917668544,11.6212300753262));
#1834=CARTESIAN_POINT('Ctrl Pts',(-4.8325074990541,-26.51374965466,11.547605629606));
#1835=CARTESIAN_POINT('Ctrl Pts',(-4.86981537831802,-26.8545716453141,11.5230623381901));
#1836=CARTESIAN_POINT('Ctrl Pts',(-4.87150546249911,-27.5373956033118,11.4739637523339));
#1837=CARTESIAN_POINT('Ctrl Pts',(-4.84806449389349,-27.8775537395237,11.4494246411902));
#1838=CARTESIAN_POINT('Ctrl Pts',(-4.8332020483632,-28.2179636982637,11.4248805192881));
#1839=CARTESIAN_POINT('Ctrl Pts',(-4.49992531496781,-27.2005618150104,22.4987331790167));
#1840=CARTESIAN_POINT('Ctrl Pts',(-4.50123266577206,-27.9399345555106,22.4403537839278));
#1841=CARTESIAN_POINT('Ctrl Pts',(-4.31885456358521,-28.6714666153785,22.3845992765752));
#1842=CARTESIAN_POINT('Ctrl Pts',(-3.27206873853112,-30.6387455869407,22.2092430694354));
#1843=CARTESIAN_POINT('Ctrl Pts',(-1.90301347052226,-31.5589454854703,22.0978648836455));
#1844=CARTESIAN_POINT('Ctrl Pts',(1.08133745456905,-31.8588483286696,21.8641055935273));
#1845=CARTESIAN_POINT('Ctrl Pts',(2.62163729847883,-31.2259625043182,21.7526920522415));
#1846=CARTESIAN_POINT('Ctrl Pts',(4.54712383673962,-28.889667640373,21.5189807362004));
#1847=CARTESIAN_POINT('Ctrl Pts',(4.87991725612086,-27.2420071964223,21.4075326300492));
#1848=CARTESIAN_POINT('Ctrl Pts',(3.99926793651637,-24.3160463481836,21.1738683059317));
#1849=CARTESIAN_POINT('Ctrl Pts',(2.80324492166405,-23.1127118024641,21.0623863989465));
#1850=CARTESIAN_POINT('Ctrl Pts',(-0.145664295624094,-22.2108911563125,
20.8287681139101));
#1851=CARTESIAN_POINT('Ctrl Pts',(-1.82608753442347,-22.5396643242445,20.7172531447498));
#1852=CARTESIAN_POINT('Ctrl Pts',(-4.23617685498116,-24.5081432429562,20.4836799735107));
#1853=CARTESIAN_POINT('Ctrl Pts',(-4.90258935139331,-26.1024197715759,20.3721326565532));
#1854=CARTESIAN_POINT('Ctrl Pts',(-4.60239401978947,-29.2279523583354,20.1386037010885));
#1855=CARTESIAN_POINT('Ctrl Pts',(-3.63850146388098,-30.6809230335259,20.0270247275001));
#1856=CARTESIAN_POINT('Ctrl Pts',(-0.848312218451317,-32.1812843569572,
19.7935391153079));
#1857=CARTESIAN_POINT('Ctrl Pts',(0.910962191510308,-32.187257662144,19.6819291541039));
#1858=CARTESIAN_POINT('Ctrl Pts',(3.73351916376344,-30.6878849222468,19.4484860378945));
#1859=CARTESIAN_POINT('Ctrl Pts',(4.72474370347859,-29.2155039993741,19.3368457367663));
#1860=CARTESIAN_POINT('Ctrl Pts',(5.04923349895883,-26.0077171480983,19.103444293163));
#1861=CARTESIAN_POINT('Ctrl Pts',(4.36986673206198,-24.3509968931086,18.9917742794446));
#1862=CARTESIAN_POINT('Ctrl Pts',(1.86145168328288,-22.2810150440159,18.7584137083719));
#1863=CARTESIAN_POINT('Ctrl Pts',(0.0911844603756664,-21.9222328729832,
18.6467145899854));
#1864=CARTESIAN_POINT('Ctrl Pts',(-3.05047794174479,-22.8657614168808,18.4133941133931));
#1865=CARTESIAN_POINT('Ctrl Pts',(-4.3434939460169,-24.1492993667947,18.3016664794364));
#1866=CARTESIAN_POINT('Ctrl Pts',(-5.31279863706187,-27.3124610697944,18.0683853413922));
#1867=CARTESIAN_POINT('Ctrl Pts',(-4.96105242549078,-29.116041915327,17.9566297629436));
#1868=CARTESIAN_POINT('Ctrl Pts',(-2.85190795720616,-31.7012004702625,17.7233872278977));
#1869=CARTESIAN_POINT('Ctrl Pts',(-1.14247440761136,-32.4168925823255,17.6116042590234));
#1870=CARTESIAN_POINT('Ctrl Pts',(1.36942113919458,-32.1769364386145,17.4367007733733));
#1871=CARTESIAN_POINT('Ctrl Pts',(2.17863030294074,-31.8896680393015,17.3807991645495));
#1872=CARTESIAN_POINT('Ctrl Pts',(3.58594774059714,-30.955345510934,17.2642061815091));
#1873=CARTESIAN_POINT('Ctrl Pts',(4.1666380278044,-30.3178934995088,17.2082979257248));
#1874=CARTESIAN_POINT('Ctrl Pts',(4.97070480320723,-28.8243377732163,17.0917141975888));
#1875=CARTESIAN_POINT('Ctrl Pts',(5.18324736692089,-27.9849325707496,17.0357993595099));
#1876=CARTESIAN_POINT('Ctrl Pts',(5.18837634682399,-26.2816906794162,16.9192248016874));
#1877=CARTESIAN_POINT('Ctrl Pts',(4.97928961288882,-25.4377044137181,16.8633034450976));
#1878=CARTESIAN_POINT('Ctrl Pts',(4.17766130573194,-23.9269514586941,16.7467379739209));
#1879=CARTESIAN_POINT('Ctrl Pts',(3.59301796923098,-23.2784899136664,16.6908101616495));
#1880=CARTESIAN_POINT('Ctrl Pts',(2.16808835767185,-22.3200655571735,16.5742536948244));
#1881=CARTESIAN_POINT('Ctrl Pts',(1.34341569002319,-22.0225242875423,16.5183194887516));
#1882=CARTESIAN_POINT('Ctrl Pts',(-0.37202542262785,-21.848229520912,16.4017719448942));
#1883=CARTESIAN_POINT('Ctrl Pts',(-1.2431512747268,-21.9750627042462,16.3458314060321));
#1884=CARTESIAN_POINT('Ctrl Pts',(-2.84469319036191,-22.6326276198057,16.2292927049662));
#1885=CARTESIAN_POINT('Ctrl Pts',(-3.55608395141779,-23.1572481132965,16.1733458934499));
#1886=CARTESIAN_POINT('Ctrl Pts',(-4.66303405570225,-24.4975081087771,16.0568159559262));
#1887=CARTESIAN_POINT('Ctrl Pts',(-5.0446924336988,-25.2987711172549,16.0008629310603));
#1888=CARTESIAN_POINT('Ctrl Pts',(-5.39056519898843,-27.0094466251327,15.8843416789414));
#1889=CARTESIAN_POINT('Ctrl Pts',(-5.34930304043553,-27.8996098051487,15.8283824991195));
#1890=CARTESIAN_POINT('Ctrl Pts',(-4.84595092330871,-29.5780539034839,15.7118698553524));
#1891=CARTESIAN_POINT('Ctrl Pts',(-4.38811855967175,-30.3467642405488,15.6559045781531));
#1892=CARTESIAN_POINT('Ctrl Pts',(-3.14807661476919,-31.5947342749175,15.5394004666024));
#1893=CARTESIAN_POINT('Ctrl Pts',(-2.37886502949379,-32.0587365058605,15.4834291488454));
#1894=CARTESIAN_POINT('Ctrl Pts',(-0.690271412805203,-32.5768833169426,
15.3669334943444));
#1895=CARTESIAN_POINT('Ctrl Pts',(0.210437406783647,-32.6237032613599,15.3109561919855));
#1896=CARTESIAN_POINT('Ctrl Pts',(1.95077582228988,-32.2833593081943,15.1944689204932));
#1897=CARTESIAN_POINT('Ctrl Pts',(2.77047067840731,-31.8985499371097,15.1384856887274));
#1898=CARTESIAN_POINT('Ctrl Pts',(4.15032302098314,-30.7736043375475,15.0220067269618));
#1899=CARTESIAN_POINT('Ctrl Pts',(4.69400309684405,-30.0449584837519,14.9660176202321));
#1900=CARTESIAN_POINT('Ctrl Pts',(5.38335863834062,-28.395939593178,14.8495468960155));
#1901=CARTESIAN_POINT('Ctrl Pts',(5.51992097583071,-27.4934852178884,14.7935519679768));
#1902=CARTESIAN_POINT('Ctrl Pts',(5.34990401728289,-25.7072478702335,14.6770894099612));
#1903=CARTESIAN_POINT('Ctrl Pts',(5.04374456081733,-24.8435781449226,14.6210887135337));
#1904=CARTESIAN_POINT('Ctrl Pts',(4.0479320191368,-23.342552408645,14.5046342513644));
#1905=CARTESIAN_POINT('Ctrl Pts',(3.36814614645295,-22.7227447945842,14.4486278387742));
#1906=CARTESIAN_POINT('Ctrl Pts',(1.77619102970885,-21.8650344590564,14.3321814028423));
#1907=CARTESIAN_POINT('Ctrl Pts',(0.881013595157293,-21.6379564042767,14.2761693255965));
#1908=CARTESIAN_POINT('Ctrl Pts',(-0.934286602741275,-21.631913240891,14.1597308473328));
#1909=CARTESIAN_POINT('Ctrl Pts',(-1.83430603011931,-21.85447637771,14.1037131561842));
#1910=CARTESIAN_POINT('Ctrl Pts',(-3.44430347736566,-22.7081266226923,13.9872825678333));
#1911=CARTESIAN_POINT('Ctrl Pts',(-4.13582211102842,-23.3310704412515,13.9312593128857));
#1912=CARTESIAN_POINT('Ctrl Pts',(-5.15723598600513,-24.8486604334571,13.8148365475172));
#1913=CARTESIAN_POINT('Ctrl Pts',(-5.47468869489397,-25.7274061109226,13.7588077782201));
#1914=CARTESIAN_POINT('Ctrl Pts',(-5.66084498304722,-27.5542511137055,13.6423927697258));
#1915=CARTESIAN_POINT('Ctrl Pts',(-5.52607729259019,-28.4824463986154,13.5863585348362));
#1916=CARTESIAN_POINT('Ctrl Pts',(-4.82645265952584,-30.1878171234494,13.4699512180057));
#1917=CARTESIAN_POINT('Ctrl Pts',(-4.26793016275464,-30.9457917464557,13.4139115656321));
#1918=CARTESIAN_POINT('Ctrl Pts',(-2.84163338331343,-32.1244708835282,13.2975118759857));
#1919=CARTESIAN_POINT('Ctrl Pts',(-1.98851329456531,-32.5312245863753,13.2414668535995));
#1920=CARTESIAN_POINT('Ctrl Pts',(-0.168154346495923,-32.8997884885716,
13.1250747275302));
#1921=CARTESIAN_POINT('Ctrl Pts',(0.779568298212397,-32.8562079727566,13.0690243819638));
#1922=CARTESIAN_POINT('Ctrl Pts',(2.56542990953642,-32.3211571768756,12.9526397565944));
#1923=CARTESIAN_POINT('Ctrl Pts',(3.38380416962575,-31.8341443288812,12.8965841340846));
#1924=CARTESIAN_POINT('Ctrl Pts',(4.71155278837089,-30.5155103343138,12.7802069473221));
#1925=CARTESIAN_POINT('Ctrl Pts',(5.20559259369133,-29.6971531119313,12.7241460934996));
#1926=CARTESIAN_POINT('Ctrl Pts',(5.75703886090729,-27.9016459598323,12.6077762839981));
#1927=CARTESIAN_POINT('Ctrl Pts',(5.80717713818053,-26.9434385648419,12.5517102438793));
#1928=CARTESIAN_POINT('Ctrl Pts',(5.44579520263474,-25.0931237590171,12.4353477510898));
#1929=CARTESIAN_POINT('Ctrl Pts',(5.0368047411671,-24.2211610859936,12.3792765691091));
#1930=CARTESIAN_POINT('Ctrl Pts',(3.84146164273372,-22.7542474974693,12.2629213331626));
#1931=CARTESIAN_POINT('Ctrl Pts',(3.06685116348872,-22.1758765063834,12.2068450531984));
#1932=CARTESIAN_POINT('Ctrl Pts',(1.3147114679644,-21.4429359570459,12.0904970149672));
#1933=CARTESIAN_POINT('Ctrl Pts',(0.355369734306315,-21.2974519808943,12.0344156803179));
#1934=CARTESIAN_POINT('Ctrl Pts',(-2.21947927012219,-21.541945111076,11.8765628382364));
#1935=CARTESIAN_POINT('Ctrl Pts',(-3.75768230547338,-22.4163266113853,11.7792514363029));
#1936=CARTESIAN_POINT('Ctrl Pts',(-5.21498730250992,-24.3919766537203,11.6318625545005));
#1937=CARTESIAN_POINT('Ctrl Pts',(-5.56061254440886,-25.1583366949337,11.5821196744937));
#1938=CARTESIAN_POINT('Ctrl Pts',(-5.82237026188237,-26.3605430038448,11.5086720015383));
#1939=CARTESIAN_POINT('Ctrl Pts',(-5.86810470583882,-26.7709263784967,11.4841148639085));
#1940=CARTESIAN_POINT('Ctrl Pts',(-5.87151787372438,-27.5964966533761,11.4342490225503));
#1941=CARTESIAN_POINT('Ctrl Pts',(-5.8464491178956,-27.9182877595946,11.4098155239949));
#1942=CARTESIAN_POINT('Ctrl Pts',(-5.83158667236532,-28.2586977183358,11.3852714020937));
#1943=CARTESIAN_POINT('Ctrl Pts',(-4.49992531496781,-27.1010184425723,21.5036999549465));
#1944=CARTESIAN_POINT('Ctrl Pts',(-4.51674600628465,-27.8405511731054,21.4453045543583));
#1945=CARTESIAN_POINT('Ctrl Pts',(-4.3513754570227,-28.5765453512511,21.3895276624965));
#1946=CARTESIAN_POINT('Ctrl Pts',(-3.34502119885618,-30.5657740901924,21.2141080231263));
#1947=CARTESIAN_POINT('Ctrl Pts',(-1.99683196222126,-31.5170666924607,21.1026952188504));
#1948=CARTESIAN_POINT('Ctrl Pts',(0.980993279522333,-31.8772272555485,20.8688610765165));
#1949=CARTESIAN_POINT('Ctrl Pts',(2.53490239289457,-31.2787547245274,20.7574094693259));
#1950=CARTESIAN_POINT('Ctrl Pts',(4.50569444399399,-28.9816631968142,20.5236326621716));
#1951=CARTESIAN_POINT('Ctrl Pts',(4.87413701918684,-27.3422265898772,20.41214314674));
#1952=CARTESIAN_POINT('Ctrl Pts',(4.05086560996824,-24.4015014064168,20.1784223463925));
#1953=CARTESIAN_POINT('Ctrl Pts',(2.88154677707693,-23.173754043832,20.0668957873436));
#1954=CARTESIAN_POINT('Ctrl Pts',(-0.0470467715653138,-22.2169532717186,
19.8332297105388));
#1955=CARTESIAN_POINT('Ctrl Pts',(-1.73235777827075,-22.5102673549153,19.7216669438178));
#1956=CARTESIAN_POINT('Ctrl Pts',(-4.17572182242301,-24.4312269013205,19.4880543497385));
#1957=CARTESIAN_POINT('Ctrl Pts',(-4.87376845888169,-26.0095620732211,19.3764561838128));
#1958=CARTESIAN_POINT('Ctrl Pts',(-4.6310120681261,-29.1353686231182,19.1428958730047));
#1959=CARTESIAN_POINT('Ctrl Pts',(-3.69789395427398,-30.6051559498652,19.0312630900414));
#1960=CARTESIAN_POINT('Ctrl Pts',(-0.939901316815822,-32.1524297385279,
18.797753901872));
#1961=CARTESIAN_POINT('Ctrl Pts',(0.815770716897848,-32.192946710534,18.6860872589115));
#1962=CARTESIAN_POINT('Ctrl Pts',(3.65834639903831,-30.746287086809,18.4526280705631));
#1963=CARTESIAN_POINT('Ctrl Pts',(4.67570856491877,-29.2962834910467,18.3409283004432));
#1964=CARTESIAN_POINT('Ctrl Pts',(5.05445235298275,-26.1019770515496,18.1075180249339));
#1965=CARTESIAN_POINT('Ctrl Pts',(4.40805306181254,-24.4365392522985,17.9957858373769));
#1966=CARTESIAN_POINT('Ctrl Pts',(1.94130016670179,-22.3299662886282,17.7624234222861));
#1967=CARTESIAN_POINT('Ctrl Pts',(0.182492857305352,-21.939377617945,17.6506595049407));
#1968=CARTESIAN_POINT('Ctrl Pts',(-2.96543044577777,-22.8282401952741,17.4173439305767));
#1969=CARTESIAN_POINT('Ctrl Pts',(-4.27794385851622,-24.0844995025642,17.3055489496951));
#1970=CARTESIAN_POINT('Ctrl Pts',(-5.29537653242634,-27.2218242153782,17.0722792286103));
#1971=CARTESIAN_POINT('Ctrl Pts',(-4.97689278167529,-29.0259395054587,16.9604538299531));
#1972=CARTESIAN_POINT('Ctrl Pts',(-2.91608530249191,-31.6357336752382,16.7272290046934));
#1973=CARTESIAN_POINT('Ctrl Pts',(-1.22497985084763,-32.3788890909175,16.6153738146158));
#1974=CARTESIAN_POINT('Ctrl Pts',(1.28145612063066,-32.1789932923933,16.4404881713498));
#1975=CARTESIAN_POINT('Ctrl Pts',(2.0927818601203,-31.9069109397873,16.3845495671917));
#1976=CARTESIAN_POINT('Ctrl Pts',(3.50922640420288,-30.9978632225545,16.2679699605668));
#1977=CARTESIAN_POINT('Ctrl Pts',(4.09881550944335,-30.3728309488599,16.2120241353908));
#1978=CARTESIAN_POINT('Ctrl Pts',(4.92262783581331,-28.8973868790768,16.0954552401651));
#1979=CARTESIAN_POINT('Ctrl Pts',(5.14877399302525,-28.064821040575,16.0395022670422));
#1980=CARTESIAN_POINT('Ctrl Pts',(5.17972192673461,-26.3684552205223,15.9229439741396));
#1981=CARTESIAN_POINT('Ctrl Pts',(4.98580796318786,-25.5242055246215,15.8669839251149));
#1982=CARTESIAN_POINT('Ctrl Pts',(4.21017429044416,-24.0075929294983,15.7504361268929));
#1983=CARTESIAN_POINT('Ctrl Pts',(3.63880072013838,-23.351872300329,15.6944690729279));
#1984=CARTESIAN_POINT('Ctrl Pts',(2.23413550967172,-22.3762507712042,15.5779316635816));
#1985=CARTESIAN_POINT('Ctrl Pts',(1.41781408360257,-22.0661561590653,15.5219576745624));
#1986=CARTESIAN_POINT('Ctrl Pts',(-0.2876678119969,-21.8672909533799,15.4054305496812));
#1987=CARTESIAN_POINT('Ctrl Pts',(-1.15723576718454,-21.9791742088117,15.349449694498));
#1988=CARTESIAN_POINT('Ctrl Pts',(-2.76133682475571,-22.6104139372597,15.2329327513282));
#1989=CARTESIAN_POINT('Ctrl Pts',(-3.47827719059933,-23.1211141138698,15.1769450978676));
#1990=CARTESIAN_POINT('Ctrl Pts',(-4.59966549973914,-24.4392847330131,15.0604382350449));
#1991=CARTESIAN_POINT('Ctrl Pts',(-4.99267244674646,-25.2308278340738,15.0044438502435));
#1992=CARTESIAN_POINT('Ctrl Pts',(-5.36152867501004,-26.9286517721488,14.8879469679338));
#1993=CARTESIAN_POINT('Ctrl Pts',(-5.33479062947237,-27.815489816777,14.8319459176988));
#1994=CARTESIAN_POINT('Ctrl Pts',(-4.85770689425811,-29.4932029850683,14.7154589175941));
#1995=CARTESIAN_POINT('Ctrl Pts',(-4.41424130928336,-30.2657064039853,14.6594512668976));
#1996=CARTESIAN_POINT('Ctrl Pts',(-3.19776731478627,-31.5251842790945,14.5429740520141));
#1997=CARTESIAN_POINT('Ctrl Pts',(-2.43948640778453,-31.9991936236663,14.4869598649523));
#1998=CARTESIAN_POINT('Ctrl Pts',(-0.76641117646687,-32.538424291025,14.3704923396933));
#1999=CARTESIAN_POINT('Ctrl Pts',(0.129280639488567,-32.5991484080323,14.3144716793848));
#2000=CARTESIAN_POINT('Ctrl Pts',(1.86565117755554,-32.2846351962422,14.1980137496642));
#2001=CARTESIAN_POINT('Ctrl Pts',(2.6873584363981,-31.9144328140864,14.1419866783607));
#2002=CARTESIAN_POINT('Ctrl Pts',(4.0756575425974,-30.8141731242952,14.025538251239));
#2003=CARTESIAN_POINT('Ctrl Pts',(4.62788574697171,-30.0974982118229,13.9695048303297));
#2004=CARTESIAN_POINT('Ctrl Pts',(5.33614212196108,-28.4664074366612,13.8530658143517));
#2005=CARTESIAN_POINT('Ctrl Pts',(5.48580553915912,-27.5705664905401,13.7970261043234));
#2006=CARTESIAN_POINT('Ctrl Pts',(5.34081184824442,-25.791439376031,13.6805964092432));
#2007=CARTESIAN_POINT('Ctrl Pts',(5.04929361698828,-24.927539264489,13.6245504697451));
#2008=CARTESIAN_POINT('Ctrl Pts',(4.07891464172889,-23.4212168574546,13.5081300066553));
#2009=CARTESIAN_POINT('Ctrl Pts',(3.41195903484832,-22.794417393971,13.4520778965404));
#2010=CARTESIAN_POINT('Ctrl Pts',(1.84005664325852,-21.9202404356125,13.3356665776424));
#2011=CARTESIAN_POINT('Ctrl Pts',(0.952974962988242,-21.6810345955686,13.2796083549412));
#2012=CARTESIAN_POINT('Ctrl Pts',(-0.852207019879878,-21.6511301665541,
13.1632060938123));
#2013=CARTESIAN_POINT('Ctrl Pts',(-1.75069597922114,-21.8592211322789,13.1071418157038));
#2014=CARTESIAN_POINT('Ctrl Pts',(-3.36279321619093,-22.687065563139,12.9907485270725));
#2015=CARTESIAN_POINT('Ctrl Pts',(-4.0596712085529,-23.2965088909024,12.9346782499817));
#2016=CARTESIAN_POINT('Ctrl Pts',(-5.09490115062812,-24.7922309126811,12.8182938497412));
#2017=CARTESIAN_POINT('Ctrl Pts',(-5.42335290963779,-25.6615296657728,12.7622176293468));
#2018=CARTESIAN_POINT('Ctrl Pts',(-5.6318733184926,-27.4754205110425,12.6458420345123));
#2019=CARTESIAN_POINT('Ctrl Pts',(-5.51121048465282,-28.4003675711241,12.5897599257099));
#2020=CARTESIAN_POINT('Ctrl Pts',(-4.83738798718038,-30.1046366902265,12.4733930545196));
#2021=CARTESIAN_POINT('Ctrl Pts',(-4.29284127804266,-30.8662836546237,12.4173051114547));
#2022=CARTESIAN_POINT('Ctrl Pts',(-2.88989812922953,-32.0559489908963,12.3009468831881));
#2023=CARTESIAN_POINT('Ctrl Pts',(-2.04742969825749,-32.4724339533943,12.244853159285));
#2024=CARTESIAN_POINT('Ctrl Pts',(-0.2426536662203,-32.8615528897918,12.1285034943741));
#2025=CARTESIAN_POINT('Ctrl Pts',(0.700167228706349,-32.8315189484388,12.0724040423241));
#2026=CARTESIAN_POINT('Ctrl Pts',(2.48176316317964,-32.3218947112272,11.9560628622509));
#2027=CARTESIAN_POINT('Ctrl Pts',(3.30209026051788,-31.8491345603716,11.8999577340539));
#2028=CARTESIAN_POINT('Ctrl Pts',(4.63785467742761,-30.5549942620067,11.7836249613568));
#2029=CARTESIAN_POINT('Ctrl Pts',(5.14023670521377,-29.7483336343732,11.7275142083257));
#2030=CARTESIAN_POINT('Ctrl Pts',(5.71014369190083,-27.9707987230122,11.6111897665715));
#2031=CARTESIAN_POINT('Ctrl Pts',(5.77308874181379,-27.0190622633568,11.5550734393245));
#2032=CARTESIAN_POINT('Ctrl Pts',(5.43639437006847,-25.1760989492496,11.4387572531387));
#2033=CARTESIAN_POINT('Ctrl Pts',(5.04173404968112,-24.3039132848956,11.3826354016244));
#2034=CARTESIAN_POINT('Ctrl Pts',(3.87166745943498,-22.8320547671859,11.2663273965984));
#2035=CARTESIAN_POINT('Ctrl Pts',(3.10962740498996,-22.2468328201306,11.2102000701237));
#2036=CARTESIAN_POINT('Ctrl Pts',(1.3775808247441,-21.4977812085784,11.0939001728392));
#2037=CARTESIAN_POINT('Ctrl Pts',(0.426176004646674,-21.3404003073863,11.0377674200549));
#2038=CARTESIAN_POINT('Ctrl Pts',(-2.13467139062884,-21.5528754416251,10.8799811119317));
#2039=CARTESIAN_POINT('Ctrl Pts',(-3.67375330512296,-22.4019087871921,10.7826247286485));
#2040=CARTESIAN_POINT('Ctrl Pts',(-5.14572845587871,-24.3467779409998,10.6352234649416));
#2041=CARTESIAN_POINT('Ctrl Pts',(-5.4980087978572,-25.10396329861,10.585497622957));
#2042=CARTESIAN_POINT('Ctrl Pts',(-5.77284291612865,-26.2950238657267,10.5120341100286));
#2043=CARTESIAN_POINT('Ctrl Pts',(-5.82326382778836,-26.7021580375338,10.4874753114238));
#2044=CARTESIAN_POINT('Ctrl Pts',(-5.83613711196663,-27.5221379313639,10.4376301541696));
#2045=CARTESIAN_POINT('Ctrl Pts',(-5.80990657648216,-27.8448337026384,10.4131866340964));
#2046=CARTESIAN_POINT('Ctrl Pts',(-5.79504413095202,-28.1852436613808,10.3886425121934));
#2047=CARTESIAN_POINT('Ctrl Pts',(-3.5,-27.1131792176833,21.5024833879649));
#2048=CARTESIAN_POINT('Ctrl Pts',(-3.51479119919922,-27.6859453885664,21.4451837185487));
#2049=CARTESIAN_POINT('Ctrl Pts',(-3.3869826954375,-28.2639018202575,21.3878808596267));
#2050=CARTESIAN_POINT('Ctrl Pts',(-2.61104013965461,-29.8091522948055,21.2159741435134));
#2051=CARTESIAN_POINT('Ctrl Pts',(-1.55527081107218,-30.5598658867912,21.1013735009366));
#2052=CARTESIAN_POINT('Ctrl Pts',(0.7596584103706,-30.8465909355752,20.8721694081605));
#2053=CARTESIAN_POINT('Ctrl Pts',(1.98433800521209,-30.3798149635844,20.7575670418755));
#2054=CARTESIAN_POINT('Ctrl Pts',(3.52578602540974,-28.5931135200025,20.5283676296524));
#2055=CARTESIAN_POINT('Ctrl Pts',(3.8208190800791,-27.3005795704328,20.4137635916772));
#2056=CARTESIAN_POINT('Ctrl Pts',(3.18340034511317,-25.0004020130352,20.1845686868986));
#2057=CARTESIAN_POINT('Ctrl Pts',(2.26172892311522,-24.0264166801336,20.0699630275308));
#2058=CARTESIAN_POINT('Ctrl Pts',(-0.0310075805132356,-23.2709470686081,
19.840772464982));
#2059=CARTESIAN_POINT('Ctrl Pts',(-1.36774615552683,-23.4993356660845,19.7261652328664));
#2060=CARTESIAN_POINT('Ctrl Pts',(-3.29044999554861,-25.003443698954,19.4969788547815));
#2061=CARTESIAN_POINT('Ctrl Pts',(-3.84882652597964,-26.255889878113,19.3823700969656));
#2062=CARTESIAN_POINT('Ctrl Pts',(-3.66341653596594,-28.7171925636406,19.1531877526223));
#2063=CARTESIAN_POINT('Ctrl Pts',(-2.92366288113256,-29.8898022514147,19.0385775146034));
#2064=CARTESIAN_POINT('Ctrl Pts',(-0.750050065449063,-31.1155888685023,
18.8093990599493));
#2065=CARTESIAN_POINT('Ctrl Pts',(0.651110587682156,-31.1517796318851,18.6947873857344));
#2066=CARTESIAN_POINT('Ctrl Pts',(2.90172211077653,-30.0124147872479,18.4656126830036));
#2067=CARTESIAN_POINT('Ctrl Pts',(3.71853772096227,-28.8547645355866,18.3509996151738));
#2068=CARTESIAN_POINT('Ctrl Pts',(4.02392234264642,-26.3233804905586,18.1218285325501));
#2069=CARTESIAN_POINT('Ctrl Pts',(3.50918503257104,-24.9871031169595,18.0072141122992));
#2070=CARTESIAN_POINT('Ctrl Pts',(1.55288051607053,-23.3098136929698,17.7780465236243));
#2071=CARTESIAN_POINT('Ctrl Pts',(0.140896517323791,-22.9926200323223,17.6634307908027));
#2072=CARTESIAN_POINT('Ctrl Pts',(-2.36650964254058,-23.6955465860942,17.4342665752667));
#2073=CARTESIAN_POINT('Ctrl Pts',(-3.42532249325332,-24.7042160076948,17.319649568463));
#2074=CARTESIAN_POINT('Ctrl Pts',(-4.24151789226149,-27.205672166438,17.0904886102752));
#2075=CARTESIAN_POINT('Ctrl Pts',(-3.98794903777075,-28.6613021650618,16.9758703668355));
#2076=CARTESIAN_POINT('Ctrl Pts',(-2.34405122024042,-30.7505189403242,16.7467125550671));
#2077=CARTESIAN_POINT('Ctrl Pts',(-0.978754765971974,-31.3540484715026,
16.6320931111307));
#2078=CARTESIAN_POINT('Ctrl Pts',(1.02933886603348,-31.1972354808515,16.460227032321));
#2079=CARTESIAN_POINT('Ctrl Pts',(1.68709482472537,-30.9779968406706,16.4029168679907));
#2080=CARTESIAN_POINT('Ctrl Pts',(2.8240837151474,-30.2508925065775,16.2883402228593));
#2081=CARTESIAN_POINT('Ctrl Pts',(3.30314935266293,-29.7448544918448,16.2310297714992));
#2082=CARTESIAN_POINT('Ctrl Pts',(3.96627580118359,-28.5616040731508,16.116453854622));
#2083=CARTESIAN_POINT('Ctrl Pts',(4.15104388235541,-27.8860791480164,16.0591431204344));
#2084=CARTESIAN_POINT('Ctrl Pts',(4.17802239058402,-26.5231491652539,15.9445679195579));
#2085=CARTESIAN_POINT('Ctrl Pts',(4.02164463287101,-25.836899273559,15.8872569066736));
#2086=CARTESIAN_POINT('Ctrl Pts',(3.39969277305442,-24.6162176795914,15.7726824098211));
#2087=CARTESIAN_POINT('Ctrl Pts',(2.9359020278153,-24.0821430128742,15.7153711223063));
#2088=CARTESIAN_POINT('Ctrl Pts',(1.80627259289743,-23.295059368917,15.6007973177115));
#2089=CARTESIAN_POINT('Ctrl Pts',(1.14217129355625,-23.0415308728188,15.5434857595736));
#2090=CARTESIAN_POINT('Ctrl Pts',(-0.231877317222814,-22.8792861228552,
15.4289126357253));
#2091=CARTESIAN_POINT('Ctrl Pts',(-0.940537550161687,-22.9692999005262,
15.3716008109));
#2092=CARTESIAN_POINT('Ctrl Pts',(-2.23508230276584,-23.4765970744679,15.2570283565139));
#2093=CARTESIAN_POINT('Ctrl Pts',(-2.82042721228882,-23.8921601369938,15.1997162688729));
#2094=CARTESIAN_POINT('Ctrl Pts',(-3.72724254909164,-24.9550994865649,15.0851444728953));
#2095=CARTESIAN_POINT('Ctrl Pts',(-4.04904226418634,-25.6007082903028,15.0278321262568));
#2096=CARTESIAN_POINT('Ctrl Pts',(-4.34898179372202,-26.9722920315092,14.913260977831));
#2097=CARTESIAN_POINT('Ctrl Pts',(-4.32823823833014,-27.696864249156,14.8559483759565));
#2098=CARTESIAN_POINT('Ctrl Pts',(-3.94416673686108,-29.0543767984046,14.741377864454));
#2099=CARTESIAN_POINT('Ctrl Pts',(-3.58247834736109,-29.6866038630478,14.684065011041));
#2100=CARTESIAN_POINT('Ctrl Pts',(-2.59897553580158,-30.7075411869121,14.5694951260371));
#2101=CARTESIAN_POINT('Ctrl Pts',(-1.97893887953295,-31.0963900092535,14.5121820247212));
#2102=CARTESIAN_POINT('Ctrl Pts',(-0.62377058727827,-31.5350735702099,14.3976127560067));
#2103=CARTESIAN_POINT('Ctrl Pts',(0.109859887125028,-31.5858618602476,14.3402994103674));
#2104=CARTESIAN_POINT('Ctrl Pts',(1.51846868411767,-31.3325375520331,14.2257307479178));
#2105=CARTESIAN_POINT('Ctrl Pts',(2.19257064211805,-31.0299670824768,14.1684171614822));
#2106=CARTESIAN_POINT('Ctrl Pts',(3.32065975230898,-30.1381775844584,14.0538490954731));
#2107=CARTESIAN_POINT('Ctrl Pts',(3.77459621319051,-29.5507269915758,13.9965352717156));
#2108=CARTESIAN_POINT('Ctrl Pts',(4.35164549000208,-28.2261503388289,13.8819677925012));
#2109=CARTESIAN_POINT('Ctrl Pts',(4.47554085920862,-27.4906059318028,13.8246537348364));
#2110=CARTESIAN_POINT('Ctrl Pts',(4.35932633846837,-26.043646007592,13.7100868329779));
#2111=CARTESIAN_POINT('Ctrl Pts',(4.1206457473642,-25.3332578752253,13.6527725447744));
#2112=CARTESIAN_POINT('Ctrl Pts',(3.33223129728641,-24.106308328171,13.5382062109767));
#2113=CARTESIAN_POINT('Ctrl Pts',(2.78423731477771,-23.5899834651597,13.4808916955503));
#2114=CARTESIAN_POINT('Ctrl Pts',(1.50450674316234,-22.8764080003258,13.3663259207328));
#2115=CARTESIAN_POINT('Ctrl Pts',(0.774413779611081,-22.6785518889991,13.309011181339));
#2116=CARTESIAN_POINT('Ctrl Pts',(-0.69739330426496,-22.6525522223851,13.1944459565731));
#2117=CARTESIAN_POINT('Ctrl Pts',(-1.43794247925327,-22.8231062186778,13.1371309964266));
#2118=CARTESIAN_POINT('Ctrl Pts',(-2.7541948376007,-23.4972409646481,13.0225663129528));
#2119=CARTESIAN_POINT('Ctrl Pts',(-3.32948087019843,-23.9991290609593,12.9652511352145));
#2120=CARTESIAN_POINT('Ctrl Pts',(-4.17626345911414,-25.2198325829076,12.8506869844455));
#2121=CARTESIAN_POINT('Ctrl Pts',(-4.4481843446811,-25.936961310921,12.7933715922294));
#2122=CARTESIAN_POINT('Ctrl Pts',(-4.62015665278908,-27.4194785452993,12.6788079657272));
#2123=CARTESIAN_POINT('Ctrl Pts',(-4.52137115313415,-28.183579240772,12.621492362104));
#2124=CARTESIAN_POINT('Ctrl Pts',(-3.97152663554103,-29.5783806208201,12.5069292515898));
#2125=CARTESIAN_POINT('Ctrl Pts',(-3.5220951227733,-30.2084906103522,12.4496134395774));
#2126=CARTESIAN_POINT('Ctrl Pts',(-2.37437165907619,-31.183679244984,12.3350508369351));
#2127=CARTESIAN_POINT('Ctrl Pts',(-1.67779038310627,-31.5289988293348,12.277734819509));
#2128=CARTESIAN_POINT('Ctrl Pts',(-0.199197333900588,-31.8492812709321,
12.1631727167557));
#2129=CARTESIAN_POINT('Ctrl Pts',(0.581419535730091,-31.825256919753,12.1058564968451));
#2130=CARTESIAN_POINT('Ctrl Pts',(2.04290487097247,-31.4086885823989,11.9912948861633));
#2131=CARTESIAN_POINT('Ctrl Pts',(2.72301785637377,-31.017689933097,11.9339784666505));
#2132=CARTESIAN_POINT('Ctrl Pts',(3.82034316796606,-29.9565159886648,11.8194173403514));
#2133=CARTESIAN_POINT('Ctrl Pts',(4.23761275995296,-29.2880562452814,11.7621007240815));
#2134=CARTESIAN_POINT('Ctrl Pts',(4.70706068115205,-27.8283747226536,11.6475400746183));
#2135=CARTESIAN_POINT('Ctrl Pts',(4.76009229327592,-27.0386382546772,11.5902232643864));
#2136=CARTESIAN_POINT('Ctrl Pts',(4.48463927434238,-25.5233462828554,11.4756630843606));
#2137=CARTESIAN_POINT('Ctrl Pts',(4.15760185288866,-24.7987006850272,11.4183460829245));
#2138=CARTESIAN_POINT('Ctrl Pts',(3.19600835697949,-23.5869462478655,11.3037863650511));
#2139=CARTESIAN_POINT('Ctrl Pts',(2.56315379146772,-23.099962191222,11.2464691751292));
#2140=CARTESIAN_POINT('Ctrl Pts',(1.13757263913847,-22.4820219779078,11.1319099122695));
#2141=CARTESIAN_POINT('Ctrl Pts',(0.346404347142174,-22.3503795041057,11.0745925365344));
#2142=CARTESIAN_POINT('Ctrl Pts',(-1.76387591167285,-22.5237230755283,10.9191576492385));
#2143=CARTESIAN_POINT('Ctrl Pts',(-3.04213419140331,-23.2249589278969,10.8209586709532));
#2144=CARTESIAN_POINT('Ctrl Pts',(-4.26287386638314,-24.8351878142477,10.6736877485838));
#2145=CARTESIAN_POINT('Ctrl Pts',(-4.55417709738229,-25.4602183705301,10.6246080237907));
#2146=CARTESIAN_POINT('Ctrl Pts',(-4.78298015330037,-26.4482305165422,10.5509677380958));
#2147=CARTESIAN_POINT('Ctrl Pts',(-4.82497450026767,-26.7858033043513,10.5264227857054));
#2148=CARTESIAN_POINT('Ctrl Pts',(-4.83612470074125,-27.4630368812996,10.4773448839533));
#2149=CARTESIAN_POINT('Ctrl Pts',(-4.81152195248019,-27.8040996825675,10.4527957512917));
#2150=CARTESIAN_POINT('Ctrl Pts',(-4.7966595069499,-28.1445096413087,10.4282516293878));
#2151=CARTESIAN_POINT('',(-3.5,-27.1131792176833,21.5024833879649));
#2152=CARTESIAN_POINT('',(-3.5,-27.2127225901214,22.4975166120351));
#2153=CARTESIAN_POINT('Origin',(-3.5,-27.1629509039024,22.));
#2154=CARTESIAN_POINT('',(-4.8706353805564,-27.2129260271478,11.4970938327966));
#2155=CARTESIAN_POINT('Ctrl Pts',(-3.5,-27.2127225901214,22.4975166120351));
#2156=CARTESIAN_POINT('Ctrl Pts',(-3.49927785868713,-27.7853287709716,22.4402329481162));
#2157=CARTESIAN_POINT('Ctrl Pts',(-3.35446180200001,-28.3588230843844,22.3829524737063));
#2158=CARTESIAN_POINT('Ctrl Pts',(-3.08233709444319,-28.8665899867746,22.3256713790777));
#2159=CARTESIAN_POINT('Ctrl Pts',(-2.53808767932955,-29.8821237915549,22.2111091898206));
#2160=CARTESIAN_POINT('Ctrl Pts',(-1.46145231937318,-30.6017446798008,22.0965431657326));
#2161=CARTESIAN_POINT('Ctrl Pts',(-0.300724866977927,-30.7149783442486,
21.9819785454515));
#2162=CARTESIAN_POINT('Ctrl Pts',(0.860002585417323,-30.8282120086964,21.8674139251703));
#2163=CARTESIAN_POINT('Ctrl Pts',(2.07107291079633,-30.3270227433741,21.752849624791));
#2164=CARTESIAN_POINT('Ctrl Pts',(2.81914416447585,-29.4140703534682,21.6382826642361));
#2165=CARTESIAN_POINT('Ctrl Pts',(3.56721541815537,-28.5011179635623,21.5237157036811));
#2166=CARTESIAN_POINT('Ctrl Pts',(3.82659931701312,-27.20036017698,21.4091530749885));
#2167=CARTESIAN_POINT('Ctrl Pts',(3.47920099433721,-26.05765356589,21.2945838607121));
#2168=CARTESIAN_POINT('Ctrl Pts',(3.13180267166131,-24.9149469548,21.1800146464357));
#2169=CARTESIAN_POINT('Ctrl Pts',(2.18342706770339,-23.9653744387647,21.0654536391327));
#2170=CARTESIAN_POINT('Ctrl Pts',(1.02690098156517,-23.6151296959839,20.9508822537436));
#2171=CARTESIAN_POINT('Ctrl Pts',(-0.129625104573071,-23.2648849532031,
20.8363108683544));
#2172=CARTESIAN_POINT('Ctrl Pts',(-1.46147591168062,-23.5287326354126,20.7217514337973));
#2173=CARTESIAN_POINT('Ctrl Pts',(-2.40619046989316,-24.3045463380016,20.6071779561761));
#2174=CARTESIAN_POINT('Ctrl Pts',(-3.35090502810569,-25.0803600405907,20.4926044785548));
#2175=CARTESIAN_POINT('Ctrl Pts',(-3.87764741849126,-26.3487475764667,20.3780465697071));
#2176=CARTESIAN_POINT('Ctrl Pts',(-3.75622295306029,-27.5792619376628,20.2634710752061));
#2177=CARTESIAN_POINT('Ctrl Pts',(-3.63479848762931,-28.8097762988588,20.148895580705));
#2178=CARTESIAN_POINT('Ctrl Pts',(-2.86427039073957,-29.9655693350743,20.0343391520621));
#2179=CARTESIAN_POINT('Ctrl Pts',(-1.76136567891206,-30.5550064110035,19.9197617127236));
#2180=CARTESIAN_POINT('Ctrl Pts',(-0.658460967084561,-31.1444434869326,
19.8051842733852));
#2181=CARTESIAN_POINT('Ctrl Pts',(0.746302062294618,-31.1460905834951,19.6906292809279));
#2182=CARTESIAN_POINT('Ctrl Pts',(1.86159846889728,-30.5500516030908,19.5760499656309));
#2183=CARTESIAN_POINT('Ctrl Pts',(2.97689487550167,-29.9540126226856,19.4614706503338));
#2184=CARTESIAN_POINT('Ctrl Pts',(3.76757285952208,-28.7739850439139,19.3469170514958));
#2185=CARTESIAN_POINT('Ctrl Pts',(3.89313817407229,-27.5015528155106,19.232335926138));
#2186=CARTESIAN_POINT('Ctrl Pts',(4.0187034886225,-26.2291205871072,19.1177548007802));
#2187=CARTESIAN_POINT('Ctrl Pts',(3.47099870281935,-24.9015607577697,19.0032025543658));
#2188=CARTESIAN_POINT('Ctrl Pts',(2.47201536773451,-24.0812116030623,18.8886196820384));
#2189=CARTESIAN_POINT('Ctrl Pts',(1.47303203265275,-23.2608624483575,18.7740368097113));
#2190=CARTESIAN_POINT('Ctrl Pts',(0.0495881203952367,-22.9754752873616,
18.6594858758451));
#2191=CARTESIAN_POINT('Ctrl Pts',(-1.20098450905675,-23.3542715475307,18.5449013169653));
#2192=CARTESIAN_POINT('Ctrl Pts',(-2.45155713850874,-23.7330678076998,18.4303167580854));
#2193=CARTESIAN_POINT('Ctrl Pts',(-3.49087258075458,-24.7690158719264,18.3157670982032));
#2194=CARTESIAN_POINT('Ctrl Pts',(-3.87490628882521,-26.0326624463887,18.2011809106308));
#2195=CARTESIAN_POINT('Ctrl Pts',(-4.25893999689644,-27.296309020853,18.0865947230583));
#2196=CARTESIAN_POINT('Ctrl Pts',(-3.97210868158914,-28.7514045749302,17.9720462998272));
#2197=CARTESIAN_POINT('Ctrl Pts',(-3.12599127827046,-29.7836951551393,17.8574585390487));
#2198=CARTESIAN_POINT('Ctrl Pts',(-2.27987387495177,-30.8159857353485,17.7428707782702));
#2199=CARTESIAN_POINT('Ctrl Pts',(-0.896249322735716,-31.3920519629118,
17.6283235555406));
#2200=CARTESIAN_POINT('Ctrl Pts',(0.446119482153031,-31.260803072352,17.5137342747424));
#2201=CARTESIAN_POINT('Ctrl Pts',(1.11730388459739,-31.1951786270721,17.4564396343434));
#2202=CARTESIAN_POINT('Ctrl Pts',(1.77294326754582,-30.9607539401843,17.3991664653485));
#2203=CARTESIAN_POINT('Ctrl Pts',(2.33687415954374,-30.584564367571,17.341871454575));
#2204=CARTESIAN_POINT('Ctrl Pts',(2.90080505154166,-30.2083747949576,17.2845764438015));
#2205=CARTESIAN_POINT('Ctrl Pts',(3.37097187102429,-29.6899170424932,17.2273035618313));
#2206=CARTESIAN_POINT('Ctrl Pts',(3.69266231980076,-29.0892360048921,17.1700081869394));
#2207=CARTESIAN_POINT('Ctrl Pts',(4.01435276857722,-28.4885549672909,17.1127128120475));
#2208=CARTESIAN_POINT('Ctrl Pts',(4.1855172562512,-27.8061906781911,17.0554402129015));
#2209=CARTESIAN_POINT('Ctrl Pts',(4.18609703346223,-27.1212876511694,16.9981444800039));
#2210=CARTESIAN_POINT('Ctrl Pts',(4.18667681067326,-26.4363846241478,16.9408487471063));
#2211=CARTESIAN_POINT('Ctrl Pts',(4.01512628257138,-25.7503981626563,16.8835764266556));
#2212=CARTESIAN_POINT('Ctrl Pts',(3.69115303545709,-25.1429871857214,16.8262803417527));
#2213=CARTESIAN_POINT('Ctrl Pts',(3.36717978834281,-24.5355762087865,16.7689842568497));
#2214=CARTESIAN_POINT('Ctrl Pts',(2.8901192769073,-24.0087606262116,16.7117122110268));
#2215=CARTESIAN_POINT('Ctrl Pts',(2.31517235890273,-23.6238173905489,16.6544157799911));
#2216=CARTESIAN_POINT('Ctrl Pts',(1.74022544089816,-23.2388741548863,16.5971193489555));
#2217=CARTESIAN_POINT('Ctrl Pts',(1.06777289997686,-22.997899001297,16.5398475737628));
#2218=CARTESIAN_POINT('Ctrl Pts',(0.375768986061547,-22.9290618458416,16.4825508023506));
#2219=CARTESIAN_POINT('Ctrl Pts',(-0.316234927853762,-22.8602246903861,
16.4252540309383));
#2220=CARTESIAN_POINT('Ctrl Pts',(-1.02645305770396,-22.9651883959601,16.3679825224341));
#2221=CARTESIAN_POINT('Ctrl Pts',(-1.67244586303799,-23.2319995764873,16.310685416293));
#2222=CARTESIAN_POINT('Ctrl Pts',(-2.31843866837203,-23.4988107570144,16.253388310152));
#2223=CARTESIAN_POINT('Ctrl Pts',(-2.89823397310667,-23.9282941364198,16.196117064454));
#2224=CARTESIAN_POINT('Ctrl Pts',(-3.34442253908102,-24.4708084993747,16.1388196291159));
#2225=CARTESIAN_POINT('Ctrl Pts',(-3.79061110505536,-25.0133228623296,16.0815221937778));
#2226=CARTESIAN_POINT('Ctrl Pts',(-4.10106225113868,-25.6686515734845,16.0242512070742));
#2227=CARTESIAN_POINT('Ctrl Pts',(-4.23954028441954,-26.3608692289885,15.9669534479561));
#2228=CARTESIAN_POINT('Ctrl Pts',(-4.37801831770041,-27.0530868844925,15.909655688838));
#2229=CARTESIAN_POINT('Ctrl Pts',(-4.34275064929299,-27.7809842375283,15.8523849573772));
#2230=CARTESIAN_POINT('Ctrl Pts',(-4.13758070760249,-28.4601059771739,15.7950868797947));
#2231=CARTESIAN_POINT('Ctrl Pts',(-3.93241076591198,-29.1392277168195,15.7377888022123));
#2232=CARTESIAN_POINT('Ctrl Pts',(-3.55635559774948,-29.7676616996119,15.6805183222975));
#2233=CARTESIAN_POINT('Ctrl Pts',(-3.05282021676699,-30.2723764411732,15.623219931461));
#2234=CARTESIAN_POINT('Ctrl Pts',(-2.5492848357845,-30.7770911827345,15.5659215406245));
#2235=CARTESIAN_POINT('Ctrl Pts',(-1.91831750124282,-31.1559328914483,15.508651308613));
#2236=CARTESIAN_POINT('Ctrl Pts',(-1.2329741624294,-31.3647327437876,15.451352609636));
#2237=CARTESIAN_POINT('Ctrl Pts',(-0.547630823615978,-31.5735325961269,
15.3940539106591));
#2238=CARTESIAN_POINT('Ctrl Pts',(0.191016654419482,-31.6104167135758,15.3367839229662));
#2239=CARTESIAN_POINT('Ctrl Pts',(0.89730499163605,-31.4708391887802,15.2794849208574));
#2240=CARTESIAN_POINT('Ctrl Pts',(1.60359332885263,-31.3312616639846,15.2221859187487));
#2241=CARTESIAN_POINT('Ctrl Pts',(2.27568288412789,-31.0140842055001,15.1649161718489));
#2242=CARTESIAN_POINT('Ctrl Pts',(2.83550405741099,-30.5558465016054,15.1076168715224));
#2243=CARTESIAN_POINT('Ctrl Pts',(3.39532523069409,-30.0976087977106,15.0503175711959));
#2244=CARTESIAN_POINT('Ctrl Pts',(3.84071356306252,-29.4981872635055,14.9930480616187));
#2245=CARTESIAN_POINT('Ctrl Pts',(4.11978778472223,-28.8269348794253,14.9357484678916));
#2246=CARTESIAN_POINT('Ctrl Pts',(4.39886200638193,-28.1556824953451,14.8784488741644));
#2247=CARTESIAN_POINT('Ctrl Pts',(4.50965629588013,-27.4135246591517,14.821179598491));
#2248=CARTESIAN_POINT('Ctrl Pts',(4.43903740169352,-26.6864895804728,14.7638797160928));
#2249=CARTESIAN_POINT('Ctrl Pts',(4.36841850750692,-25.9594545017938,14.7065798336947));
#2250=CARTESIAN_POINT('Ctrl Pts',(4.11509669119356,-25.2492967556584,14.649310788563));
#2251=CARTESIAN_POINT('Ctrl Pts',(3.70817268294378,-24.6384703175102,14.5920106221244));
#2252=CARTESIAN_POINT('Ctrl Pts',(3.301248674694,-24.027643879362,14.5347104556859));
#2253=CARTESIAN_POINT('Ctrl Pts',(2.7404244263817,-23.5183108657722,14.4774416377848));
#2254=CARTESIAN_POINT('Ctrl Pts',(2.09053277799751,-23.1697564447712,14.4201411918584));
#2255=CARTESIAN_POINT('Ctrl Pts',(1.44064112961332,-22.8212020237703,14.3628407459321));
#2256=CARTESIAN_POINT('Ctrl Pts',(0.702452411780131,-22.6354736977066,14.3055721519949));
#2257=CARTESIAN_POINT('Ctrl Pts',(-0.0385102376731089,-22.6344044972146,
14.2482714310439));
#2258=CARTESIAN_POINT('Ctrl Pts',(-0.779472887126349,-22.6333352967227,
14.190970710093));
#2259=CARTESIAN_POINT('Ctrl Pts',(-1.52155253015144,-22.8183614641083,14.1337023369077));
#2260=CARTESIAN_POINT('Ctrl Pts',(-2.17862881446343,-23.1683317441552,14.0764013453103));
#2261=CARTESIAN_POINT('Ctrl Pts',(-2.83570509877542,-23.5183020242021,14.0191003537129));
#2262=CARTESIAN_POINT('Ctrl Pts',(-3.40563177267264,-24.0336906113065,13.9618321981179));
#2263=CARTESIAN_POINT('Ctrl Pts',(-3.82211503358254,-24.6549763574959,13.90453094017));
#2264=CARTESIAN_POINT('Ctrl Pts',(-4.23859829449244,-25.2762621036854,13.8472296822221));
#2265=CARTESIAN_POINT('Ctrl Pts',(-4.49952012993745,-26.0028377560707,13.7899617411021));
#2266=CARTESIAN_POINT('Ctrl Pts',(-4.5743242236405,-26.7505734520165,13.7326602210217));
#2267=CARTESIAN_POINT('Ctrl Pts',(-4.64912831734354,-27.4983091479623,13.6753587009413));
#2268=CARTESIAN_POINT('Ctrl Pts',(-4.53623796107103,-28.2656580682613,13.6180909712297));
#2269=CARTESIAN_POINT('Ctrl Pts',(-4.248414634479,-28.9636095611531,13.5607891931531));
#2270=CARTESIAN_POINT('Ctrl Pts',(-3.96059130788698,-29.6615610540449,13.5034874150766));
#2271=CARTESIAN_POINT('Ctrl Pts',(-3.49718400748527,-30.2879987021829,13.4462198937543));
#2272=CARTESIAN_POINT('Ctrl Pts',(-2.91164546032268,-30.7700999199001,13.3889178617438));
#2273=CARTESIAN_POINT('Ctrl Pts',(-2.32610691316009,-31.2522011376172,13.3316158297333));
#2274=CARTESIAN_POINT('Ctrl Pts',(-1.61887397941474,-31.5877894623157,13.2743485138248));
#2275=CARTESIAN_POINT('Ctrl Pts',(-0.87178599679515,-31.7376531660138,13.2170462318676));
#2276=CARTESIAN_POINT('Ctrl Pts',(-0.124698014175558,-31.8875168697119,
13.1597439499104));
#2277=CARTESIAN_POINT('Ctrl Pts',(0.660820605236809,-31.8499459440715,13.1024768364861));
#2278=CARTESIAN_POINT('Ctrl Pts',(1.3936961112827,-31.6289484960591,13.0451743084958));
#2279=CARTESIAN_POINT('Ctrl Pts',(2.12657161732859,-31.4079510480467,12.9878717805055));
#2280=CARTESIAN_POINT('Ctrl Pts',(2.8047317654823,-31.0026997016065,12.9306048666813));
#2281=CARTESIAN_POINT('Ctrl Pts',(3.34938652219548,-30.4598658812891,12.873302096499));
#2282=CARTESIAN_POINT('Ctrl Pts',(3.89404127890866,-29.9170320609718,12.8159993263168));
#2283=CARTESIAN_POINT('Ctrl Pts',(4.30296864843085,-29.2368757228388,12.7587326092554));
#2284=CARTESIAN_POINT('Ctrl Pts',(4.5284622492945,-28.4980488411566,12.7014296006501));
#2285=CARTESIAN_POINT('Ctrl Pts',(4.75395585015816,-27.7592219594744,12.6441265920449));
#2286=CARTESIAN_POINT('Ctrl Pts',(4.79418068964257,-26.9630145561609,12.5868600689426));
#2287=CARTESIAN_POINT('Ctrl Pts',(4.64411039827566,-26.2016928243926,12.5295568256265));
#2288=CARTESIAN_POINT('Ctrl Pts',(4.49404010690874,-25.4403710926243,12.4722535823103));
#2289=CARTESIAN_POINT('Ctrl Pts',(4.15267254437464,-24.7159484861244,12.4149872504092));
#2290=CARTESIAN_POINT('Ctrl Pts',(3.65923754232643,-24.112543732137,12.3576837760122));
#2291=CARTESIAN_POINT('Ctrl Pts',(3.16580254027822,-23.5091389781496,12.3003803016153));
#2292=CARTESIAN_POINT('Ctrl Pts',(2.52037754996714,-23.0290058774741,12.2431141582024));
#2293=CARTESIAN_POINT('Ctrl Pts',(1.79754041616261,-22.7280913019251,12.1858104563006));
#2294=CARTESIAN_POINT('Ctrl Pts',(1.07470328235808,-22.427176726376,12.1285067543989));
#2295=CARTESIAN_POINT('Ctrl Pts',(0.275598076802497,-22.3074311776151,12.0712407967975));
#2296=CARTESIAN_POINT('Ctrl Pts',(-0.507222361580798,-22.3831090971102,
12.0139368708962));
#2297=CARTESIAN_POINT('Ctrl Pts',(-1.84868379116738,-22.5127927449768,11.9157393755432));
#2298=CARTESIAN_POINT('Ctrl Pts',(-3.12606319175256,-23.2393767520925,11.8175853786087));
#2299=CARTESIAN_POINT('Ctrl Pts',(-3.93010953926081,-24.3333832686755,11.7194130182977));
#2300=CARTESIAN_POINT('Ctrl Pts',(-4.33213271301493,-24.8803865269671,11.6703268381421));
#2301=CARTESIAN_POINT('Ctrl Pts',(-4.61678084393395,-25.5145917668544,11.6212300753262));
#2302=CARTESIAN_POINT('Ctrl Pts',(-4.76059861401404,-26.1806970253915,11.5721471115128));
#2303=CARTESIAN_POINT('Ctrl Pts',(-4.8325074990541,-26.51374965466,11.5476056296061));
#2304=CARTESIAN_POINT('Ctrl Pts',(-4.86981537831802,-26.8545716453141,11.5230623381901));
#2305=CARTESIAN_POINT('Ctrl Pts',(-4.87066042040856,-27.195983624313,11.498513045262));
#2306=CARTESIAN_POINT('Ctrl Pts',(-4.8706744167737,-27.2016384038463,11.4981064372701));
#2307=CARTESIAN_POINT('Ctrl Pts',(-4.87068176644947,-27.207292836302,11.4976998360475));
#2308=CARTESIAN_POINT('Ctrl Pts',(-4.87064344737806,-27.2129433732647,11.4972950499307));
#2309=CARTESIAN_POINT('',(-4.85063011250931,-27.2127229045708,11.4975165893541));
#2310=CARTESIAN_POINT('Origin',(-4.85063016993195,-27.162950903902,11.));
#2311=CARTESIAN_POINT('',(-4.83035516948488,-27.1129735823552,10.5029173190626));
#2312=CARTESIAN_POINT('Origin',(-4.85063016993195,-27.162950903902,11.));
#2313=CARTESIAN_POINT('Ctrl Pts',(-3.5,-27.1131792176833,21.5024833879649));
#2314=CARTESIAN_POINT('Ctrl Pts',(-3.51479119919922,-27.6859453885664,21.4451837185487));
#2315=CARTESIAN_POINT('Ctrl Pts',(-3.3869826954375,-28.2639018202575,21.3878808596267));
#2316=CARTESIAN_POINT('Ctrl Pts',(-3.1283351768432,-28.7789853117735,21.3305786209223));
#2317=CARTESIAN_POINT('Ctrl Pts',(-2.6110401396546,-29.8091522948055,21.2159741435134));
#2318=CARTESIAN_POINT('Ctrl Pts',(-1.55527081107218,-30.5598658867912,21.1013735009366));
#2319=CARTESIAN_POINT('Ctrl Pts',(-0.397806200350788,-30.7032284111832,
20.9867714545485));
#2320=CARTESIAN_POINT('Ctrl Pts',(0.7596584103706,-30.8465909355753,20.8721694081605));
#2321=CARTESIAN_POINT('Ctrl Pts',(1.98433800521209,-30.3798149635844,20.7575670418755));
#2322=CARTESIAN_POINT('Ctrl Pts',(2.75506201531091,-29.4864642417935,20.6429673357639));
#2323=CARTESIAN_POINT('Ctrl Pts',(3.52578602540974,-28.5931135200026,20.5283676296524));
#2324=CARTESIAN_POINT('Ctrl Pts',(3.8208190800791,-27.3005795704328,20.4137635916772));
#2325=CARTESIAN_POINT('Ctrl Pts',(3.50210971259614,-26.150490791734,20.2991661392879));
#2326=CARTESIAN_POINT('Ctrl Pts',(3.18340034511317,-25.0004020130352,20.1845686868986));
#2327=CARTESIAN_POINT('Ctrl Pts',(2.26172892311522,-24.0264166801336,20.0699630275308));
#2328=CARTESIAN_POINT('Ctrl Pts',(1.115360671301,-23.6486818743709,19.9553677462564));
#2329=CARTESIAN_POINT('Ctrl Pts',(-0.0310075805132359,-23.2709470686081,
19.840772464982));
#2330=CARTESIAN_POINT('Ctrl Pts',(-1.36774615552683,-23.4993356660845,19.7261652328664));
#2331=CARTESIAN_POINT('Ctrl Pts',(-2.32909807553772,-24.2513896825192,19.6115720438239));
#2332=CARTESIAN_POINT('Ctrl Pts',(-3.29044999554861,-25.003443698954,19.4969788547815));
#2333=CARTESIAN_POINT('Ctrl Pts',(-3.84882652597964,-26.255889878113,19.3823700969656));
#2334=CARTESIAN_POINT('Ctrl Pts',(-3.75612153097279,-27.4865412208768,19.267778924794));
#2335=CARTESIAN_POINT('Ctrl Pts',(-3.66341653596594,-28.7171925636406,19.1531877526223));
#2336=CARTESIAN_POINT('Ctrl Pts',(-2.92366288113256,-29.8898022514147,19.0385775146034));
#2337=CARTESIAN_POINT('Ctrl Pts',(-1.83685647329081,-30.5026955599585,18.9239882872764));
#2338=CARTESIAN_POINT('Ctrl Pts',(-0.750050065449064,-31.1155888685022,
18.8093990599493));
#2339=CARTESIAN_POINT('Ctrl Pts',(0.651110587682155,-31.1517796318851,18.6947873857344));
#2340=CARTESIAN_POINT('Ctrl Pts',(1.77641634922847,-30.5820972095669,18.5802000343691));
#2341=CARTESIAN_POINT('Ctrl Pts',(2.90172211077653,-30.0124147872479,18.4656126830036));
#2342=CARTESIAN_POINT('Ctrl Pts',(3.71853772096226,-28.8547645355866,18.3509996151738));
#2343=CARTESIAN_POINT('Ctrl Pts',(3.87123003180434,-27.5890725130726,18.236414073862));
#2344=CARTESIAN_POINT('Ctrl Pts',(4.02392234264641,-26.3233804905586,18.1218285325501));
#2345=CARTESIAN_POINT('Ctrl Pts',(3.50918503257104,-24.9871031169595,18.0072141122992));
#2346=CARTESIAN_POINT('Ctrl Pts',(2.53103277431928,-24.1484584049633,17.8926303179616));
#2347=CARTESIAN_POINT('Ctrl Pts',(1.55288051607053,-23.3098136929698,17.7780465236243));
#2348=CARTESIAN_POINT('Ctrl Pts',(0.140896517323788,-22.9926200323223,17.6634307908027));
#2349=CARTESIAN_POINT('Ctrl Pts',(-1.1128065626084,-23.3440833092083,17.5488486830347));
#2350=CARTESIAN_POINT('Ctrl Pts',(-2.36650964254058,-23.6955465860942,17.4342665752667));
#2351=CARTESIAN_POINT('Ctrl Pts',(-3.42532249325332,-24.7042160076948,17.319649568463));
#2352=CARTESIAN_POINT('Ctrl Pts',(-3.83342019275709,-25.9549440870654,17.2050690893692));
#2353=CARTESIAN_POINT('Ctrl Pts',(-4.24151789226148,-27.205672166438,17.0904886102752));
#2354=CARTESIAN_POINT('Ctrl Pts',(-3.98794903777076,-28.6613021650618,16.9758703668355));
#2355=CARTESIAN_POINT('Ctrl Pts',(-3.16600012900559,-29.705910552693,16.8612914609513));
#2356=CARTESIAN_POINT('Ctrl Pts',(-2.34405122024042,-30.7505189403242,16.7467125550671));
#2357=CARTESIAN_POINT('Ctrl Pts',(-0.978754765971974,-31.3540484715026,
16.6320931111307));
#2358=CARTESIAN_POINT('Ctrl Pts',(0.359974322031668,-31.2495064777352,16.5175157252576));
#2359=CARTESIAN_POINT('Ctrl Pts',(1.02933886603347,-31.1972354808515,16.460227032321));
#2360=CARTESIAN_POINT('Ctrl Pts',(1.68709482472536,-30.9779968406706,16.4029168679907));
#2361=CARTESIAN_POINT('Ctrl Pts',(2.25558926993638,-30.6144446736241,16.345628545425));
#2362=CARTESIAN_POINT('Ctrl Pts',(2.82408371514739,-30.2508925065775,16.2883402228593));
#2363=CARTESIAN_POINT('Ctrl Pts',(3.30314935266293,-29.7448544918448,16.2310297714992));
#2364=CARTESIAN_POINT('Ctrl Pts',(3.63471257692326,-29.1532292824978,16.1737418130606));
#2365=CARTESIAN_POINT('Ctrl Pts',(3.96627580118359,-28.5616040731508,16.116453854622));
#2366=CARTESIAN_POINT('Ctrl Pts',(4.15104388235541,-27.8860791480164,16.0591431204344));
#2367=CARTESIAN_POINT('Ctrl Pts',(4.16453313646972,-27.2046141566351,16.0018555199961));
#2368=CARTESIAN_POINT('Ctrl Pts',(4.17802239058402,-26.5231491652539,15.9445679195579));
#2369=CARTESIAN_POINT('Ctrl Pts',(4.02164463287101,-25.836899273559,15.8872569066736));
#2370=CARTESIAN_POINT('Ctrl Pts',(3.71066870296272,-25.2265584765752,15.8299696582473));
#2371=CARTESIAN_POINT('Ctrl Pts',(3.39969277305442,-24.6162176795914,15.7726824098211));
#2372=CARTESIAN_POINT('Ctrl Pts',(2.9359020278153,-24.0821430128742,15.7153711223063));
#2373=CARTESIAN_POINT('Ctrl Pts',(2.37108731035637,-23.6886011908956,15.6580842200089));
#2374=CARTESIAN_POINT('Ctrl Pts',(1.80627259289744,-23.295059368917,15.6007973177115));
#2375=CARTESIAN_POINT('Ctrl Pts',(1.14217129355625,-23.0415308728188,15.5434857595736));
#2376=CARTESIAN_POINT('Ctrl Pts',(0.455146988166719,-22.960408497837,15.4861991976495));
#2377=CARTESIAN_POINT('Ctrl Pts',(-0.231877317222808,-22.8792861228552,
15.4289126357253));
#2378=CARTESIAN_POINT('Ctrl Pts',(-0.940537550161691,-22.9692999005262,
15.3716008109));
#2379=CARTESIAN_POINT('Ctrl Pts',(-1.58780992646376,-23.222948487497,15.314314583707));
#2380=CARTESIAN_POINT('Ctrl Pts',(-2.23508230276583,-23.4765970744678,15.2570283565139));
#2381=CARTESIAN_POINT('Ctrl Pts',(-2.82042721228882,-23.8921601369938,15.1997162688729));
#2382=CARTESIAN_POINT('Ctrl Pts',(-3.27383488069023,-24.4236298117793,15.1424303708841));
#2383=CARTESIAN_POINT('Ctrl Pts',(-3.72724254909164,-24.9550994865649,15.0851444728953));
#2384=CARTESIAN_POINT('Ctrl Pts',(-4.04904226418634,-25.6007082903028,15.0278321262568));
#2385=CARTESIAN_POINT('Ctrl Pts',(-4.19901202895418,-26.286500160906,14.9705465520439));
#2386=CARTESIAN_POINT('Ctrl Pts',(-4.34898179372202,-26.9722920315092,14.913260977831));
#2387=CARTESIAN_POINT('Ctrl Pts',(-4.32823823833014,-27.696864249156,14.8559483759565));
#2388=CARTESIAN_POINT('Ctrl Pts',(-4.13620248759561,-28.3756205237803,14.7986631202052));
#2389=CARTESIAN_POINT('Ctrl Pts',(-3.94416673686108,-29.0543767984046,14.741377864454));
#2390=CARTESIAN_POINT('Ctrl Pts',(-3.58247834736109,-29.6866038630478,14.684065011041));
#2391=CARTESIAN_POINT('Ctrl Pts',(-3.09072694158133,-30.1970725249799,14.6267800685391));
#2392=CARTESIAN_POINT('Ctrl Pts',(-2.59897553580158,-30.7075411869121,14.5694951260371));
#2393=CARTESIAN_POINT('Ctrl Pts',(-1.97893887953295,-31.0963900092535,14.5121820247212));
#2394=CARTESIAN_POINT('Ctrl Pts',(-1.30135473340561,-31.3157317897317,14.454897390364));
#2395=CARTESIAN_POINT('Ctrl Pts',(-0.62377058727827,-31.5350735702099,14.3976127560067));
#2396=CARTESIAN_POINT('Ctrl Pts',(0.109859887125027,-31.5858618602476,14.3402994103674));
#2397=CARTESIAN_POINT('Ctrl Pts',(0.814164285621345,-31.4591997061404,14.2830150791426));
#2398=CARTESIAN_POINT('Ctrl Pts',(1.51846868411766,-31.3325375520331,14.2257307479178));
#2399=CARTESIAN_POINT('Ctrl Pts',(2.19257064211805,-31.0299670824768,14.1684171614822));
#2400=CARTESIAN_POINT('Ctrl Pts',(2.75661519721351,-30.5840723334676,14.1111331284776));
#2401=CARTESIAN_POINT('Ctrl Pts',(3.32065975230897,-30.1381775844583,14.0538490954731));
#2402=CARTESIAN_POINT('Ctrl Pts',(3.77459621319051,-29.5507269915758,13.9965352717156));
#2403=CARTESIAN_POINT('Ctrl Pts',(4.0631208515963,-28.8884386652024,13.9392515321084));
#2404=CARTESIAN_POINT('Ctrl Pts',(4.35164549000209,-28.2261503388289,13.8819677925012));
#2405=CARTESIAN_POINT('Ctrl Pts',(4.47554085920862,-27.4906059318028,13.8246537348364));
#2406=CARTESIAN_POINT('Ctrl Pts',(4.4174335988385,-26.7671259696974,13.7673702839072));
#2407=CARTESIAN_POINT('Ctrl Pts',(4.35932633846837,-26.043646007592,13.7100868329779));
#2408=CARTESIAN_POINT('Ctrl Pts',(4.1206457473642,-25.3332578752253,13.6527725447744));
#2409=CARTESIAN_POINT('Ctrl Pts',(3.7264385223253,-24.7197831016981,13.5954893778756));
#2410=CARTESIAN_POINT('Ctrl Pts',(3.33223129728641,-24.106308328171,13.5382062109767));
#2411=CARTESIAN_POINT('Ctrl Pts',(2.78423731477771,-23.5899834651597,13.4808916955503));
#2412=CARTESIAN_POINT('Ctrl Pts',(2.14437202897003,-23.2331957327427,13.4236088081416));
#2413=CARTESIAN_POINT('Ctrl Pts',(1.50450674316235,-22.8764080003258,13.3663259207328));
#2414=CARTESIAN_POINT('Ctrl Pts',(0.774413779611077,-22.6785518889991,13.309011181339));
#2415=CARTESIAN_POINT('Ctrl Pts',(0.0385102376730604,-22.6655520556921,
13.2517285689561));
#2416=CARTESIAN_POINT('Ctrl Pts',(-0.697393304264956,-22.6525522223851,
13.1944459565731));
#2417=CARTESIAN_POINT('Ctrl Pts',(-1.43794247925328,-22.8231062186778,13.1371309964266));
#2418=CARTESIAN_POINT('Ctrl Pts',(-2.09606865842699,-23.160173591663,13.0798486546897));
#2419=CARTESIAN_POINT('Ctrl Pts',(-2.7541948376007,-23.4972409646481,13.0225663129528));
#2420=CARTESIAN_POINT('Ctrl Pts',(-3.32948087019844,-23.9991290609593,12.9652511352145));
#2421=CARTESIAN_POINT('Ctrl Pts',(-3.75287216465629,-24.6094808219334,12.90796905983));
#2422=CARTESIAN_POINT('Ctrl Pts',(-4.17626345911414,-25.2198325829076,12.8506869844455));
#2423=CARTESIAN_POINT('Ctrl Pts',(-4.4481843446811,-25.936961310921,12.7933715922294));
#2424=CARTESIAN_POINT('Ctrl Pts',(-4.53417049873509,-26.6782199281101,12.7360897789783));
#2425=CARTESIAN_POINT('Ctrl Pts',(-4.62015665278908,-27.4194785452993,12.6788079657272));
#2426=CARTESIAN_POINT('Ctrl Pts',(-4.52137115313414,-28.183579240772,12.621492362104));
#2427=CARTESIAN_POINT('Ctrl Pts',(-4.24644889433759,-28.880979930796,12.5642108068469));
#2428=CARTESIAN_POINT('Ctrl Pts',(-3.97152663554103,-29.5783806208201,12.5069292515898));
#2429=CARTESIAN_POINT('Ctrl Pts',(-3.52209512277329,-30.2084906103522,12.4496134395774));
#2430=CARTESIAN_POINT('Ctrl Pts',(-2.94823339092475,-30.6960849276681,12.3923321382562));
#2431=CARTESIAN_POINT('Ctrl Pts',(-2.3743716590762,-31.183679244984,12.335050836935));
#2432=CARTESIAN_POINT('Ctrl Pts',(-1.67779038310626,-31.5289988293348,12.277734819509));
#2433=CARTESIAN_POINT('Ctrl Pts',(-0.938493858503428,-31.6891400501335,
12.2204537681324));
#2434=CARTESIAN_POINT('Ctrl Pts',(-0.199197333900594,-31.8492812709321,
12.1631727167557));
#2435=CARTESIAN_POINT('Ctrl Pts',(0.581419535730098,-31.8252569197531,12.1058564968451));
#2436=CARTESIAN_POINT('Ctrl Pts',(1.31216220335129,-31.616972751076,12.0485756915042));
#2437=CARTESIAN_POINT('Ctrl Pts',(2.04290487097248,-31.408688582399,11.9912948861633));
#2438=CARTESIAN_POINT('Ctrl Pts',(2.72301785637377,-31.017689933097,11.9339784666505));
#2439=CARTESIAN_POINT('Ctrl Pts',(3.27168051216991,-30.4871029608809,11.876697903501));
#2440=CARTESIAN_POINT('Ctrl Pts',(3.82034316796606,-29.9565159886648,11.8194173403514));
#2441=CARTESIAN_POINT('Ctrl Pts',(4.23761275995297,-29.2880562452814,11.7621007240815));
#2442=CARTESIAN_POINT('Ctrl Pts',(4.47233672055251,-28.5582154839675,11.7048203993499));
#2443=CARTESIAN_POINT('Ctrl Pts',(4.70706068115206,-27.8283747226536,11.6475400746183));
#2444=CARTESIAN_POINT('Ctrl Pts',(4.76009229327592,-27.0386382546772,11.5902232643864));
#2445=CARTESIAN_POINT('Ctrl Pts',(4.62236578380915,-26.2809922687663,11.5329431743735));
#2446=CARTESIAN_POINT('Ctrl Pts',(4.48463927434238,-25.5233462828554,11.4756630843606));
#2447=CARTESIAN_POINT('Ctrl Pts',(4.15760185288866,-24.7987006850272,11.4183460829245));
#2448=CARTESIAN_POINT('Ctrl Pts',(3.67680510493408,-24.1928234664463,11.3610662239878));
#2449=CARTESIAN_POINT('Ctrl Pts',(3.19600835697949,-23.5869462478655,11.3037863650511));
#2450=CARTESIAN_POINT('Ctrl Pts',(2.56315379146771,-23.099962191222,11.2464691751292));
#2451=CARTESIAN_POINT('Ctrl Pts',(1.85036321530309,-22.7909920845649,11.1891895436994));
#2452=CARTESIAN_POINT('Ctrl Pts',(1.13757263913847,-22.4820219779078,11.1319099122695));
#2453=CARTESIAN_POINT('Ctrl Pts',(0.346404347142174,-22.3503795041057,11.0745925365344));
#2454=CARTESIAN_POINT('Ctrl Pts',(-0.431256349503487,-22.4142584519129,
11.0173131291038));
#2455=CARTESIAN_POINT('Ctrl Pts',(-1.76387591167286,-22.5237230755283,10.9191576492385));
#2456=CARTESIAN_POINT('Ctrl Pts',(-3.04213419140331,-23.2249589278969,10.8209586709532));
#2457=CARTESIAN_POINT('Ctrl Pts',(-3.85596064138987,-24.2984448521308,10.7227780560402));
#2458=CARTESIAN_POINT('Ctrl Pts',(-4.26287386638314,-24.8351878142477,10.6736877485838));
#2459=CARTESIAN_POINT('Ctrl Pts',(-4.55417709738229,-25.4602183705301,10.6246080237907));
#2460=CARTESIAN_POINT('Ctrl Pts',(-4.70671246799434,-26.1188931345382,10.5755144999941));
#2461=CARTESIAN_POINT('Ctrl Pts',(-4.78211921639114,-26.444512838385,10.5512448307234));
#2462=CARTESIAN_POINT('Ctrl Pts',(-4.82402156275938,-26.7781833518283,10.5269769370843));
#2463=CARTESIAN_POINT('Ctrl Pts',(-4.83034694125566,-27.1129561266807,10.5027146395677));
#2464=CARTESIAN_POINT('Ctrl Pts',(-3.50000130290148,-27.2127226059667,0.497516610448255));
#2465=CARTESIAN_POINT('Ctrl Pts',(-3.51517971121378,-26.6400362227171,0.554808277114941));
#2466=CARTESIAN_POINT('Ctrl Pts',(-3.38700359289755,-26.0622729395371,0.612099943781561));
#2467=CARTESIAN_POINT('Ctrl Pts',(-2.87059541238073,-25.0317435939839,0.72668327711495));
#2468=CARTESIAN_POINT('Ctrl Pts',(-2.48281014130459,-24.5799885832371,0.783974943781635));
#2469=CARTESIAN_POINT('Ctrl Pts',(-1.53584837306688,-23.9107391275463,0.898558277114875));
#2470=CARTESIAN_POINT('Ctrl Pts',(-0.977548004253359,-23.6939293925514,
0.955849943781558));
#2471=CARTESIAN_POINT('Ctrl Pts',(0.179952606081418,-23.5494218341822,1.07043327711495));
#2472=CARTESIAN_POINT('Ctrl Pts',(0.778050826506515,-23.6219155146099,1.1277249437816));
#2473=CARTESIAN_POINT('Ctrl Pts',(1.87337605723642,-24.0427561003574,1.24230827711491));
#2474=CARTESIAN_POINT('Ctrl Pts',(2.36953479367315,-24.3907498795612,1.29959994378166));
#2475=CARTESIAN_POINT('Ctrl Pts',(3.14152373336449,-25.2835693957278,1.41418327711485));
#2476=CARTESIAN_POINT('Ctrl Pts',(3.41657407444237,-25.8275750154296,1.47147494378145));
#2477=CARTESIAN_POINT('Ctrl Pts',(3.67788264996072,-26.9856580353439,1.58605827711506));
#2478=CARTESIAN_POINT('Ctrl Pts',(3.66383841906194,-27.5986380524938,1.64334994378159));
#2479=CARTESIAN_POINT('Ctrl Pts',(3.34637070640969,-28.7497648633494,1.75793327711492));
#2480=CARTESIAN_POINT('Ctrl Pts',(3.04319969463925,-29.2867949482463,1.81522494378156));
#2481=CARTESIAN_POINT('Ctrl Pts',(2.21569737033779,-30.1572282923719,1.92980827711495));
#2482=CARTESIAN_POINT('Ctrl Pts',(1.69211980095435,-30.4897610442556,1.98709994378157));
#2483=CARTESIAN_POINT('Ctrl Pts',(0.545399706903326,-30.8693375696566,2.10168327711494));
#2484=CARTESIAN_POINT('Ctrl Pts',(-0.0766613991650282,-30.9159670184662,
2.1589749437815));
#2485=CARTESIAN_POINT('Ctrl Pts',(-1.27368280615195,-30.7088161970159,2.27355827711501));
#2486=CARTESIAN_POINT('Ctrl Pts',(-1.84748758998441,-30.4551815910792,2.33084994378156));
#2487=CARTESIAN_POINT('Ctrl Pts',(-2.81085451659558,-29.7038376853842,2.44543327711495));
#2488=CARTESIAN_POINT('Ctrl Pts',(-3.19946114294195,-29.2068057482841,2.50272494378152));
#2489=CARTESIAN_POINT('Ctrl Pts',(-3.69753671927098,-28.0836711179268,2.61730827711499));
#2490=CARTESIAN_POINT('Ctrl Pts',(-3.806479757265,-27.4586223362847,2.67459994378158));
#2491=CARTESIAN_POINT('Ctrl Pts',(-3.71562427983475,-26.2264419408016,2.78918327711493));
#2492=CARTESIAN_POINT('Ctrl Pts',(-3.51585940949974,-25.6204942820667,2.84647494378164));
#2493=CARTESIAN_POINT('Ctrl Pts',(-2.85104937088523,-24.5708949233056,2.96105827711487));
#2494=CARTESIAN_POINT('Ctrl Pts',(-2.38659565795852,-24.1282770115141,3.01834994378155));
#2495=CARTESIAN_POINT('Ctrl Pts',(-1.29941716743804,-23.5127467708991,3.13293327711496));
#2496=CARTESIAN_POINT('Ctrl Pts',(-0.677707157851868,-23.3404704661548,
3.19022494378159));
#2497=CARTESIAN_POINT('Ctrl Pts',(0.578163753723292,-23.3101136508809,3.30480827711492));
#2498=CARTESIAN_POINT('Ctrl Pts',(1.21112328389688,-23.4521157051967,3.36209994378163));
#2499=CARTESIAN_POINT('Ctrl Pts',(2.33910331776924,-24.020612363763,3.47668327711488));
#2500=CARTESIAN_POINT('Ctrl Pts',(2.83301955876491,-24.4466103465917,3.53397494378134));
#2501=CARTESIAN_POINT('Ctrl Pts',(3.56365851013518,-25.4854479877254,3.64855827711517));
#2502=CARTESIAN_POINT('Ctrl Pts',(3.79963778298962,-26.0973236259647,3.70584994378171));
#2503=CARTESIAN_POINT('Ctrl Pts',(3.95497605633098,-27.3647903302184,3.8204332771148));
#2504=CARTESIAN_POINT('Ctrl Pts',(3.87413319178915,-28.0191741775874,3.87772494378131));
#2505=CARTESIAN_POINT('Ctrl Pts',(3.41100678604432,-29.2165864086031,3.9923082771152));
#2506=CARTESIAN_POINT('Ctrl Pts',(3.02911682295908,-29.7584488581732,4.04959994378164));
#2507=CARTESIAN_POINT('Ctrl Pts',(2.05088106415332,-30.6005370966614,4.16418327711487));
#2508=CARTESIAN_POINT('Ctrl Pts',(1.45543709786498,-30.8999159637434,4.2214749437816));
#2509=CARTESIAN_POINT('Ctrl Pts',(0.188979096554336,-31.1827816634333,4.33605827711491));
#2510=CARTESIAN_POINT('Ctrl Pts',(-0.480833880026034,-31.1659454082194,
4.39334994378137));
#2511=CARTESIAN_POINT('Ctrl Pts',(-1.73770084949707,-30.8164017691893,4.50793327711514));
#2512=CARTESIAN_POINT('Ctrl Pts',(-2.32353697868073,-30.4839775401827,4.5652249437816));
#2513=CARTESIAN_POINT('Ctrl Pts',(-3.2721043301499,-29.5783412086159,4.67980827711491));
#2514=CARTESIAN_POINT('Ctrl Pts',(-3.63389029917657,-29.0059575948908,4.73709994378148));
#2515=CARTESIAN_POINT('Ctrl Pts',(-4.04554275106343,-27.7534973422558,4.85168327711503));
#2516=CARTESIAN_POINT('Ctrl Pts',(-4.09496422407853,-27.0746032767544,4.90897494378134));
#2517=CARTESIAN_POINT('Ctrl Pts',(-3.86625627856773,-25.7692068883448,5.02355827711517));
#2518=CARTESIAN_POINT('Ctrl Pts',(-3.58829314652568,-25.1439637579671,5.08084994378156));
#2519=CARTESIAN_POINT('Ctrl Pts',(-2.76684994212521,-24.0951805886606,5.19543327711495));
#2520=CARTESIAN_POINT('Ctrl Pts',(-2.22411429181341,-23.6726777785058,5.25272494378155));
#2521=CARTESIAN_POINT('Ctrl Pts',(-0.998892661235347,-23.1323163820897,
5.36730827711496));
#2522=CARTESIAN_POINT('Ctrl Pts',(-0.317558252613747,-23.0150241600847,
5.42459994378155));
#2523=CARTESIAN_POINT('Ctrl Pts',(1.02458823678216,-23.1167103523708,5.53918327711497));
#2524=CARTESIAN_POINT('Ctrl Pts',(1.68411116492473,-23.3356447606771,5.59647494378161));
#2525=CARTESIAN_POINT('Ctrl Pts',(2.82558639662397,-24.061844294864,5.7110582771149));
#2526=CARTESIAN_POINT('Ctrl Pts',(3.30641702010581,-24.568459238132,5.76834994378167));
#2527=CARTESIAN_POINT('Ctrl Pts',(3.97403573885252,-25.7530884168939,5.88293327711484));
#2528=CARTESIAN_POINT('Ctrl Pts',(4.16013798020538,-26.4299946596524,5.94022494378164));
#2529=CARTESIAN_POINT('Ctrl Pts',(4.19049479552954,-27.7963637440239,6.05480827711487));
#2530=CARTESIAN_POINT('Ctrl Pts',(4.03466680450649,-28.4845195073438,6.11209994378139));
#2531=CARTESIAN_POINT('Ctrl Pts',(3.41408166790506,-29.7099502295094,6.22668327711512));
#2532=CARTESIAN_POINT('Ctrl Pts',(2.94987097329771,-30.2460277007815,6.28397494378131));
#2533=CARTESIAN_POINT('Ctrl Pts',(1.8191574593059,-31.0380561478021,6.3985582771152));
#2534=CARTESIAN_POINT('Ctrl Pts',(1.15370655160782,-31.2932049585382,6.45584994378166));
#2535=CARTESIAN_POINT('Ctrl Pts',(-0.22372624653663,-31.4593739468365,6.57043327711484));
#2536=CARTESIAN_POINT('Ctrl Pts',(-0.934395720889725,-31.3701818981879,
6.62772494378144));
#2537=CARTESIAN_POINT('Ctrl Pts',(-2.23389495213891,-30.8647696724464,6.74230827711507));
#2538=CARTESIAN_POINT('Ctrl Pts',(-2.82146111488582,-30.4489835254622,6.79959994378158));
#2539=CARTESIAN_POINT('Ctrl Pts',(-3.73364865213651,-29.3853315240515,6.91418327711493));
#2540=CARTESIAN_POINT('Ctrl Pts',(-4.05735604524484,-28.7384492111523,6.97147494378131));
#2541=CARTESIAN_POINT('Ctrl Pts',(-4.36177886909609,-27.3636162284599,7.0860582771152));
#2542=CARTESIAN_POINT('Ctrl Pts',(-4.34215058957306,-26.6369702924209,7.14334994378177));
#2543=CARTESIAN_POINT('Ctrl Pts',(-3.96053102416322,-25.2743631643761,7.25793327711474));
#2544=CARTESIAN_POINT('Ctrl Pts',(-3.59885357791486,-24.6397209908769,7.31522494378181));
#2545=CARTESIAN_POINT('Ctrl Pts',(-2.61508323909598,-23.61301963208,7.4298082771147));
#2546=CARTESIAN_POINT('Ctrl Pts',(-1.9938935810033,-23.2219804458925,7.48709994378137));
#2547=CARTESIAN_POINT('Ctrl Pts',(-0.635693169822906,-22.7782520675398,
7.60168327711514));
#2548=CARTESIAN_POINT('Ctrl Pts',(0.100033855150708,-22.726038570305,7.65897494378174));
#2549=CARTESIAN_POINT('Ctrl Pts',(1.51380522494329,-22.9763036398845,7.77355827711478));
#2550=CARTESIAN_POINT('Ctrl Pts',(2.19048670189786,-23.2785952980398,7.8308499437815));
#2551=CARTESIAN_POINT('Ctrl Pts',(3.32468611387601,-24.1701378011219,7.94543327711501));
#2552=CARTESIAN_POINT('Ctrl Pts',(3.78108510785602,-24.7585771646693,8.00272494378146));
#2553=CARTESIAN_POINT('Ctrl Pts',(4.36373232434941,-26.085885795444,8.11730827711505));
#2554=CARTESIAN_POINT('Ctrl Pts',(4.48937373037522,-26.8235058310766,8.17459994378218));
#2555=CARTESIAN_POINT('Ctrl Pts',(4.37685682322345,-28.2756184143465,8.28918327711433));
#2556=CARTESIAN_POINT('Ctrl Pts',(4.13875287694128,-28.9887166119371,8.3464749437818));
#2557=CARTESIAN_POINT('Ctrl Pts',(3.35116384720094,-30.2220677165326,8.46105827711471));
#2558=CARTESIAN_POINT('Ctrl Pts',(2.80238767357428,-30.741111051742,8.51834994378256));
#2559=CARTESIAN_POINT('Ctrl Pts',(1.52030780658665,-31.4608182485878,8.63293327711395));
#2560=CARTESIAN_POINT('Ctrl Pts',(0.788205330640013,-31.6607464265703,8.69022494378047));
#2561=CARTESIAN_POINT('Ctrl Pts',(-0.688661926511778,-31.6911032419353,
8.80480827711605));
#2562=CARTESIAN_POINT('Ctrl Pts',(-1.43201392300667,-31.5214493142069,8.86209994378189));
#2563=CARTESIAN_POINT('Ctrl Pts',(-2.75489533342443,-30.8487756995759,8.97668327711462));
#2564=CARTESIAN_POINT('Ctrl Pts',(-3.33313403500641,-30.3463522931823,9.03397494378135));
#2565=CARTESIAN_POINT('Ctrl Pts',(-4.18655197765132,-29.123762906342,9.14855827711516));
#2566=CARTESIAN_POINT('Ctrl Pts',(-4.46087032628663,-28.4047367291627,9.20584994378135));
#2567=CARTESIAN_POINT('Ctrl Pts',(-4.63787002953295,-26.9173378371627,9.32043327711516));
#2568=CARTESIAN_POINT('Ctrl Pts',(-4.54032879677263,-26.1503827357956,9.37772494378163));
#2569=CARTESIAN_POINT('Ctrl Pts',(-3.99263075105309,-24.7487965043376,9.49230827711489));
#2570=CARTESIAN_POINT('Ctrl Pts',(-3.54294842016277,-24.1155266283949,9.54959994378147));
#2571=CARTESIAN_POINT('Ctrl Pts',(-2.393880176143,-23.1332397923951,9.66418327711504));
#2572=CARTESIAN_POINT('Ctrl Pts',(-1.69555951661787,-22.7852038732428,9.72147494378146));
#2573=CARTESIAN_POINT('Ctrl Pts',(-0.21235155257781,-22.4592239252521,9.83605827711505));
#2574=CARTESIAN_POINT('Ctrl Pts',(0.571127342942618,-22.4816442290709,9.8933499437812));
#2575=CARTESIAN_POINT('Ctrl Pts',(2.03947462954967,-22.8953397208652,10.0079332771153));
#2576=CARTESIAN_POINT('Ctrl Pts',(2.72292284739241,-23.2862703843579,10.0652249437816));
#2577=CARTESIAN_POINT('Ctrl Pts',(3.82775821347252,-24.3481747304191,10.179808277115));
#2578=CARTESIAN_POINT('Ctrl Pts',(4.24805061685128,-25.0181704328983,10.237099943781));
#2579=CARTESIAN_POINT('Ctrl Pts',(4.72385492165356,-26.4821110025959,10.3516832771155));
#2580=CARTESIAN_POINT('Ctrl Pts',(4.77886044311237,-27.2746709870712,10.4089749437799));
#2581=CARTESIAN_POINT('Ctrl Pts',(4.50703824947158,-28.796817338216,10.5235582771166));
#2582=CARTESIAN_POINT('Ctrl Pts',(4.18041806520056,-29.5249371617849,10.580849943781));
#2583=CARTESIAN_POINT('Ctrl Pts',(3.21877626343458,-30.7445528163907,10.6954332771156));
#2584=CARTESIAN_POINT('Ctrl Pts',(2.58463318663832,-31.2348479942316,10.752724943781));
#2585=CARTESIAN_POINT('Ctrl Pts',(1.15523755569548,-31.8597810307748,10.8673082771155));
#2586=CARTESIAN_POINT('Ctrl Pts',(0.361331893025007,-31.9937716208391,10.9245999437816));
#2587=CARTESIAN_POINT('Ctrl Pts',(-1.20074678409337,-31.8704239988137,11.0391832771149));
#2588=CARTESIAN_POINT('Ctrl Pts',(-1.96742025115454,-31.6131505145616,11.0964749437817));
#2589=CARTESIAN_POINT('Ctrl Pts',(-3.29264722862687,-30.7641719892639,11.2110582771148));
#2590=CARTESIAN_POINT('Ctrl Pts',(-3.84990327557803,-30.1732345852601,11.2683499437819));
#2591=CARTESIAN_POINT('Ctrl Pts',(-4.62169895051392,-28.7937040300877,11.3829332771146));
#2592=CARTESIAN_POINT('Ctrl Pts',(-4.83545306471002,-28.0064053323945,11.4402249437801));
#2593=CARTESIAN_POINT('Ctrl Pts',(-4.85063147283344,-27.2127226059663,11.4975166104483));
#2594=CARTESIAN_POINT('Ctrl Pts',(-2.50007468503219,-27.2005618150104,0.498733179016744));
#2595=CARTESIAN_POINT('Ctrl Pts',(-2.51326328854572,-26.7914880446566,0.55602484568343));
#2596=CARTESIAN_POINT('Ctrl Pts',(-2.424042889801,-26.3776787977216,0.613316512350049));
#2597=CARTESIAN_POINT('Ctrl Pts',(-2.05837790695547,-25.6376123049861,0.727899845683439));
#2598=CARTESIAN_POINT('Ctrl Pts',(-1.78223591282738,-25.3120882495965,0.785191512350124));
#2599=CARTESIAN_POINT('Ctrl Pts',(-1.10514101707629,-24.8279443088378,0.899774845683364));
#2600=CARTESIAN_POINT('Ctrl Pts',(-0.704806088645041,-24.6698320611445,
0.957066512350047));
#2601=CARTESIAN_POINT('Ctrl Pts',(0.127435052567004,-24.5613586294748,1.07164984568344));
#2602=CARTESIAN_POINT('Ctrl Pts',(0.558550388136447,-24.611154478993,1.12894151235009));
#2603=CARTESIAN_POINT('Ctrl Pts',(1.35003600685502,-24.9104480749466,1.2435248456834));
#2604=CARTESIAN_POINT('Ctrl Pts',(1.70962866979797,-25.1597089674028,1.30081651235015));
#2605=CARTESIAN_POINT('Ctrl Pts',(2.27095184904808,-25.8021046070125,1.41539984568334));
#2606=CARTESIAN_POINT('Ctrl Pts',(2.47210402656363,-26.1946587930152,1.47269151234994));
#2607=CARTESIAN_POINT('Ctrl Pts',(2.66567098650756,-27.0325805190397,1.58727484568355));
#2608=CARTESIAN_POINT('Ctrl Pts',(2.65784810539905,-27.4771569431548,1.64456651235008));
#2609=CARTESIAN_POINT('Ctrl Pts',(2.43156061069391,-28.3139935243568,1.75914984568341));
#2610=CARTESIAN_POINT('Ctrl Pts',(2.21326124381233,-28.7054376235712,1.81644151235005));
#2611=CARTESIAN_POINT('Ctrl Pts',(1.61432808129647,-29.341673788178,1.93102484568344));
#2612=CARTESIAN_POINT('Ctrl Pts',(1.23422937884041,-29.5858193799578,1.98831651235005));
#2613=CARTESIAN_POINT('Ctrl Pts',(0.399489075163559,-29.8665991896874,2.10289984568343));
#2614=CARTESIAN_POINT('Ctrl Pts',(-0.0543695483476922,-29.902913592182,
2.16019151234999));
#2615=CARTESIAN_POINT('Ctrl Pts',(-0.929676894760097,-29.7556981014736,
2.2747748456835));
#2616=CARTESIAN_POINT('Ctrl Pts',(-1.35027785335415,-29.5722565382445,2.33206651235005));
#2617=CARTESIAN_POINT('Ctrl Pts',(-2.05817162822115,-29.0254258335761,2.44664984568344));
#2618=CARTESIAN_POINT('Ctrl Pts',(-2.34475331460298,-28.6625184167178,2.50394151235001));
#2619=CARTESIAN_POINT('Ctrl Pts',(-2.71392854153148,-27.8401775372868,2.61852484568348));
#2620=CARTESIAN_POINT('Ctrl Pts',(-2.79611947665046,-27.38151024587,2.67581651235007));
#2621=CARTESIAN_POINT('Ctrl Pts',(-2.73337723274891,-26.4753694596141,2.79039984568342));
#2622=CARTESIAN_POINT('Ctrl Pts',(-2.58845080557611,-26.0287680290841,2.84769151235013));
#2623=CARTESIAN_POINT('Ctrl Pts',(-2.10212843329669,-25.253457448189,2.96227484568336));
#2624=CARTESIAN_POINT('Ctrl Pts',(-1.76115320148598,-24.925519700272,3.01956651235004));
#2625=CARTESIAN_POINT('Ctrl Pts',(-0.960685614181144,-24.4677520619668,
3.13414984568345));
#2626=CARTESIAN_POINT('Ctrl Pts',(-0.501933757791044,-24.3384072792704,
3.19144151235008));
#2627=CARTESIAN_POINT('Ctrl Pts',(0.426711935575103,-24.3120300735039,3.30602484568341));
#2628=CARTESIAN_POINT('Ctrl Pts',(0.895717425864195,-24.4150764083739,3.36331651235012));
#2629=CARTESIAN_POINT('Ctrl Pts',(1.73323460661518,-24.8328298691077,3.47789984568337));
#2630=CARTESIAN_POINT('Ctrl Pts',(2.10091989250226,-25.1471845752111,3.53519151234975));
#2631=CARTESIAN_POINT('Ctrl Pts',(2.64645332874688,-25.9161553435738,3.64977484568374));
#2632=CARTESIAN_POINT('Ctrl Pts',(2.82373511441566,-26.3700655417409,3.70706651235029));
#2633=CARTESIAN_POINT('Ctrl Pts',(2.94303926101928,-27.3122727765361,3.8216498456832));
#2634=CARTESIAN_POINT('Ctrl Pts',(2.88489422734382,-27.7996737393716,3.8789415123498));
#2635=CARTESIAN_POINT('Ctrl Pts',(2.54331481151743,-28.6932463580673,3.99352484568369));
#2636=CARTESIAN_POINT('Ctrl Pts',(2.26015773499116,-29.0985427344035,4.05081651235013));
#2637=CARTESIAN_POINT('Ctrl Pts',(1.53234585299496,-29.7299652122396,4.16539984568336));
#2638=CARTESIAN_POINT('Ctrl Pts',(1.08835332012082,-29.9554459158982,4.22269151235009));
#2639=CARTESIAN_POINT('Ctrl Pts',(0.142056613017233,-30.1705699999466,4.3372748456834));
#2640=CARTESIAN_POINT('Ctrl Pts',(-0.359352770840531,-30.1599550945101,
4.39456651234986));
#2641=CARTESIAN_POINT('Ctrl Pts',(-1.30192951035091,-29.9015916735199,4.50914984568362));
#2642=CARTESIAN_POINT('Ctrl Pts',(-1.74217965412023,-29.6540390892461,4.56644151235009));
#2643=CARTESIAN_POINT('Ctrl Pts',(-2.45654982584139,-28.9769719196844,4.6810248456834));
#2644=CARTESIAN_POINT('Ctrl Pts',(-2.72994863492545,-28.5480671726279,4.73831651234997));
#2645=CARTESIAN_POINT('Ctrl Pts',(-3.04280437104754,-27.607586710665,4.85289984568352));
#2646=CARTESIAN_POINT('Ctrl Pts',(-3.08191079776549,-27.0968951274201,4.91019151234983));
#2647=CARTESIAN_POINT('Ctrl Pts',(-2.91313818305431,-26.1132127998883,5.02477484568366));
#2648=CARTESIAN_POINT('Ctrl Pts',(-2.7053680935962,-25.641173494479,5.08206651235005));
#2649=CARTESIAN_POINT('Ctrl Pts',(-2.08843809041187,-24.8478634771535,5.19664984568344));
#2650=CARTESIAN_POINT('Ctrl Pts',(-1.67982696010923,-24.527385606786,5.25394151235004));
#2651=CARTESIAN_POINT('Ctrl Pts',(-0.755399080733289,-24.115924559888,5.36852484568345));
#2652=CARTESIAN_POINT('Ctrl Pts',(-0.240446162052198,-24.025384440712,5.42581651235003));
#2653=CARTESIAN_POINT('Ctrl Pts',(0.775660717822627,-24.0989573994438,5.54039984568345));
#2654=CARTESIAN_POINT('Ctrl Pts',(1.27583741803011,-24.2630533646806,5.5976915123501));
#2655=CARTESIAN_POINT('Ctrl Pts',(2.14302387161775,-24.8107652323726,5.71227484568339));
#2656=CARTESIAN_POINT('Ctrl Pts',(2.50917433141652,-25.1939016947322,5.76956651235015));
#2657=CARTESIAN_POINT('Ctrl Pts',(3.01903044771613,-26.0918199700231,5.88414984568333));
#2658=CARTESIAN_POINT('Ctrl Pts',(3.16220116709098,-26.605768059855,5.94144151235013));
#2659=CARTESIAN_POINT('Ctrl Pts',(3.18857837290535,-27.6449119257339,6.05602484568335));
#2660=CARTESIAN_POINT('Ctrl Pts',(3.07170610126387,-28.1691136494362,6.11331651234988));
#2661=CARTESIAN_POINT('Ctrl Pts',(2.60186416262591,-29.1040815182302,6.22789984568361));
#2662=CARTESIAN_POINT('Ctrl Pts',(2.24929674456444,-29.5139280345983,6.2851915123498));
#2663=CARTESIAN_POINT('Ctrl Pts',(1.38845010357141,-30.1208509663343,6.39977484568369));
#2664=CARTESIAN_POINT('Ctrl Pts',(0.880964635695304,-30.3173022899789,6.45706651235015));
#2665=CARTESIAN_POINT('Ctrl Pts',(-0.171208692717956,-30.4474371515102,
6.57164984568333));
#2666=CARTESIAN_POINT('Ctrl Pts',(-0.714895282800354,-30.3809429336921,
6.62894151234993));
#2667=CARTESIAN_POINT('Ctrl Pts',(-1.71055490147675,-29.99707769797,6.74352484568356));
#2668=CARTESIAN_POINT('Ctrl Pts',(-2.1615549912013,-29.680024437392,6.80081651235007));
#2669=CARTESIAN_POINT('Ctrl Pts',(-2.8630767676294,-28.8667963129956,6.91539984568342));
#2670=CARTESIAN_POINT('Ctrl Pts',(-3.11288599742707,-28.3713654332789,6.9726915123498));
#2671=CARTESIAN_POINT('Ctrl Pts',(-3.34956720558195,-27.316693745052,7.08727484568369));
#2672=CARTESIAN_POINT('Ctrl Pts',(-3.33616027582943,-26.758451401481,7.14456651235026));
#2673=CARTESIAN_POINT('Ctrl Pts',(-3.0457209285282,-25.7101345036477,7.25914984568322));
#2674=CARTESIAN_POINT('Ctrl Pts',(-2.76891512688693,-25.2210783153451,7.31644151235029));
#2675=CARTESIAN_POINT('Ctrl Pts',(-2.01371395025572,-24.4285741364808,7.43102484568319));
#2676=CARTESIAN_POINT('Ctrl Pts',(-1.53600315861845,-24.1259221101056,7.48831651234986));
#2677=CARTESIAN_POINT('Ctrl Pts',(-0.489782538354123,-23.7809904475937,
7.60289984568363));
#2678=CARTESIAN_POINT('Ctrl Pts',(0.0777420046090931,-23.7390919966418,
7.66019151235023));
#2679=CARTESIAN_POINT('Ctrl Pts',(1.16979931327565,-23.9294217353742,7.77477484568326));
#2680=CARTESIAN_POINT('Ctrl Pts',(1.69327696548401,-24.1615203510483,7.83206651235037));
#2681=CARTESIAN_POINT('Ctrl Pts',(2.57200322528511,-24.8485496527562,7.94664984568312));
#2682=CARTESIAN_POINT('Ctrl Pts',(2.92637727962451,-25.3028644964882,8.00394151234995));
#2683=CARTESIAN_POINT('Ctrl Pts',(3.38012414650242,-26.3293793758314,8.11852484568354));
#2684=CARTESIAN_POINT('Ctrl Pts',(3.47901344973788,-26.9006179217584,8.17581651235106));
#2685=CARTESIAN_POINT('Ctrl Pts',(3.39460977616041,-28.0266908952667,8.29039984568243));
#2686=CARTESIAN_POINT('Ctrl Pts',(3.21134427287294,-28.5804428651419,8.34769151235029));
#2687=CARTESIAN_POINT('Ctrl Pts',(2.60224290975714,-29.539505191427,8.4622748456832));
#2688=CARTESIAN_POINT('Ctrl Pts',(2.17694521686884,-29.9438683631093,8.51956651235105));
#2689=CARTESIAN_POINT('Ctrl Pts',(1.18157625356271,-30.5058129573948,8.63414984568244));
#2690=CARTESIAN_POINT('Ctrl Pts',(0.612431930317692,-30.662809613458,8.69144151234896));
#2691=CARTESIAN_POINT('Ctrl Pts',(-0.537210108102021,-30.689186819309,8.80602484568453));
#2692=CARTESIAN_POINT('Ctrl Pts',(-1.11660806520128,-30.5584886109117,8.86331651235037));
#2693=CARTESIAN_POINT('Ctrl Pts',(-2.149026622043,-30.0365581943494,8.97789984568311));
#2694=CARTESIAN_POINT('Ctrl Pts',(-2.60103436888815,-29.6457780643529,9.03519151234983));
#2695=CARTESIAN_POINT('Ctrl Pts',(-3.2693467961186,-28.6930555507037,9.14977484568365));
#2696=CARTESIAN_POINT('Ctrl Pts',(-3.48496765774055,-28.1319948131383,9.20706651234983));
#2697=CARTESIAN_POINT('Ctrl Pts',(-3.62593323419338,-26.9698553910934,9.32164984568365));
#2698=CARTESIAN_POINT('Ctrl Pts',(-3.55108983223544,-26.3698831737798,9.37894151235011));
#2699=CARTESIAN_POINT('Ctrl Pts',(-3.12493877661809,-25.2721365551049,9.49352484568337));
#2700=CARTESIAN_POINT('Ctrl Pts',(-2.77398933200833,-24.7754327520073,9.55081651234996));
#2701=CARTESIAN_POINT('Ctrl Pts',(-1.87534496517122,-24.0038116769744,9.66539984568352));
#2702=CARTESIAN_POINT('Ctrl Pts',(-1.32847573863619,-23.7296739210376,9.72269151234995));
#2703=CARTESIAN_POINT('Ctrl Pts',(-0.165429069278296,-23.4714355887892,
9.83727484568354));
#2704=CARTESIAN_POINT('Ctrl Pts',(0.449646233987307,-23.4876345428461,9.89456651234969));
#2705=CARTESIAN_POINT('Ctrl Pts',(1.60370329017324,-23.8101498164686,10.0091498456838));
#2706=CARTESIAN_POINT('Ctrl Pts',(2.14156552300047,-24.1162088354615,10.06644151235));
#2707=CARTESIAN_POINT('Ctrl Pts',(3.01220370899539,-24.9495440191837,10.1810248456835));
#2708=CARTESIAN_POINT('Ctrl Pts',(3.34410895267091,-25.4760608553855,10.2383165123495));
#2709=CARTESIAN_POINT('Ctrl Pts',(3.72111654156689,-26.6280216339623,10.352899845684));
#2710=CARTESIAN_POINT('Ctrl Pts',(3.76580701675634,-27.2523791366326,10.4101915123484));
#2711=CARTESIAN_POINT('Ctrl Pts',(3.55392015400117,-28.4528114264453,10.5247748456851));
#2712=CARTESIAN_POINT('Ctrl Pts',(3.29749301212752,-29.0277274254513,10.5820665123494));
#2713=CARTESIAN_POINT('Ctrl Pts',(2.54036441186484,-29.9918699277194,10.696649845684));
#2714=CARTESIAN_POINT('Ctrl Pts',(2.04034585472464,-30.3801401660391,10.7539415123495));
#2715=CARTESIAN_POINT('Ctrl Pts',(0.911743975403001,-30.8761728528888,10.868524845684));
#2716=CARTESIAN_POINT('Ctrl Pts',(0.284219802238695,-30.9834113401931,10.9258165123501));
#2717=CARTESIAN_POINT('Ctrl Pts',(-0.951819264909011,-30.8881769517593,
11.0403998456834));
#2718=CARTESIAN_POINT('Ctrl Pts',(-1.55914650444578,-30.6857419104376,11.0976915123502));
#2719=CARTESIAN_POINT('Ctrl Pts',(-2.61008470343474,-30.0152510518758,11.2122748456833));
#2720=CARTESIAN_POINT('Ctrl Pts',(-3.0526605869948,-29.5477921284695,11.2695665123504));
#2721=CARTESIAN_POINT('Ctrl Pts',(-3.66669365927143,-28.4549724771489,11.3841498456831));
#2722=CARTESIAN_POINT('Ctrl Pts',(-3.83751625162752,-27.8306319296078,11.4414415123486));
#2723=CARTESIAN_POINT('Ctrl Pts',(-3.85070485496414,-27.2005618150101,11.4987331790167));
#2724=CARTESIAN_POINT('Ctrl Pts',(-2.50007468503219,-27.1010184425723,-0.496300045053517));
#2725=CARTESIAN_POINT('Ctrl Pts',(-2.4969755420553,-26.6919446722147,-0.439008378386831));
#2726=CARTESIAN_POINT('Ctrl Pts',(-2.39148297849306,-26.282211390483,-0.381716711720212));
#2727=CARTESIAN_POINT('Ctrl Pts',(-1.99708897638351,-25.5575008784686,-0.267133378386822));
#2728=CARTESIAN_POINT('Ctrl Pts',(-1.70851761043281,-25.2432421490424,-0.209841711720177));
#2729=CARTESIAN_POINT('Ctrl Pts',(-1.01332474089414,-24.78618374015,-0.0952583783868566));
#2730=CARTESIAN_POINT('Ctrl Pts',(-0.607338523048543,-24.6438657882886,
-0.0379667117201735));
#2731=CARTESIAN_POINT('Ctrl Pts',(0.228095574754098,-24.5678109889204,0.0766166216131396));
#2732=CARTESIAN_POINT('Ctrl Pts',(0.656749523111612,-24.6342001631764,0.133908288279827));
#2733=CARTESIAN_POINT('Ctrl Pts',(1.43576904066519,-24.9635895896308,0.248491621613139));
#2734=CARTESIAN_POINT('Ctrl Pts',(1.78536891475194,-25.2263241981206,0.305783288279848));
#2735=CARTESIAN_POINT('Ctrl Pts',(2.32151089800951,-25.8893855112099,0.420366621613118));
#2736=CARTESIAN_POINT('Ctrl Pts',(2.50749875677538,-26.2891118858318,0.477658288279721));
#2737=CARTESIAN_POINT('Ctrl Pts',(2.66911615346284,-27.133388775121,0.592241621613245));
#2738=CARTESIAN_POINT('Ctrl Pts',(2.64453859088259,-27.5771420945141,0.649533288279816));
#2739=CARTESIAN_POINT('Ctrl Pts',(2.38707829372837,-28.404522509479,0.76411662161315));
#2740=CARTESIAN_POINT('Ctrl Pts',(2.15439062586044,-28.7873425929663,0.821408288279792));
#2741=CARTESIAN_POINT('Ctrl Pts',(1.53242311190211,-29.4005444061292,0.935991621613174));
#2742=CARTESIAN_POINT('Ctrl Pts',(1.14370039372121,-29.6303016969254,0.993283288279668));
#2743=CARTESIAN_POINT('Ctrl Pts',(0.299503923801187,-29.8799087042019,1.1078666216133));
#2744=CARTESIAN_POINT('Ctrl Pts',(-0.155177804428747,-29.8994684252318,
1.16515828827989));
#2745=CARTESIAN_POINT('Ctrl Pts',(-1.02412998757692,-29.7203033712568,1.27974162161307));
#2746=CARTESIAN_POINT('Ctrl Pts',(-1.43755875755687,-29.5216974892904,1.33703328827979));
#2747=CARTESIAN_POINT('Ctrl Pts',(-2.12478685893361,-28.9496855886148,1.45161662161318));
#2748=CARTESIAN_POINT('Ctrl Pts',(-2.39789482929683,-28.5767853829115,1.50890828827974));
#2749=CARTESIAN_POINT('Ctrl Pts',(-2.73697422570521,-27.7419784023078,1.62349162161322));
#2750=CARTESIAN_POINT('Ctrl Pts',(-2.80257183610632,-27.280849723684,1.68078328827981));
#2751=CARTESIAN_POINT('Ctrl Pts',(-2.70741095988276,-26.3779018940165,1.79536662161316));
#2752=CARTESIAN_POINT('Ctrl Pts',(-2.54669023689932,-25.9369517528952,1.85265828827987));
#2753=CARTESIAN_POINT('Ctrl Pts',(-2.03328233273154,-25.1797391458012,1.9672416216131));
#2754=CARTESIAN_POINT('Ctrl Pts',(-1.68104177497557,-24.8642307696851,2.02453328827986));
#2755=CARTESIAN_POINT('Ctrl Pts',(-0.865218206935421,-24.4351921506738,
2.1391166216131));
#2756=CARTESIAN_POINT('Ctrl Pts',(-0.402390385352991,-24.3221195331577,
2.19640828827973));
#2757=CARTESIAN_POINT('Ctrl Pts',(0.526255308013156,-24.3283178196167,2.31099162161323));
#2758=CARTESIAN_POINT('Ctrl Pts',(0.991184833112652,-24.4476363196676,2.36828328827977));
#2759=CARTESIAN_POINT('Ctrl Pts',(1.81334603312285,-24.8941187996939,2.4828666216132));
#2760=CARTESIAN_POINT('Ctrl Pts',(2.16976599307112,-25.2209028775953,2.54015828827966));
#2761=CARTESIAN_POINT('Ctrl Pts',(2.68821389741996,-26.0079716197664,2.65474162161331));
#2762=CARTESIAN_POINT('Ctrl Pts',(2.84970138728746,-26.4675331073362,2.71203328827994));
#2763=CARTESIAN_POINT('Ctrl Pts',(2.93658690155775,-27.4129332987244,2.82661662161303));
#2764=CARTESIAN_POINT('Ctrl Pts',(2.86184854317733,-27.8978728743535,2.88390828827962));
#2765=CARTESIAN_POINT('Ctrl Pts',(2.49017329681634,-28.7789793918707,2.99849162161334));
#2766=CARTESIAN_POINT('Ctrl Pts',(2.19354250428536,-29.1742829793717,3.05578328827987));
#2767=CARTESIAN_POINT('Ctrl Pts',(1.44506494878558,-29.7805242611867,3.1703666216131));
#2768=CARTESIAN_POINT('Ctrl Pts',(0.993900227308371,-29.9908406461274,3.22765828827983));
#2769=CARTESIAN_POINT('Ctrl Pts',(0.0412483569317987,-30.1740151668844,
3.34224162161314));
#2770=CARTESIAN_POINT('Ctrl Pts',(-0.459337922206362,-30.1466455800109,
3.3995332882796));
#2771=CARTESIAN_POINT('Ctrl Pts',(-1.39245849546665,-29.8571093565371,3.51411662161336));
#2772=CARTESIAN_POINT('Ctrl Pts',(-1.82408462352403,-29.5951684713072,3.57140828827983));
#2773=CARTESIAN_POINT('Ctrl Pts',(-2.51542044378384,-28.895066950277,3.68599162161314));
#2774=CARTESIAN_POINT('Ctrl Pts',(-2.77443095190869,-28.4575381875142,3.74328328827971));
#2775=CARTESIAN_POINT('Ctrl Pts',(-3.0561138855463,-27.5076015592972,3.85786662161326));
#2776=CARTESIAN_POINT('Ctrl Pts',(-3.07846563082932,-26.9960868713341,3.91515828827957));
#2777=CARTESIAN_POINT('Ctrl Pts',(-2.87774345282345,-26.0187597070765,4.0297416216134));
#2778=CARTESIAN_POINT('Ctrl Pts',(-2.6548090446523,-25.5538925902661,4.0870332882796));
#2779=CARTESIAN_POINT('Ctrl Pts',(-2.01269784544036,-24.7812482464512,4.20161662161336));
#2780=CARTESIAN_POINT('Ctrl Pts',(-1.59409392630807,-24.4742440920755,4.25890828827978));
#2781=CARTESIAN_POINT('Ctrl Pts',(-0.657199945749121,-24.0928788757309,
4.37349162161319));
#2782=CARTESIAN_POINT('Ctrl Pts',(-0.13978563986163,-24.0189320812405,4.43078328827959));
#2783=CARTESIAN_POINT('Ctrl Pts',(0.873128283415644,-24.1249236723256,4.54536662161338));
#2784=CARTESIAN_POINT('Ctrl Pts',(1.36765369423033,-24.3048139333446,4.60265828827984));
#2785=CARTESIAN_POINT('Ctrl Pts',(2.21674217399424,-24.8796113329506,4.71724162161312));
#2786=CARTESIAN_POINT('Ctrl Pts',(2.57046326201523,-25.2740131212371,4.77453328828008));
#2787=CARTESIAN_POINT('Ctrl Pts',(3.05159035899733,-26.1872873772743,4.88911662161288));
#2788=CARTESIAN_POINT('Ctrl Pts',(3.17848891321873,-26.705311432293,4.94640828827969));
#2789=CARTESIAN_POINT('Ctrl Pts',(3.17229062677759,-27.7444552981719,5.06099162161328));
#2790=CARTESIAN_POINT('Ctrl Pts',(3.03914618998225,-28.2645810566892,5.11828328827961));
#2791=CARTESIAN_POINT('Ctrl Pts',(2.54057523202762,-29.1841929447334,5.23286662161335));
#2792=CARTESIAN_POINT('Ctrl Pts',(2.17557844218674,-29.5827741351755,5.29015828827954));
#2793=CARTESIAN_POINT('Ctrl Pts',(1.2966338273724,-30.1626115349991,5.40474162161343));
#2794=CARTESIAN_POINT('Ctrl Pts',(0.783497070102546,-30.3432685628663,5.46203328828008));
#2795=CARTESIAN_POINT('Ctrl Pts',(-0.271869214908782,-30.440984792033,5.57661662161288));
#2796=CARTESIAN_POINT('Ctrl Pts',(-0.813094417788087,-30.3578972495394,
5.63390828827948));
#2797=CARTESIAN_POINT('Ctrl Pts',(-1.79628793527435,-29.9439361832551,5.74849162161349));
#2798=CARTESIAN_POINT('Ctrl Pts',(-2.23729523617899,-29.6134092066964,5.80578328828));
#2799=CARTESIAN_POINT('Ctrl Pts',(-2.9136358165671,-28.7795154087759,5.92036662161297));
#2800=CARTESIAN_POINT('Ctrl Pts',(-3.14828072766742,-28.2769123404668,5.97765828827954));
#2801=CARTESIAN_POINT('Ctrl Pts',(-3.35301237250861,-27.2158854889663,6.09224162161343));
#2802=CARTESIAN_POINT('Ctrl Pts',(-3.32285076134111,-26.6584662501118,6.14953328827981));
#2803=CARTESIAN_POINT('Ctrl Pts',(-3.00123861153452,-25.6196055185354,6.26411662161316));
#2804=CARTESIAN_POINT('Ctrl Pts',(-2.71004450895648,-25.1391733459278,6.32140828828022));
#2805=CARTESIAN_POINT('Ctrl Pts',(-1.93180898083992,-24.3697035185519,6.43599162161274));
#2806=CARTESIAN_POINT('Ctrl Pts',(-1.4454741735086,-24.0814397931112,6.49328328827941));
#2807=CARTESIAN_POINT('Ctrl Pts',(-0.389797386982391,-23.7676809331061,
6.60786662161356));
#2808=CARTESIAN_POINT('Ctrl Pts',(0.178550260697191,-23.7425371635652,6.66515828827996));
#2809=CARTESIAN_POINT('Ctrl Pts',(1.26425240608542,-23.9648164656178,6.779741621613));
#2810=CARTESIAN_POINT('Ctrl Pts',(1.78055786970335,-24.2120793999817,6.83703328828011));
#2811=CARTESIAN_POINT('Ctrl Pts',(2.63861845598095,-24.9242898977382,6.95161662161285));
#2812=CARTESIAN_POINT('Ctrl Pts',(2.97951879434458,-25.3885975302847,7.00890828827969));
#2813=CARTESIAN_POINT('Ctrl Pts',(3.40316983064992,-26.4275785108202,7.12349162161328));
#2814=CARTESIAN_POINT('Ctrl Pts',(3.48546580921967,-27.0012784439486,7.18078328828002));
#2815=CARTESIAN_POINT('Ctrl Pts',(3.36864350326833,-28.12415846086,7.29536662161295));
#2816=CARTESIAN_POINT('Ctrl Pts',(3.16958370421836,-28.6722591413468,7.35265828828003));
#2817=CARTESIAN_POINT('Ctrl Pts',(2.53339680916978,-29.6132234937987,7.46724162161294));
#2818=CARTESIAN_POINT('Ctrl Pts',(2.09683379037026,-30.0051572937212,7.5245332882802));
#2819=CARTESIAN_POINT('Ctrl Pts',(1.08610884630516,-30.5383728686628,7.63911662161277));
#2820=CARTESIAN_POINT('Ctrl Pts',(0.512888557879637,-30.6790973595949,7.6964082882785));
#2821=CARTESIAN_POINT('Ctrl Pts',(-0.636753480540073,-30.6728990731721,
7.81099162161447));
#2822=CARTESIAN_POINT('Ctrl Pts',(-1.21207547246262,-30.5259286996412,7.86828328828011));
#2823=CARTESIAN_POINT('Ctrl Pts',(-2.22913804853779,-29.97526926374,7.98286662161285));
#2824=CARTESIAN_POINT('Ctrl Pts',(-2.66988046947652,-29.5720597619835,8.04015828827957));
#2825=CARTESIAN_POINT('Ctrl Pts',(-3.31110736477216,-28.6012392744964,8.15474162161339));
#2826=CARTESIAN_POINT('Ctrl Pts',(-3.51093393063736,-28.0345272475469,8.21203328827957));
#2827=CARTESIAN_POINT('Ctrl Pts',(-3.61948087470683,-26.8691948689011,8.32661662161339));
#2828=CARTESIAN_POINT('Ctrl Pts',(-3.52804414809214,-26.2716840387888,8.38390828827985));
#2829=CARTESIAN_POINT('Ctrl Pts',(-3.07179726189379,-25.1864035213107,8.49849162161311));
#2830=CARTESIAN_POINT('Ctrl Pts',(-2.70737410131727,-24.69969250702,8.5557832882797));
#2831=CARTESIAN_POINT('Ctrl Pts',(-1.78806406094709,-23.9532526280462,8.67036662161327));
#2832=CARTESIAN_POINT('Ctrl Pts',(-1.23402264582689,-23.6942791907854,8.72765828827969));
#2833=CARTESIAN_POINT('Ctrl Pts',(-0.0646208131897154,-23.4679904218743,
8.84224162161328));
#2834=CARTESIAN_POINT('Ctrl Pts',(0.549631385361328,-23.5009440573235,8.89953328827943));
#2835=CARTESIAN_POINT('Ctrl Pts',(1.69423227528079,-23.8546321334732,9.01411662161354));
#2836=CARTESIAN_POINT('Ctrl Pts',(2.2234704924224,-24.1750794533858,9.07140828827978));
#2837=CARTESIAN_POINT('Ctrl Pts',(3.0710743269197,-25.0314489886056,9.18599162161319));
#2838=CARTESIAN_POINT('Ctrl Pts',(3.38859126967608,-25.566589840493,9.24328328827926));
#2839=CARTESIAN_POINT('Ctrl Pts',(3.73442605604372,-26.7280067853365,9.3578666216137));
#2840=CARTESIAN_POINT('Ctrl Pts',(3.76236184984361,-27.3531873927232,9.41515828827891));
#2841=CARTESIAN_POINT('Ctrl Pts',(3.51852542374687,-28.5472645192526,9.52974162161405));
#2842=CARTESIAN_POINT('Ctrl Pts',(3.24693396320241,-29.1150083296771,9.58703328827918));
#2843=CARTESIAN_POINT('Ctrl Pts',(2.46462416687454,-30.0584851584089,9.70161662161378));
#2844=CARTESIAN_POINT('Ctrl Pts',(1.95461282093448,-30.433281680772,9.75890828827921));
#2845=CARTESIAN_POINT('Ctrl Pts',(0.813544840407825,-30.8992185370235,9.87349162161376));
#2846=CARTESIAN_POINT('Ctrl Pts',(0.183559280048123,-30.9898636996832,9.9307832882798));
#2847=CARTESIAN_POINT('Ctrl Pts',(-1.04928683050202,-30.8622106788589,10.0453666216132));
#2848=CARTESIAN_POINT('Ctrl Pts',(-1.65096278065817,-30.64398134179,10.1026582882799));
#2849=CARTESIAN_POINT('Ctrl Pts',(-2.68380300579906,-29.9464049512814,10.217241621613));
#2850=CARTESIAN_POINT('Ctrl Pts',(-3.11394951761039,-29.4676807019775,10.2745332882801));
#2851=CARTESIAN_POINT('Ctrl Pts',(-3.69925357053573,-28.3595050698848,10.3891166216128));
#2852=CARTESIAN_POINT('Ctrl Pts',(-3.85380399801319,-27.7310885571697,10.4464082882783));
#2853=CARTESIAN_POINT('Ctrl Pts',(-3.85070485496413,-27.101018442572,10.5036999549465));
#2854=CARTESIAN_POINT('Ctrl Pts',(-3.5,-27.1131792176833,-0.497516612035131));
#2855=CARTESIAN_POINT('Ctrl Pts',(-3.49889065922935,-26.5404930476192,-0.440224945368445));
#2856=CARTESIAN_POINT('Ctrl Pts',(-3.3544424268553,-25.9668059432703,-0.382933278701826));
#2857=CARTESIAN_POINT('Ctrl Pts',(-2.80930542349117,-24.951632956913,-0.268349945368436));
#2858=CARTESIAN_POINT('Ctrl Pts',(-2.40909092606461,-24.5111434366068,-0.211058278701791));
#2859=CARTESIAN_POINT('Ctrl Pts',(-1.4440315356738,-23.8689797539743,-0.0964749453684705));
#2860=CARTESIAN_POINT('Ctrl Pts',(-0.880080083275105,-23.6679643912945,
-0.0391832787017875));
#2861=CARTESIAN_POINT('Ctrl Pts',(0.280613059838117,-23.5558755121778,0.0754000546315256));
#2862=CARTESIAN_POINT('Ctrl Pts',(0.876249675472422,-23.6449624877681,0.132691721298213));
#2863=CARTESIAN_POINT('Ctrl Pts',(1.95910840913653,-24.0958987456423,0.247275054631525));
#2864=CARTESIAN_POINT('Ctrl Pts',(2.44527417877255,-24.4573661122303,0.304566721298234));
#2865=CARTESIAN_POINT('Ctrl Pts',(3.19208164797187,-25.370850975575,0.419150054631504));
#2866=CARTESIAN_POINT('Ctrl Pts',(3.45196757401249,-25.9220285865551,0.476441721298107));
#2867=CARTESIAN_POINT('Ctrl Pts',(3.68132649800696,-27.086466352565,0.591025054631631));
#2868=CARTESIAN_POINT('Ctrl Pts',(3.65052759374337,-27.6986230455641,0.648316721298202));
#2869=CARTESIAN_POINT('Ctrl Pts',(3.30188719744899,-28.840293280662,0.762900054631536));
#2870=CARTESIAN_POINT('Ctrl Pts',(2.98432799528007,-29.3686991601337,0.820191721298178));
#2871=CARTESIAN_POINT('Ctrl Pts',(2.13379161736112,-30.2160978476585,0.93477505463156));
#2872=CARTESIAN_POINT('Ctrl Pts',(1.60159021920541,-30.5342421833904,0.992066721298095));
#2873=CARTESIAN_POINT('Ctrl Pts',(0.445414365419992,-30.8826457776052,1.10665005463164));
#2874=CARTESIAN_POINT('Ctrl Pts',(-0.177469626200369,-30.9125205315103,
1.16394172129828));
#2875=CARTESIAN_POINT('Ctrl Pts',(-1.36813545072923,-30.673420224889,1.27852505463146));
#2876=CARTESIAN_POINT('Ctrl Pts',(-1.93476784632414,-30.4046213916764,1.33581672129817));
#2877=CARTESIAN_POINT('Ctrl Pts',(-2.87746876656431,-29.6280965564544,1.45040005463156));
#2878=CARTESIAN_POINT('Ctrl Pts',(-3.25260154395457,-29.1210720052738,1.50769172129813));
#2879=CARTESIAN_POINT('Ctrl Pts',(-3.72058112180538,-27.9854716656758,1.62227505463161));
#2880=CARTESIAN_POINT('Ctrl Pts',(-3.81293080022416,-27.3579617136213,1.67956672129819));
#2881=CARTESIAN_POINT('Ctrl Pts',(-3.68965672710377,-26.1289746995567,1.79415005463154));
#2882=CARTESIAN_POINT('Ctrl Pts',(-3.47409763241299,-25.5286785378583,1.85144172129826));
#2883=CARTESIAN_POINT('Ctrl Pts',(-2.7822022944777,-24.4971775102941,1.96602505463148));
#2884=CARTESIAN_POINT('Ctrl Pts',(-2.30648341649853,-24.0669891197329,2.02331672129817));
#2885=CARTESIAN_POINT('Ctrl Pts',(-1.20394931882625,-23.4801881039745,2.13790005463157));
#2886=CARTESIAN_POINT('Ctrl Pts',(-0.578163556381753,-23.3241840203502,
2.19519172129821));
#2887=CARTESIAN_POINT('Ctrl Pts',(0.677706928819897,-23.3264027024885,2.30977505463153));
#2888=CARTESIAN_POINT('Ctrl Pts',(1.30659028017156,-23.4846768712254,2.36706672129824));
#2889=CARTESIAN_POINT('Ctrl Pts',(2.4192139548323,-24.0819023526662,2.4816500546315));
#2890=CARTESIAN_POINT('Ctrl Pts',(2.90186470540991,-24.520329561822,2.53894172129796));
#2891=CARTESIAN_POINT('Ctrl Pts',(3.60541788369249,-25.5772648251282,2.65352505463178));
#2892=CARTESIAN_POINT('Ctrl Pts',(3.82560278426285,-26.1947915469424,2.71081672129833));
#2893=CARTESIAN_POINT('Ctrl Pts',(3.94852237831892,-27.4654507839756,2.82540005463141));
#2894=CARTESIAN_POINT('Ctrl Pts',(3.85108621864684,-28.1173730265607,2.88269172129792));
#2895=CARTESIAN_POINT('Ctrl Pts',(3.35786414074355,-29.3023187604958,2.99727505463182));
#2896=CARTESIAN_POINT('Ctrl Pts',(2.96250059030193,-29.8341882432863,3.05456672129825));
#2897=CARTESIAN_POINT('Ctrl Pts',(1.96359948429421,-30.6510950112551,3.16915005463148));
#2898=CARTESIAN_POINT('Ctrl Pts',(1.36098352674217,-30.93530946333,3.22644172129821));
#2899=CARTESIAN_POINT('Ctrl Pts',(0.0881707793306293,-31.186225511463,3.34102505463152));
#2900=CARTESIAN_POINT('Ctrl Pts',(-0.580818873102875,-31.1526345829163,
3.39831672129799));
#2901=CARTESIAN_POINT('Ctrl Pts',(-1.82822926680315,-30.7719182602131,3.51290005463175));
#2902=CARTESIAN_POINT('Ctrl Pts',(-2.40544119057821,-30.4251058408366,3.57019172129822));
#2903=CARTESIAN_POINT('Ctrl Pts',(-3.33097388542638,-29.4964354556262,3.68477505463152));
#2904=CARTESIAN_POINT('Ctrl Pts',(-3.67837143832636,-28.9154280131467,3.74206672129809));
#2905=CARTESIAN_POINT('Ctrl Pts',(-4.05885095899697,-27.6535120007677,3.85665005463164));
#2906=CARTESIAN_POINT('Ctrl Pts',(-4.09151773713705,-26.9737950497155,3.91394172129795));
#2907=CARTESIAN_POINT('Ctrl Pts',(-3.83086030642645,-25.6747542437711,4.02852505463178));
#2908=CARTESIAN_POINT('Ctrl Pts',(-3.53773294713309,-25.0566835016172,4.08581672129817));
#2909=CARTESIAN_POINT('Ctrl Pts',(-2.69110881318515,-24.0285663387021,4.20040005463157));
#2910=CARTESIAN_POINT('Ctrl Pts',(-2.13838054880758,-23.6195373774773,4.25769172129816));
#2911=CARTESIAN_POINT('Ctrl Pts',(-0.900693208979911,-23.1092719795712,
4.37227505463158));
#2912=CARTESIAN_POINT('Ctrl Pts',(-0.216897629946524,-23.0085731171096,
4.42956672129816));
#2913=CARTESIAN_POINT('Ctrl Pts',(1.12205547802317,-23.1426779051177,4.54415005463158));
#2914=CARTESIAN_POINT('Ctrl Pts',(1.77592690914455,-23.377406537751,4.60144172129823));
#2915=CARTESIAN_POINT('Ctrl Pts',(2.89930380962407,-24.1306913712844,4.71602505463151));
#2916=CARTESIAN_POINT('Ctrl Pts',(3.36770491189876,-24.6485714795865,4.77331672129828));
#2917=CARTESIAN_POINT('Ctrl Pts',(4.00659440576528,-25.8485562655112,4.88790005463146));
#2918=CARTESIAN_POINT('Ctrl Pts',(4.17642442602432,-26.5295382611225,4.94519172129826));
#2919=CARTESIAN_POINT('Ctrl Pts',(4.17420574390762,-27.8959069191205,5.05977505463148));
#2920=CARTESIAN_POINT('Ctrl Pts',(4.00210563848955,-28.579986503623,5.117066721298));
#2921=CARTESIAN_POINT('Ctrl Pts',(3.35279167899019,-29.790060866568,5.23165005463174));
#2922=CARTESIAN_POINT('Ctrl Pts',(2.87615175807469,-30.3148728474364,5.28894172129792));
#2923=CARTESIAN_POINT('Ctrl Pts',(1.72734062189585,-31.0798155213496,5.40352505463181));
#2924=CARTESIAN_POINT('Ctrl Pts',(1.0562386306333,-31.319169959825,5.46081672129828));
#2925=CARTESIAN_POINT('Ctrl Pts',(-0.324386700297064,-31.4529202688109,
5.57540005463146));
#2926=CARTESIAN_POINT('Ctrl Pts',(-1.03259456986735,-31.3471349250583,5.63269172129805));
#2927=CARTESIAN_POINT('Ctrl Pts',(-2.3196273040273,-30.8116270271329,5.74727505463168));
#2928=CARTESIAN_POINT('Ctrl Pts',(-2.89720050000837,-30.3823672928139,5.80456672129819));
#2929=CARTESIAN_POINT('Ctrl Pts',(-3.78420656672073,-29.2980499441837,5.91915005463154));
#2930=CARTESIAN_POINT('Ctrl Pts',(-4.0927495448434,-28.643995640032,5.97644172129792));
#2931=CARTESIAN_POINT('Ctrl Pts',(-4.36522271711388,-27.2628079112337,6.09102505463182));
#2932=CARTESIAN_POINT('Ctrl Pts',(-4.32883976428306,-26.5369852993421,6.14831672129839));
#2933=CARTESIAN_POINT('Ctrl Pts',(-3.91604751517395,-25.183834747072,6.26290005463135));
#2934=CARTESIAN_POINT('Ctrl Pts',(-3.5399818785771,-24.5578167789666,6.32019172129842));
#2935=CARTESIAN_POINT('Ctrl Pts',(-2.53317748609787,-23.5541500768163,6.43477505463132));
#2936=CARTESIAN_POINT('Ctrl Pts',(-1.90336399926294,-23.1774993067315,6.49206672129798));
#2937=CARTESIAN_POINT('Ctrl Pts',(-0.535707828330981,-22.7649438596174,
6.60665005463175));
#2938=CARTESIAN_POINT('Ctrl Pts',(0.20084208219242,-22.7294850572333,6.66394172129835));
#2939=CARTESIAN_POINT('Ctrl Pts',(1.6082578695142,-23.011699612039,6.77852505463139));
#2940=CARTESIAN_POINT('Ctrl Pts',(2.27776695825421,-23.3291554974211,6.8358167212985));
#2941=CARTESIAN_POINT('Ctrl Pts',(3.39130036382811,-24.2458789300732,6.95040005463124));
#2942=CARTESIAN_POINT('Ctrl Pts',(3.83422550889456,-24.8443109076698,7.00769172129807));
#2943=CARTESIAN_POINT('Ctrl Pts',(4.38677672685788,-26.1840852477049,7.12227505463167));
#2944=CARTESIAN_POINT('Ctrl Pts',(4.49582477336048,-26.9241664537426,7.17956672129841));
#2945=CARTESIAN_POINT('Ctrl Pts',(4.35088927046636,-28.3730856555887,7.29415005463133));
#2946=CARTESIAN_POINT('Ctrl Pts',(4.09699109987682,-29.0805323561617,7.35144172129841));
#2947=CARTESIAN_POINT('Ctrl Pts',(3.2823167707711,-30.295785129528,7.46602505463132));
#2948=CARTESIAN_POINT('Ctrl Pts',(2.72227543212691,-30.8023989435457,7.52331672129839));
#2949=CARTESIAN_POINT('Ctrl Pts',(1.42483995796224,-31.4933769154898,7.63790005463135));
#2950=CARTESIAN_POINT('Ctrl Pts',(0.688661729169898,-31.6770328723976,7.69519172129708));
#2951=CARTESIAN_POINT('Ctrl Pts',(-0.788205101608382,-31.674814190305,7.80977505463266));
#2952=CARTESIAN_POINT('Ctrl Pts',(-1.52748091929412,-31.4888881482022,7.8670667212985));
#2953=CARTESIAN_POINT('Ctrl Pts',(-2.8350059704747,-30.7874857106489,7.98165005463124));
#2954=CARTESIAN_POINT('Ctrl Pts',(-3.40197918167132,-30.2726330779668,8.03894172129796));
#2955=CARTESIAN_POINT('Ctrl Pts',(-4.22831135118872,-29.0319460689245,8.15352505463178));
#2956=CARTESIAN_POINT('Ctrl Pts',(-4.48683532758525,-28.3072688081897,8.21081672129796));
#2957=CARTESIAN_POINT('Ctrl Pts',(-4.63141635149551,-26.8166773834008,8.32540005463178));
#2958=CARTESIAN_POINT('Ctrl Pts',(-4.51728182365347,-26.0521838868123,8.38269172129824));
#2959=CARTESIAN_POINT('Ctrl Pts',(-3.93948810572916,-24.6630641524548,8.4972750546315));
#2960=CARTESIAN_POINT('Ctrl Pts',(-3.47633218752115,-24.0397872432635,8.55456672129809));
#2961=CARTESIAN_POINT('Ctrl Pts',(-2.30659859626835,-23.0826818778197,8.66915005463165));
#2962=CARTESIAN_POINT('Ctrl Pts',(-1.60110594549963,-22.7498103736324,8.72644172129807));
#2963=CARTESIAN_POINT('Ctrl Pts',(-0.111543235349543,-22.455780077246,8.84102505463166));
#2964=CARTESIAN_POINT('Ctrl Pts',(0.671112336026933,-22.4949550543515,8.89831672129782));
#2965=CARTESIAN_POINT('Ctrl Pts',(2.13000304684827,-22.9398232298639,9.01290005463192));
#2966=CARTESIAN_POINT('Ctrl Pts',(2.80482705930729,-23.3451420836895,9.07019172129816));
#2967=CARTESIAN_POINT('Ctrl Pts',(3.88662776873158,-24.4300804834233,9.18477505463157));
#2968=CARTESIAN_POINT('Ctrl Pts',(4.292531756023,-25.1087000146355,9.24206672129765));
#2969=CARTESIAN_POINT('Ctrl Pts',(4.73716312956515,-26.582096344091,9.35665005463209));
#2970=CARTESIAN_POINT('Ctrl Pts',(4.77541395619357,-27.3754792141155,9.4139417212973));
#2971=CARTESIAN_POINT('Ctrl Pts',(4.47164227730762,-28.8912699827844,9.52852505463244));
#2972=CARTESIAN_POINT('Ctrl Pts',(4.12985786582675,-29.6122174181468,9.58581672129757));
#2973=CARTESIAN_POINT('Ctrl Pts',(3.14303513447574,-30.8111670663372,9.70040005463217));
#2974=CARTESIAN_POINT('Ctrl Pts',(2.49889944364267,-31.2879883952817,9.7576917212976));
#2975=CARTESIAN_POINT('Ctrl Pts',(1.05703810342987,-31.8828254332717,9.87227505463214));
#2976=CARTESIAN_POINT('Ctrl Pts',(0.260671270356948,-32.0002226638335,9.92956672129819));
#2977=CARTESIAN_POINT('Ctrl Pts',(-1.29821402533356,-31.8444564460475,10.0441500546315));
#2978=CARTESIAN_POINT('Ctrl Pts',(-2.05923599538643,-31.5713887375034,10.1014417212983));
#2979=CARTESIAN_POINT('Ctrl Pts',(-3.3663646416149,-30.6953249128279,10.2160250546314));
#2980=CARTESIAN_POINT('Ctrl Pts',(-3.91119116738902,-30.0931223438177,10.2733167212985));
#2981=CARTESIAN_POINT('Ctrl Pts',(-4.65425761740862,-28.6982361814583,10.3879000546312));
#2982=CARTESIAN_POINT('Ctrl Pts',(-4.85173951078678,-27.9068617309244,10.4451917212967));
#2983=CARTESIAN_POINT('Ctrl Pts',(-4.85063016993195,-27.113179217683,10.5024833879649));
#2984=CARTESIAN_POINT('Ctrl Pts',(-4.49992140627864,-27.1253399452581,-0.498733174261208));
#2985=CARTESIAN_POINT('Ctrl Pts',(-4.50080185993612,-26.3890420150452,-0.441441507594522));
#2986=CARTESIAN_POINT('Ctrl Pts',(-4.31739811102725,-25.6514017289714,-0.384149840927902));
#2987=CARTESIAN_POINT('Ctrl Pts',(-3.62151869566008,-24.3457674036837,-0.269566507594513));
#2988=CARTESIAN_POINT('Ctrl Pts',(-3.10966150316856,-23.7790475859312,-0.212274840927868));
#2989=CARTESIAN_POINT('Ctrl Pts',(-1.87473664682874,-22.9517793531317,-0.0976915075945471));
#2990=CARTESIAN_POINT('Ctrl Pts',(-1.15282057736006,-22.6920668090806,-0.0403998409278641));
#2991=CARTESIAN_POINT('Ctrl Pts',(0.333130339632276,-22.543943991072,0.074183492405449));
#2992=CARTESIAN_POINT('Ctrl Pts',(1.09574896981128,-22.6557286792713,0.131475159072136));
#2993=CARTESIAN_POINT('Ctrl Pts',(2.48244573188416,-23.2282112934409,0.246058492405449));
#2994=CARTESIAN_POINT('Ctrl Pts',(3.10517686323593,-23.6884110321826,0.303350159072158));
#2995=CARTESIAN_POINT('Ctrl Pts',(4.06264899488962,-24.8523184668817,0.417933492405427));
#2996=CARTESIAN_POINT('Ctrl Pts',(4.39643269933883,-25.5549467222002,0.475225159072031));
#2997=CARTESIAN_POINT('Ctrl Pts',(4.69353288583996,-27.0395441134278,0.589808492405554));
#2998=CARTESIAN_POINT('Ctrl Pts',(4.65651266421214,-27.8201035217474,0.647100159072126));
#2999=CARTESIAN_POINT('Ctrl Pts',(4.21669252519888,-29.2760623484253,0.761683492405459));
#3000=CARTESIAN_POINT('Ctrl Pts',(3.81426212049019,-29.9500534547892,0.818975159072102));
#3001=CARTESIAN_POINT('Ctrl Pts',(2.735157772082,-31.0316481012048,0.933558492405483));
#3002=CARTESIAN_POINT('Ctrl Pts',(2.05947825480693,-31.4381791363691,0.990850159072061));
#3003=CARTESIAN_POINT('Ctrl Pts',(0.591324236677636,-31.8853789313282,1.10543349240552));
#3004=CARTESIAN_POINT('Ctrl Pts',(-0.199761360833674,-31.9255686777873,
1.1627251590722));
#3005=CARTESIAN_POINT('Ctrl Pts',(-1.71213956917068,-31.6265333528055,1.27730849240538));
#3006=CARTESIAN_POINT('Ctrl Pts',(-2.43197499151047,-31.2875418427295,1.3346001590721));
#3007=CARTESIAN_POINT('Ctrl Pts',(-3.63014773197565,-30.3065048723984,1.44918349240549));
#3008=CARTESIAN_POINT('Ctrl Pts',(-4.10730491757991,-29.66535650003,1.50647515907205));
#3009=CARTESIAN_POINT('Ctrl Pts',(-4.70418417300477,-28.2289639772332,1.62105849240553));
#3010=CARTESIAN_POINT('Ctrl Pts',(-4.8232858148679,-27.4350734021293,1.67835015907212));
#3011=CARTESIAN_POINT('Ctrl Pts',(-4.67189865474462,-25.8800484781485,1.79293349240547));
#3012=CARTESIAN_POINT('Ctrl Pts',(-4.40150140270865,-25.1204069187536,1.85022515907218));
#3013=CARTESIAN_POINT('Ctrl Pts',(-3.53111932870988,-23.8146185429076,1.9648084924054));
#3014=CARTESIAN_POINT('Ctrl Pts',(-2.93192261318194,-23.2697505861832,2.022100159072));
#3015=CARTESIAN_POINT('Ctrl Pts',(-1.54267910662356,-22.5251877903681,2.13668349240558));
#3016=CARTESIAN_POINT('Ctrl Pts',(-0.753936040316516,-22.3262524084538,
2.19397515907222));
#3017=CARTESIAN_POINT('Ctrl Pts',(0.829157957605105,-22.3244915018276,2.30855849240537));
#3018=CARTESIAN_POINT('Ctrl Pts',(1.62199449431653,-22.5217211869735,2.36585015907225));
#3019=CARTESIAN_POINT('Ctrl Pts',(3.02507950821547,-23.2696890805772,2.48043349240533));
#3020=CARTESIAN_POINT('Ctrl Pts',(3.63396055598865,-23.8197589845765,2.53772515907179));
#3021=CARTESIAN_POINT('Ctrl Pts',(4.52261828463197,-25.1465597141148,2.65230849240579));
#3022=CARTESIAN_POINT('Ctrl Pts',(4.80150036645811,-25.9220510526903,2.70960015907225));
#3023=CARTESIAN_POINT('Ctrl Pts',(4.96045389944342,-27.5179680639369,2.82418349240533));
#3024=CARTESIAN_POINT('Ctrl Pts',(4.84032002720497,-28.3368723207458,2.88147515907176));
#3025=CARTESIAN_POINT('Ctrl Pts',(4.22555159288363,-29.8256560833971,2.99605849240583));
#3026=CARTESIAN_POINT('Ctrl Pts',(3.73145567047586,-30.4940909276437,3.05335015907218));
#3027=CARTESIAN_POINT('Ctrl Pts',(2.48213199286114,-31.5216623582789,3.16793349240541));
#3028=CARTESIAN_POINT('Ctrl Pts',(1.7280653912543,-31.8797745886219,3.22522515907214));
#3029=CARTESIAN_POINT('Ctrl Pts',(0.135093018310607,-32.1984318993305,3.33980849240545));
#3030=CARTESIAN_POINT('Ctrl Pts',(-0.702299349132642,-32.1586196534296,
3.39710015907191));
#3031=CARTESIAN_POINT('Ctrl Pts',(-2.26399833471994,-31.6867235879184,3.51168349240567));
#3032=CARTESIAN_POINT('Ctrl Pts',(-2.98679548512054,-31.2550399661564,3.56897515907214));
#3033=CARTESIAN_POINT('Ctrl Pts',(-4.14652413908592,-30.0978016102373,3.68355849240545));
#3034=CARTESIAN_POINT('Ctrl Pts',(-4.58230839125774,-29.3733160488965,3.74085015907202));
#3035=CARTESIAN_POINT('Ctrl Pts',(-5.06158411276736,-27.799421871877,3.85543349240557));
#3036=CARTESIAN_POINT('Ctrl Pts',(-5.10456588344323,-26.9515033152352,3.91272515907188));
#3037=CARTESIAN_POINT('Ctrl Pts',(-4.78397343431367,-25.3307501251766,4.02730849240571));
#3038=CARTESIAN_POINT('Ctrl Pts',(-4.42065339828102,-24.5594763565493,4.08460015907228));
#3039=CARTESIAN_POINT('Ctrl Pts',(-3.36951712903428,-23.2758873731723,4.19918349240531));
#3040=CARTESIAN_POINT('Ctrl Pts',(-2.68266504370096,-22.7648340039114,4.25647515907209));
#3041=CARTESIAN_POINT('Ctrl Pts',(-1.14418552040014,-22.1256689283123,4.3710584924055));
#3042=CARTESIAN_POINT('Ctrl Pts',(-0.2940093186021,-21.9982181024529,4.42835015907226));
#3043=CARTESIAN_POINT('Ctrl Pts',(1.370981699579,-22.1604359774898,4.54293349240532));
#3044=CARTESIAN_POINT('Ctrl Pts',(2.18419852812648,-22.4500027673754,4.60022515907215));
#3045=CARTESIAN_POINT('Ctrl Pts',(3.58186277713337,-23.3817743371321,4.71480849240544));
#3046=CARTESIAN_POINT('Ctrl Pts',(4.16494344537974,-24.0231322827754,4.77210015907202));
#3047=CARTESIAN_POINT('Ctrl Pts',(4.96159471944044,-25.5098264778416,4.88668349240556));
#3048=CARTESIAN_POINT('Ctrl Pts',(5.17435603791885,-26.3537657770459,4.94397515907237));
#3049=CARTESIAN_POINT('Ctrl Pts',(5.17611694457037,-28.0473579480475,5.05855849240522));
#3050=CARTESIAN_POINT('Ctrl Pts',(4.96506132280656,-28.8953907176428,5.11585015907192));
#3051=CARTESIAN_POINT('Ctrl Pts',(4.16500495101401,-30.3959264200764,5.23043349240566));
#3052=CARTESIAN_POINT('Ctrl Pts',(3.57672233543479,-31.0469686979372,5.28772515907185));
#3053=CARTESIAN_POINT('Ctrl Pts',(2.15804573279459,-31.997015922367,5.40230849240574));
#3054=CARTESIAN_POINT('Ctrl Pts',(1.32897912502245,-32.2950675420036,5.45960015907202));
#3055=CARTESIAN_POINT('Ctrl Pts',(-0.376903980395488,-32.4648517899521,
5.57418349240557));
#3056=CARTESIAN_POINT('Ctrl Pts',(-1.25209386392467,-32.3363687336658,5.63147515907217));
#3057=CARTESIAN_POINT('Ctrl Pts',(-2.84296462705654,-31.6793144792236,5.74605849240542));
#3058=CARTESIAN_POINT('Ctrl Pts',(-3.55710318428054,-31.1513223730886,5.80335015907193));
#3059=CARTESIAN_POINT('Ctrl Pts',(-4.65477391382974,-29.8165824526497,5.91793349240566));
#3060=CARTESIAN_POINT('Ctrl Pts',(-5.03721467010861,-29.0110775046754,5.97522515907185));
#3061=CARTESIAN_POINT('Ctrl Pts',(-5.37742910500803,-27.3097301500823,6.08980849240574));
#3062=CARTESIAN_POINT('Ctrl Pts',(-5.334824834833,-26.4155048234392,6.1471001590725));
#3063=CARTESIAN_POINT('Ctrl Pts',(-4.83085284284264,-24.7480656790283,6.26168349240508));
#3064=CARTESIAN_POINT('Ctrl Pts',(-4.36991600398824,-23.9764624845173,6.31897515907215));
#3065=CARTESIAN_POINT('Ctrl Pts',(-3.13454364061771,-22.7385998230638,6.43355849240543));
#3066=CARTESIAN_POINT('Ctrl Pts',(-2.36125203513461,-22.2735623538381,6.4908501590721));
#3067=CARTESIAN_POINT('Ctrl Pts',(-0.681617699318414,-21.762210705809,6.60543349240548));
#3068=CARTESIAN_POINT('Ctrl Pts',(0.223133816549338,-21.716436910903,6.66272515907227));
#3069=CARTESIAN_POINT('Ctrl Pts',(1.95226198823211,-22.0585864841759,6.77730849240531));
#3070=CARTESIAN_POINT('Ctrl Pts',(2.77497410322413,-22.4462350461933,6.83460015907242));
#3071=CARTESIAN_POINT('Ctrl Pts',(4.14397932945591,-23.5674706143039,6.94918349240517));
#3072=CARTESIAN_POINT('Ctrl Pts',(4.68892888241214,-24.3000264126609,7.006475159072));
#3073=CARTESIAN_POINT('Ctrl Pts',(5.37037977816506,-25.9405929364001,7.12105849240559));
#3074=CARTESIAN_POINT('Ctrl Pts',(5.50617978802718,-26.847054764966,7.17835015907233));
#3075=CARTESIAN_POINT('Ctrl Pts',(5.33313119808424,-28.6220118772656,7.29293349240526));
#3076=CARTESIAN_POINT('Ctrl Pts',(5.02439487031729,-29.4888039750442,7.35022515907234));
#3077=CARTESIAN_POINT('Ctrl Pts',(4.03123380485844,-30.9783440971367,7.46480849240525));
#3078=CARTESIAN_POINT('Ctrl Pts',(3.34771462904399,-31.5996374769677,7.52210015907212));
#3079=CARTESIAN_POINT('Ctrl Pts',(1.76356974552581,-32.448377229224,7.63668349240547));
#3080=CARTESIAN_POINT('Ctrl Pts',(0.864434213366158,-32.6749644842892,7.6939751590712));
#3081=CARTESIAN_POINT('Ctrl Pts',(-0.939656130655156,-32.6767253909707,
7.80855849240638));
#3082=CARTESIAN_POINT('Ctrl Pts',(-1.84288513321169,-32.4518438325729,7.86585015907242));
#3083=CARTESIAN_POINT('Ctrl Pts',(-3.44087152408535,-31.5996989826189,7.98043349240516));
#3084=CARTESIAN_POINT('Ctrl Pts',(-4.13407503210608,-30.9732036554222,8.03772515907188));
#3085=CARTESIAN_POINT('Ctrl Pts',(-5.14551175227223,-29.4626511797278,8.1523084924057));
#3086=CARTESIAN_POINT('Ctrl Pts',(-5.46273290975301,-28.5800093026908,8.20960015907188));
#3087=CARTESIAN_POINT('Ctrl Pts',(-5.64334787264751,-26.7641601031904,8.3241834924057));
#3088=CARTESIAN_POINT('Ctrl Pts',(-5.50651563230342,-25.8326845928579,8.38147515907216));
#3089=CARTESIAN_POINT('Ctrl Pts',(-4.8071755577774,-24.1397268293227,8.49605849240542));
#3090=CARTESIAN_POINT('Ctrl Pts',(-4.24528726788241,-23.3798845590642,8.55335015907201));
#3091=CARTESIAN_POINT('Ctrl Pts',(-2.8251311046479,-22.2121145306378,8.66793349240557));
#3092=CARTESIAN_POINT('Ctrl Pts',(-1.96818781025068,-21.8053452483902,8.72522515907199));
#3093=CARTESIAN_POINT('Ctrl Pts',(-0.158465474090509,-21.4435736893289,
8.83980849240559));
#3094=CARTESIAN_POINT('Ctrl Pts',(0.792592811825796,-21.4889699837715,8.89710015907174));
#3095=CARTESIAN_POINT('Ctrl Pts',(2.56577211499604,-22.0250179022253,9.01168349240585));
#3096=CARTESIAN_POINT('Ctrl Pts',(3.38618135368034,-22.5152079582028,9.06897515907209));
#3097=CARTESIAN_POINT('Ctrl Pts',(4.70217802256045,-23.8287143289791,9.1835584924055));
#3098=CARTESIAN_POINT('Ctrl Pts',(5.19646870888364,-24.6508119786607,9.24085015907157));
#3099=CARTESIAN_POINT('Ctrl Pts',(5.7398962834063,-26.4361864732067,9.35543349240601));
#3100=CARTESIAN_POINT('Ctrl Pts',(5.78846210254197,-27.3977709483694,9.41272515907122));
#3101=CARTESIAN_POINT('Ctrl Pts',(5.42475540515261,-29.2352741016053,9.52730849240636));
#3102=CARTESIAN_POINT('Ctrl Pts',(5.01277831711823,-30.1094245630356,9.58460015907149));
#3103=CARTESIAN_POINT('Ctrl Pts',(3.82144345018127,-31.5638460320461,9.69918349240609));
#3104=CARTESIAN_POINT('Ctrl Pts',(3.04318393874474,-32.142691768759,9.75647515907152));
#3105=CARTESIAN_POINT('Ctrl Pts',(1.30053041464135,-32.8664284846192,9.87105849240607));
#3106=CARTESIAN_POINT('Ctrl Pts',(0.337782959236464,-33.0105776785097,9.92835015907211));
#3107=CARTESIAN_POINT('Ctrl Pts',(-1.54714024711339,-32.8266983736559,10.0429334924055));
#3108=CARTESIAN_POINT('Ctrl Pts',(-2.46750761418241,-32.4987925079987,10.1002251590722));
#3109=CARTESIAN_POINT('Ctrl Pts',(-4.0489236093102,-31.4442419468603,10.2148084924053));
#3110=CARTESIAN_POINT('Ctrl Pts',(-4.7084297007651,-30.7185615408183,10.2721001590725));
#3111=CARTESIAN_POINT('Ctrl Pts',(-5.60925793118873,-29.0369659689382,10.3866834924051));
#3112=CARTESIAN_POINT('Ctrl Pts',(-5.8496711226493,-28.082634217585,10.4439751590706));
#3113=CARTESIAN_POINT('Ctrl Pts',(-5.85055157621059,-27.1253399452577,10.5012668257388));
#3114=CARTESIAN_POINT('Ctrl Pts',(-4.49992531496272,-27.2248831058227,0.496297452001021));
#3115=CARTESIAN_POINT('Ctrl Pts',(-4.5170934804426,-26.4885845360516,0.553589118667707));
#3116=CARTESIAN_POINT('Ctrl Pts',(-4.34996170166829,-25.7468676545126,0.610880785334326));
#3117=CARTESIAN_POINT('Ctrl Pts',(-3.68281064144925,-24.4258762531054,0.725464118667716));
#3118=CARTESIAN_POINT('Ctrl Pts',(-3.18338235197652,-23.8478906453164,0.782755785334401));
#3119=CARTESIAN_POINT('Ctrl Pts',(-1.96655436736188,-22.9935362276632,0.897339118667641));
#3120=CARTESIAN_POINT('Ctrl Pts',(-1.2502889550967,-22.7180291994921,0.954630785334324));
#3121=CARTESIAN_POINT('Ctrl Pts',(0.232470285055687,-22.537487692811,1.06921411866772));
#3122=CARTESIAN_POINT('Ctrl Pts',(0.997550948764801,-22.6326791882398,1.12650578533436));
#3123=CARTESIAN_POINT('Ctrl Pts',(2.39671496721365,-23.1750665254593,1.24108911866768));
#3124=CARTESIAN_POINT('Ctrl Pts',(3.02943939521195,-23.6217929692252,1.29838078533443));
#3125=CARTESIAN_POINT('Ctrl Pts',(4.01209348072769,-24.7650357631989,1.41296411866761));
#3126=CARTESIAN_POINT('Ctrl Pts',(4.36104175327124,-25.4604924406082,1.47025578533422));
#3127=CARTESIAN_POINT('Ctrl Pts',(4.69009168456907,-26.9387359366337,1.58483911866782));
#3128=CARTESIAN_POINT('Ctrl Pts',(4.66982607643029,-27.7201191058137,1.64213078533435));
#3129=CARTESIAN_POINT('Ctrl Pts',(4.26117830221042,-29.18553530264,1.75671411866769));
#3130=CARTESIAN_POINT('Ctrl Pts',(3.87313582923077,-29.8681509713484,1.81400578533433));
#3131=CARTESIAN_POINT('Ctrl Pts',(2.81706487876742,-30.9727808246477,1.92858911866771));
#3132=CARTESIAN_POINT('Ctrl Pts',(2.15000879388831,-31.3937004688027,1.98588078533433));
#3133=CARTESIAN_POINT('Ctrl Pts',(0.691309697839529,-31.8720733711749,2.10046411866771));
#3134=CARTESIAN_POINT('Ctrl Pts',(-0.0989534545953723,-31.9290177957557,
2.15775578533426));
#3135=CARTESIAN_POINT('Ctrl Pts',(-1.61768806720869,-31.6619317164947,2.27233911866778));
#3136=CARTESIAN_POINT('Ctrl Pts',(-2.34469625833983,-31.3381042112553,2.32963078533433));
#3137=CARTESIAN_POINT('Ctrl Pts',(-3.56353561707773,-30.3822475718731,2.44421411866772));
#3138=CARTESIAN_POINT('Ctrl Pts',(-4.05416688239932,-29.7510914380183,2.50150578533428));
#3139=CARTESIAN_POINT('Ctrl Pts',(-4.68114239378513,-28.3271638081165,2.61608911866776));
#3140=CARTESIAN_POINT('Ctrl Pts',(-4.81683742169616,-27.5357339634246,2.67338078533435));
#3141=CARTESIAN_POINT('Ctrl Pts',(-4.69786869951757,-25.9775148166942,2.7879641186677));
#3142=CARTESIAN_POINT('Ctrl Pts',(-4.44326548776946,-25.212221359738,2.84525578533441));
#3143=CARTESIAN_POINT('Ctrl Pts',(-3.59996817737392,-23.8883339850702,2.95983911866763));
#3144=CARTESIAN_POINT('Ctrl Pts',(-3.01203627575868,-23.3310362406515,3.01713078533432));
#3145=CARTESIAN_POINT('Ctrl Pts',(-1.6381475891734,-22.5577438837235,3.13171411866773));
#3146=CARTESIAN_POINT('Ctrl Pts',(-0.853479840438057,-22.3425362112162,
3.18900578533436));
#3147=CARTESIAN_POINT('Ctrl Pts',(0.72961543659743,-22.3081998816971,3.30358911866768));
#3148=CARTESIAN_POINT('Ctrl Pts',(1.52652856876947,-22.4891575963454,3.3608807853344));
#3149=CARTESIAN_POINT('Ctrl Pts',(2.94497065879964,-23.2083971347751,3.47546411866765));
#3150=CARTESIAN_POINT('Ctrl Pts',(3.56511749658876,-23.7460381357776,3.5327557853342));
#3151=CARTESIAN_POINT('Ctrl Pts',(4.48086141011516,-25.0547419935726,3.64733911866784));
#3152=CARTESIAN_POINT('Ctrl Pts',(4.77553797602982,-25.8245826749535,3.70463078533439));
#3153=CARTESIAN_POINT('Ctrl Pts',(4.96691019772129,-27.4173080093605,3.81921411866765));
#3154=CARTESIAN_POINT('Ctrl Pts',(4.86336951822156,-28.2386742996913,3.87650578533407));
#3155=CARTESIAN_POINT('Ctrl Pts',(4.27869636088015,-29.7399253187347,3.99108911866797));
#3156=CARTESIAN_POINT('Ctrl Pts',(3.79807373342137,-30.4183534596066,4.0483807853344));
#3157=CARTESIAN_POINT('Ctrl Pts',(2.56941469655591,-31.4711068441301,4.16296411866764));
#3158=CARTESIAN_POINT('Ctrl Pts',(1.82251967284502,-31.8443836425387,4.22025578533436));
#3159=CARTESIAN_POINT('Ctrl Pts',(0.23590119510592,-32.1949906980752,4.33483911866768));
#3160=CARTESIAN_POINT('Ctrl Pts',(-0.602314933192407,-32.1719330656341,
4.39213078533414));
#3161=CARTESIAN_POINT('Ctrl Pts',(-2.17347128894129,-31.7312093649436,4.5067141186679));
#3162=CARTESIAN_POINT('Ctrl Pts',(-2.9048930016682,-31.313913674884,4.56400578533437));
#3163=CARTESIAN_POINT('Ctrl Pts',(-4.08765686254034,-30.1797087169358,4.67858911866767));
#3164=CARTESIAN_POINT('Ctrl Pts',(-4.53782972367693,-29.4638465879738,4.73588078533424));
#3165=CARTESIAN_POINT('Ctrl Pts',(-5.04827855262831,-27.899407333043,4.8504641186678));
#3166=CARTESIAN_POINT('Ctrl Pts',(-5.10801500139697,-27.0523112214756,4.90775578533411));
#3167=CARTESIAN_POINT('Ctrl Pts',(-4.81937179801766,-25.4252016271365,5.02233911866794));
#3168=CARTESIAN_POINT('Ctrl Pts',(-4.4712157667966,-24.6467550897301,5.07963078533432));
#3169=CARTESIAN_POINT('Ctrl Pts',(-3.44525982851924,-23.3424994880601,5.19421411866772));
#3170=CARTESIAN_POINT('Ctrl Pts',(-2.76839998168555,-22.8179720391072,5.25150578533431));
#3171=CARTESIAN_POINT('Ctrl Pts',(-1.24238535128709,-22.1487107075167,5.36608911866773));
#3172=CARTESIAN_POINT('Ctrl Pts',(-0.394669879900677,-22.0046664956406,
5.42338078533431));
#3173=CARTESIAN_POINT('Ctrl Pts',(1.2735153610365,-22.1344659327008,5.53796411866773));
#3174=CARTESIAN_POINT('Ctrl Pts',(2.09238408713078,-22.4082386823275,5.59525578533438));
#3175=CARTESIAN_POINT('Ctrl Pts',(3.50814733498208,-23.3129254884552,5.70983911866766));
#3176=CARTESIAN_POINT('Ctrl Pts',(4.10365779089971,-23.9430186202042,5.76713078533443));
#3177=CARTESIAN_POINT('Ctrl Pts',(4.92903862609668,-25.4143579952863,5.88171411866761));
#3178=CARTESIAN_POINT('Ctrl Pts',(5.15807223514289,-26.2542219769244,5.93900578533441));
#3179=CARTESIAN_POINT('Ctrl Pts',(5.1924085647145,-27.9478154270399,6.05358911866763));
#3180=CARTESIAN_POINT('Ctrl Pts',(4.99762491342332,-28.7999247920913,6.11088078533415));
#3181=CARTESIAN_POINT('Ctrl Pts',(4.22629689682747,-30.315817570665,6.22546411866789));
#3182=CARTESIAN_POINT('Ctrl Pts',(3.65044318422569,-30.978125638526,6.28275578533408));
#3183=CARTESIAN_POINT('Ctrl Pts',(2.24986345334479,-31.9552590478615,6.39733911866797));
#3184=CARTESIAN_POINT('Ctrl Pts',(1.42644750275535,-32.2691051515638,6.45463078533443));
#3185=CARTESIAN_POINT('Ctrl Pts',(-0.276243925815165,-32.4713080882415,
6.56921411866761));
#3186=CARTESIAN_POINT('Ctrl Pts',(-1.15389584286732,-32.3594182246709,6.62650578533421));
#3187=CARTESIAN_POINT('Ctrl Pts',(-2.75723386239692,-31.7324592472316,6.74108911866784));
#3188=CARTESIAN_POINT('Ctrl Pts',(-3.48136571623396,-31.2179404360269,6.79838078533435));
#3189=CARTESIAN_POINT('Ctrl Pts',(-4.60421839969041,-29.9038651563518,6.9129641186677));
#3190=CARTESIAN_POINT('Ctrl Pts',(-5.00182372401274,-29.1055317862615,6.97025578533408));
#3191=CARTESIAN_POINT('Ctrl Pts',(-5.37398790376543,-27.4105383268823,7.08483911866797));
#3192=CARTESIAN_POINT('Ctrl Pts',(-5.34813824702216,-26.5154892393799,7.14213078533454));
#3193=CARTESIAN_POINT('Ctrl Pts',(-4.87533861988318,-24.8385927248065,7.2567141186675));
#3194=CARTESIAN_POINT('Ctrl Pts',(-4.42878971270738,-24.0583649679817,7.31400578533457));
#3195=CARTESIAN_POINT('Ctrl Pts',(-3.21645074732456,-22.7974670995972,7.42858911866747));
#3196=CARTESIAN_POINT('Ctrl Pts',(-2.45178257420817,-22.3180410214301,7.48588078533414));
#3197=CARTESIAN_POINT('Ctrl Pts',(-0.781603160488131,-21.7755162659369,
7.60046411866791));
#3198=CARTESIAN_POINT('Ctrl Pts',(0.122325910305338,-21.7129877929629,7.6577557853345));
#3199=CARTESIAN_POINT('Ctrl Pts',(1.85781048627581,-22.0231881204583,7.77233911866754));
#3200=CARTESIAN_POINT('Ctrl Pts',(2.68769537003688,-22.3956726776898,7.82963078533388));
#3201=CARTESIAN_POINT('Ctrl Pts',(4.07736721457463,-23.4917279148069,7.94421411866817));
#3202=CARTESIAN_POINT('Ctrl Pts',(4.63579084720592,-24.2142914746826,8.00150578533422));
#3203=CARTESIAN_POINT('Ctrl Pts',(5.34733799897106,-25.842393105507,8.11608911866782));
#3204=CARTESIAN_POINT('Ctrl Pts',(5.49973139482918,-26.7463942036693,8.17338078533455));
#3205=CARTESIAN_POINT('Ctrl Pts',(5.35910124288347,-28.5245455387212,8.28796411866749));
#3206=CARTESIAN_POINT('Ctrl Pts',(5.06615895535571,-29.3969895340438,8.34525578533457));
#3207=CARTESIAN_POINT('Ctrl Pts',(4.10008265354488,-30.9046286549901,8.45983911866747));
#3208=CARTESIAN_POINT('Ctrl Pts',(3.42782829160734,-31.5383518224792,8.51713078533533));
#3209=CARTESIAN_POINT('Ctrl Pts',(1.85903822808905,-32.4158211358887,8.63171411866672));
#3210=CARTESIAN_POINT('Ctrl Pts',(0.9639780134877,-32.6586806815057,8.68900578533323));
#3211=CARTESIAN_POINT('Ctrl Pts',(-0.840113609647483,-32.6930170111224,
8.80358911866881));
#3212=CARTESIAN_POINT('Ctrl Pts',(-1.74741920765194,-32.4844074231763,8.86088078533465));
#3213=CARTESIAN_POINT('Ctrl Pts',(-3.3607626746822,-31.6609909284457,8.97546411866739));
#3214=CARTESIAN_POINT('Ctrl Pts',(-4.06523197268589,-31.0469245042064,9.03275578533411));
#3215=CARTESIAN_POINT('Ctrl Pts',(-5.10375487777573,-29.5544689002848,9.14733911866793));
#3216=CARTESIAN_POINT('Ctrl Pts',(-5.43677051929896,-28.6774776804222,9.20463078533411));
#3217=CARTESIAN_POINT('Ctrl Pts',(-5.64980417095116,-26.8648201577722,9.31921411866793));
#3218=CARTESIAN_POINT('Ctrl Pts',(-5.5295651232969,-25.9308826139232,9.37650578533439));
#3219=CARTESIAN_POINT('Ctrl Pts',(-4.86032032579704,-24.2254575939744,9.49108911866765));
#3220=CARTESIAN_POINT('Ctrl Pts',(-4.31190533081157,-23.4556220271188,9.54838078533424));
#3221=CARTESIAN_POINT('Ctrl Pts',(-2.91241380835902,-22.2626700447691,9.6629641186678));
#3222=CARTESIAN_POINT('Ctrl Pts',(-2.06264209183543,-21.8407361944978,9.72025578533422));
#3223=CARTESIAN_POINT('Ctrl Pts',(-0.259273650891808,-21.4470148905597,
9.83483911866782));
#3224=CARTESIAN_POINT('Ctrl Pts',(0.692608395878797,-21.4756565715901,9.89213078533397));
#3225=CARTESIAN_POINT('Ctrl Pts',(2.47524506922415,-21.9805321251769,10.0067141186681));
#3226=CARTESIAN_POINT('Ctrl Pts',(3.30427887021131,-22.4563342494898,10.0640057853343));
#3227=CARTESIAN_POINT('Ctrl Pts',(4.64331074603158,-23.7468072222661,10.1785891186677));
#3228=CARTESIAN_POINT('Ctrl Pts',(5.15199004128089,-24.5602814395911,10.2358807853338));
#3229=CARTESIAN_POINT('Ctrl Pts',(5.7265907232892,-26.336201012033,10.3504641186682));
#3230=CARTESIAN_POINT('Ctrl Pts',(5.79191122047382,-27.2969630421229,10.4077557853326));
#3231=CARTESIAN_POINT('Ctrl Pts',(5.4601537688785,-29.1408225996516,10.5223391186694));
#3232=CARTESIAN_POINT('Ctrl Pts',(5.06334068561503,-30.0221458298436,10.5796307853337));
#3233=CARTESIAN_POINT('Ctrl Pts',(3.897186149685,-31.4972339171696,10.6942141186683));
#3234=CARTESIAN_POINT('Ctrl Pts',(3.12891887671996,-32.0895537335424,10.7515057853337));
#3235=CARTESIAN_POINT('Ctrl Pts',(1.39873024553766,-32.8433867054356,10.8660891186683));
#3236=CARTESIAN_POINT('Ctrl Pts',(0.438443520536697,-33.0041292853017,10.9233807853343));
#3237=CARTESIAN_POINT('Ctrl Pts',(-1.44967390857254,-32.8526684184651,11.0379641186677));
#3238=CARTESIAN_POINT('Ctrl Pts',(-2.37569317317473,-32.5405565930317,11.0952557853345));
#3239=CARTESIAN_POINT('Ctrl Pts',(-3.97520816717089,-31.5130907955522,11.2098391186676));
#3240=CARTESIAN_POINT('Ctrl Pts',(-4.64714404626587,-30.7986752033783,11.2671307853347));
#3241=CARTESIAN_POINT('Ctrl Pts',(-5.57670183786417,-29.1324344515049,11.3817141186674));
#3242=CARTESIAN_POINT('Ctrl Pts',(-5.83338731961563,-28.1821780177065,11.4390057853329));
#3243=CARTESIAN_POINT('Ctrl Pts',(-5.85055548489467,-27.2248831058223,11.496297452001));
#3244=CARTESIAN_POINT('Ctrl Pts',(-3.50000130290148,-27.2127226059667,0.497516610448255));
#3245=CARTESIAN_POINT('Ctrl Pts',(-3.51517971121378,-26.6400362227171,0.554808277114941));
#3246=CARTESIAN_POINT('Ctrl Pts',(-3.38700359289755,-26.0622729395371,0.612099943781561));
#3247=CARTESIAN_POINT('Ctrl Pts',(-2.87059541238073,-25.0317435939839,0.72668327711495));
#3248=CARTESIAN_POINT('Ctrl Pts',(-2.48281014130459,-24.5799885832371,0.783974943781635));
#3249=CARTESIAN_POINT('Ctrl Pts',(-1.53584837306688,-23.9107391275463,0.898558277114875));
#3250=CARTESIAN_POINT('Ctrl Pts',(-0.977548004253359,-23.6939293925514,
0.955849943781558));
#3251=CARTESIAN_POINT('Ctrl Pts',(0.179952606081418,-23.5494218341822,1.07043327711495));
#3252=CARTESIAN_POINT('Ctrl Pts',(0.778050826506515,-23.6219155146099,1.1277249437816));
#3253=CARTESIAN_POINT('Ctrl Pts',(1.87337605723642,-24.0427561003574,1.24230827711491));
#3254=CARTESIAN_POINT('Ctrl Pts',(2.36953479367315,-24.3907498795612,1.29959994378166));
#3255=CARTESIAN_POINT('Ctrl Pts',(3.14152373336449,-25.2835693957278,1.41418327711485));
#3256=CARTESIAN_POINT('Ctrl Pts',(3.41657407444237,-25.8275750154296,1.47147494378145));
#3257=CARTESIAN_POINT('Ctrl Pts',(3.67788264996072,-26.9856580353439,1.58605827711506));
#3258=CARTESIAN_POINT('Ctrl Pts',(3.66383841906194,-27.5986380524938,1.64334994378159));
#3259=CARTESIAN_POINT('Ctrl Pts',(3.34637070640969,-28.7497648633494,1.75793327711492));
#3260=CARTESIAN_POINT('Ctrl Pts',(3.04319969463925,-29.2867949482463,1.81522494378156));
#3261=CARTESIAN_POINT('Ctrl Pts',(2.21569737033779,-30.1572282923719,1.92980827711495));
#3262=CARTESIAN_POINT('Ctrl Pts',(1.69211980095435,-30.4897610442556,1.98709994378157));
#3263=CARTESIAN_POINT('Ctrl Pts',(0.545399706903326,-30.8693375696566,2.10168327711494));
#3264=CARTESIAN_POINT('Ctrl Pts',(-0.0766613991650282,-30.9159670184662,
2.1589749437815));
#3265=CARTESIAN_POINT('Ctrl Pts',(-1.27368280615195,-30.7088161970159,2.27355827711501));
#3266=CARTESIAN_POINT('Ctrl Pts',(-1.84748758998441,-30.4551815910792,2.33084994378156));
#3267=CARTESIAN_POINT('Ctrl Pts',(-2.81085451659558,-29.7038376853842,2.44543327711495));
#3268=CARTESIAN_POINT('Ctrl Pts',(-3.19946114294195,-29.2068057482841,2.50272494378152));
#3269=CARTESIAN_POINT('Ctrl Pts',(-3.69753671927098,-28.0836711179268,2.61730827711499));
#3270=CARTESIAN_POINT('Ctrl Pts',(-3.806479757265,-27.4586223362847,2.67459994378158));
#3271=CARTESIAN_POINT('Ctrl Pts',(-3.71562427983475,-26.2264419408016,2.78918327711493));
#3272=CARTESIAN_POINT('Ctrl Pts',(-3.51585940949974,-25.6204942820667,2.84647494378164));
#3273=CARTESIAN_POINT('Ctrl Pts',(-2.85104937088523,-24.5708949233056,2.96105827711487));
#3274=CARTESIAN_POINT('Ctrl Pts',(-2.38659565795852,-24.1282770115141,3.01834994378155));
#3275=CARTESIAN_POINT('Ctrl Pts',(-1.29941716743804,-23.5127467708991,3.13293327711496));
#3276=CARTESIAN_POINT('Ctrl Pts',(-0.677707157851868,-23.3404704661548,
3.19022494378159));
#3277=CARTESIAN_POINT('Ctrl Pts',(0.578163753723292,-23.3101136508809,3.30480827711492));
#3278=CARTESIAN_POINT('Ctrl Pts',(1.21112328389688,-23.4521157051967,3.36209994378163));
#3279=CARTESIAN_POINT('Ctrl Pts',(2.33910331776924,-24.020612363763,3.47668327711488));
#3280=CARTESIAN_POINT('Ctrl Pts',(2.83301955876491,-24.4466103465917,3.53397494378134));
#3281=CARTESIAN_POINT('Ctrl Pts',(3.56365851013518,-25.4854479877254,3.64855827711517));
#3282=CARTESIAN_POINT('Ctrl Pts',(3.79963778298962,-26.0973236259647,3.70584994378171));
#3283=CARTESIAN_POINT('Ctrl Pts',(3.95497605633098,-27.3647903302184,3.8204332771148));
#3284=CARTESIAN_POINT('Ctrl Pts',(3.87413319178915,-28.0191741775874,3.87772494378131));
#3285=CARTESIAN_POINT('Ctrl Pts',(3.41100678604432,-29.2165864086031,3.9923082771152));
#3286=CARTESIAN_POINT('Ctrl Pts',(3.02911682295908,-29.7584488581732,4.04959994378164));
#3287=CARTESIAN_POINT('Ctrl Pts',(2.05088106415332,-30.6005370966614,4.16418327711487));
#3288=CARTESIAN_POINT('Ctrl Pts',(1.45543709786498,-30.8999159637434,4.2214749437816));
#3289=CARTESIAN_POINT('Ctrl Pts',(0.188979096554336,-31.1827816634333,4.33605827711491));
#3290=CARTESIAN_POINT('Ctrl Pts',(-0.480833880026034,-31.1659454082194,
4.39334994378137));
#3291=CARTESIAN_POINT('Ctrl Pts',(-1.73770084949707,-30.8164017691893,4.50793327711514));
#3292=CARTESIAN_POINT('Ctrl Pts',(-2.32353697868073,-30.4839775401827,4.5652249437816));
#3293=CARTESIAN_POINT('Ctrl Pts',(-3.2721043301499,-29.5783412086159,4.67980827711491));
#3294=CARTESIAN_POINT('Ctrl Pts',(-3.63389029917657,-29.0059575948908,4.73709994378148));
#3295=CARTESIAN_POINT('Ctrl Pts',(-4.04554275106343,-27.7534973422558,4.85168327711503));
#3296=CARTESIAN_POINT('Ctrl Pts',(-4.09496422407853,-27.0746032767544,4.90897494378134));
#3297=CARTESIAN_POINT('Ctrl Pts',(-3.86625627856773,-25.7692068883448,5.02355827711517));
#3298=CARTESIAN_POINT('Ctrl Pts',(-3.58829314652568,-25.1439637579671,5.08084994378156));
#3299=CARTESIAN_POINT('Ctrl Pts',(-2.76684994212521,-24.0951805886606,5.19543327711495));
#3300=CARTESIAN_POINT('Ctrl Pts',(-2.22411429181341,-23.6726777785058,5.25272494378155));
#3301=CARTESIAN_POINT('Ctrl Pts',(-0.998892661235347,-23.1323163820897,
5.36730827711496));
#3302=CARTESIAN_POINT('Ctrl Pts',(-0.317558252613747,-23.0150241600847,
5.42459994378155));
#3303=CARTESIAN_POINT('Ctrl Pts',(1.02458823678216,-23.1167103523708,5.53918327711497));
#3304=CARTESIAN_POINT('Ctrl Pts',(1.68411116492473,-23.3356447606771,5.59647494378161));
#3305=CARTESIAN_POINT('Ctrl Pts',(2.82558639662397,-24.061844294864,5.7110582771149));
#3306=CARTESIAN_POINT('Ctrl Pts',(3.30641702010581,-24.568459238132,5.76834994378167));
#3307=CARTESIAN_POINT('Ctrl Pts',(3.97403573885252,-25.7530884168939,5.88293327711484));
#3308=CARTESIAN_POINT('Ctrl Pts',(4.16013798020538,-26.4299946596524,5.94022494378164));
#3309=CARTESIAN_POINT('Ctrl Pts',(4.19049479552954,-27.7963637440239,6.05480827711487));
#3310=CARTESIAN_POINT('Ctrl Pts',(4.03466680450649,-28.4845195073438,6.11209994378139));
#3311=CARTESIAN_POINT('Ctrl Pts',(3.41408166790506,-29.7099502295094,6.22668327711512));
#3312=CARTESIAN_POINT('Ctrl Pts',(2.94987097329771,-30.2460277007815,6.28397494378131));
#3313=CARTESIAN_POINT('Ctrl Pts',(1.8191574593059,-31.0380561478021,6.3985582771152));
#3314=CARTESIAN_POINT('Ctrl Pts',(1.15370655160782,-31.2932049585382,6.45584994378166));
#3315=CARTESIAN_POINT('Ctrl Pts',(-0.22372624653663,-31.4593739468365,6.57043327711484));
#3316=CARTESIAN_POINT('Ctrl Pts',(-0.934395720889725,-31.3701818981879,
6.62772494378144));
#3317=CARTESIAN_POINT('Ctrl Pts',(-2.23389495213891,-30.8647696724464,6.74230827711507));
#3318=CARTESIAN_POINT('Ctrl Pts',(-2.82146111488582,-30.4489835254622,6.79959994378158));
#3319=CARTESIAN_POINT('Ctrl Pts',(-3.73364865213651,-29.3853315240515,6.91418327711493));
#3320=CARTESIAN_POINT('Ctrl Pts',(-4.05735604524484,-28.7384492111523,6.97147494378131));
#3321=CARTESIAN_POINT('Ctrl Pts',(-4.36177886909609,-27.3636162284599,7.0860582771152));
#3322=CARTESIAN_POINT('Ctrl Pts',(-4.34215058957306,-26.6369702924209,7.14334994378177));
#3323=CARTESIAN_POINT('Ctrl Pts',(-3.96053102416322,-25.2743631643761,7.25793327711474));
#3324=CARTESIAN_POINT('Ctrl Pts',(-3.59885357791486,-24.6397209908769,7.31522494378181));
#3325=CARTESIAN_POINT('Ctrl Pts',(-2.61508323909598,-23.61301963208,7.4298082771147));
#3326=CARTESIAN_POINT('Ctrl Pts',(-1.9938935810033,-23.2219804458925,7.48709994378137));
#3327=CARTESIAN_POINT('Ctrl Pts',(-0.635693169822906,-22.7782520675398,
7.60168327711514));
#3328=CARTESIAN_POINT('Ctrl Pts',(0.100033855150708,-22.726038570305,7.65897494378174));
#3329=CARTESIAN_POINT('Ctrl Pts',(1.51380522494329,-22.9763036398845,7.77355827711478));
#3330=CARTESIAN_POINT('Ctrl Pts',(2.19048670189786,-23.2785952980398,7.8308499437815));
#3331=CARTESIAN_POINT('Ctrl Pts',(3.32468611387601,-24.1701378011219,7.94543327711501));
#3332=CARTESIAN_POINT('Ctrl Pts',(3.78108510785602,-24.7585771646693,8.00272494378146));
#3333=CARTESIAN_POINT('Ctrl Pts',(4.36373232434941,-26.085885795444,8.11730827711505));
#3334=CARTESIAN_POINT('Ctrl Pts',(4.48937373037522,-26.8235058310766,8.17459994378218));
#3335=CARTESIAN_POINT('Ctrl Pts',(4.37685682322345,-28.2756184143465,8.28918327711433));
#3336=CARTESIAN_POINT('Ctrl Pts',(4.13875287694128,-28.9887166119371,8.3464749437818));
#3337=CARTESIAN_POINT('Ctrl Pts',(3.35116384720094,-30.2220677165326,8.46105827711471));
#3338=CARTESIAN_POINT('Ctrl Pts',(2.80238767357428,-30.741111051742,8.51834994378256));
#3339=CARTESIAN_POINT('Ctrl Pts',(1.52030780658665,-31.4608182485878,8.63293327711395));
#3340=CARTESIAN_POINT('Ctrl Pts',(0.788205330640013,-31.6607464265703,8.69022494378047));
#3341=CARTESIAN_POINT('Ctrl Pts',(-0.688661926511778,-31.6911032419353,
8.80480827711605));
#3342=CARTESIAN_POINT('Ctrl Pts',(-1.43201392300667,-31.5214493142069,8.86209994378189));
#3343=CARTESIAN_POINT('Ctrl Pts',(-2.75489533342443,-30.8487756995759,8.97668327711462));
#3344=CARTESIAN_POINT('Ctrl Pts',(-3.33313403500641,-30.3463522931823,9.03397494378135));
#3345=CARTESIAN_POINT('Ctrl Pts',(-4.18655197765132,-29.123762906342,9.14855827711516));
#3346=CARTESIAN_POINT('Ctrl Pts',(-4.46087032628663,-28.4047367291627,9.20584994378135));
#3347=CARTESIAN_POINT('Ctrl Pts',(-4.63787002953295,-26.9173378371627,9.32043327711516));
#3348=CARTESIAN_POINT('Ctrl Pts',(-4.54032879677263,-26.1503827357956,9.37772494378163));
#3349=CARTESIAN_POINT('Ctrl Pts',(-3.99263075105309,-24.7487965043376,9.49230827711489));
#3350=CARTESIAN_POINT('Ctrl Pts',(-3.54294842016277,-24.1155266283949,9.54959994378147));
#3351=CARTESIAN_POINT('Ctrl Pts',(-2.393880176143,-23.1332397923951,9.66418327711504));
#3352=CARTESIAN_POINT('Ctrl Pts',(-1.69555951661787,-22.7852038732428,9.72147494378146));
#3353=CARTESIAN_POINT('Ctrl Pts',(-0.21235155257781,-22.4592239252521,9.83605827711505));
#3354=CARTESIAN_POINT('Ctrl Pts',(0.571127342942618,-22.4816442290709,9.8933499437812));
#3355=CARTESIAN_POINT('Ctrl Pts',(2.03947462954967,-22.8953397208652,10.0079332771153));
#3356=CARTESIAN_POINT('Ctrl Pts',(2.72292284739241,-23.2862703843579,10.0652249437816));
#3357=CARTESIAN_POINT('Ctrl Pts',(3.82775821347252,-24.3481747304191,10.179808277115));
#3358=CARTESIAN_POINT('Ctrl Pts',(4.24805061685128,-25.0181704328983,10.237099943781));
#3359=CARTESIAN_POINT('Ctrl Pts',(4.72385492165356,-26.4821110025959,10.3516832771155));
#3360=CARTESIAN_POINT('Ctrl Pts',(4.77886044311237,-27.2746709870712,10.4089749437799));
#3361=CARTESIAN_POINT('Ctrl Pts',(4.50703824947158,-28.796817338216,10.5235582771166));
#3362=CARTESIAN_POINT('Ctrl Pts',(4.18041806520056,-29.5249371617849,10.580849943781));
#3363=CARTESIAN_POINT('Ctrl Pts',(3.21877626343458,-30.7445528163907,10.6954332771156));
#3364=CARTESIAN_POINT('Ctrl Pts',(2.58463318663832,-31.2348479942316,10.752724943781));
#3365=CARTESIAN_POINT('Ctrl Pts',(1.15523755569548,-31.8597810307748,10.8673082771155));
#3366=CARTESIAN_POINT('Ctrl Pts',(0.361331893025007,-31.9937716208391,10.9245999437816));
#3367=CARTESIAN_POINT('Ctrl Pts',(-1.20074678409337,-31.8704239988137,11.0391832771149));
#3368=CARTESIAN_POINT('Ctrl Pts',(-1.96742025115454,-31.6131505145616,11.0964749437817));
#3369=CARTESIAN_POINT('Ctrl Pts',(-3.29264722862687,-30.7641719892639,11.2110582771148));
#3370=CARTESIAN_POINT('Ctrl Pts',(-3.84990327557803,-30.1732345852601,11.2683499437819));
#3371=CARTESIAN_POINT('Ctrl Pts',(-4.62169895051392,-28.7937040300877,11.3829332771146));
#3372=CARTESIAN_POINT('Ctrl Pts',(-4.83545306471002,-28.0064053323945,11.4402249437801));
#3373=CARTESIAN_POINT('Ctrl Pts',(-4.85063147283344,-27.2127226059663,11.4975166104483));
#3374=CARTESIAN_POINT('',(-3.5,-27.2127225901214,0.49751661203513));
#3375=CARTESIAN_POINT('',(-3.5,-27.1131792176833,-0.497516612035131));
#3376=CARTESIAN_POINT('Origin',(-3.5,-27.1629509039024,-4.33680868994202E-16));
#3377=CARTESIAN_POINT('',(-4.85063029663924,-27.113179219224,10.5024833878107));
#3378=CARTESIAN_POINT('Ctrl Pts',(-3.5,-27.1131792176833,-0.497516612035131));
#3379=CARTESIAN_POINT('Ctrl Pts',(-3.49889065922935,-26.5404930476192,-0.440224945368445));
#3380=CARTESIAN_POINT('Ctrl Pts',(-3.3544424268553,-25.9668059432703,-0.382933278701826));
#3381=CARTESIAN_POINT('Ctrl Pts',(-3.08187392517324,-25.4592194500916,-0.325641612035131));
#3382=CARTESIAN_POINT('Ctrl Pts',(-2.80930542349117,-24.951632956913,-0.268349945368436));
#3383=CARTESIAN_POINT('Ctrl Pts',(-2.40909092606461,-24.5111434366068,-0.211058278701792));
#3384=CARTESIAN_POINT('Ctrl Pts',(-1.92656123086921,-24.1900615952905,-0.153766612035131));
#3385=CARTESIAN_POINT('Ctrl Pts',(-1.4440315356738,-23.8689797539743,-0.0964749453684703));
#3386=CARTESIAN_POINT('Ctrl Pts',(-0.880080083275106,-23.6679643912945,
-0.0391832787017876));
#3387=CARTESIAN_POINT('Ctrl Pts',(-0.299733511718495,-23.6119199517362,
0.018108387964869));
#3388=CARTESIAN_POINT('Ctrl Pts',(0.280613059838117,-23.5558755121778,0.0754000546315256));
#3389=CARTESIAN_POINT('Ctrl Pts',(0.876249675472422,-23.6449624877681,0.132691721298213));
#3390=CARTESIAN_POINT('Ctrl Pts',(1.41767904230447,-23.8704306167052,0.189983387964869));
#3391=CARTESIAN_POINT('Ctrl Pts',(1.95910840913652,-24.0958987456423,0.247275054631525));
#3392=CARTESIAN_POINT('Ctrl Pts',(2.44527417877255,-24.4573661122303,0.304566721298234));
#3393=CARTESIAN_POINT('Ctrl Pts',(2.81867791337221,-24.9141085439026,0.361858387964869));
#3394=CARTESIAN_POINT('Ctrl Pts',(3.19208164797187,-25.370850975575,0.419150054631504));
#3395=CARTESIAN_POINT('Ctrl Pts',(3.45196757401249,-25.9220285865551,0.476441721298107));
#3396=CARTESIAN_POINT('Ctrl Pts',(3.56664703600973,-26.50424746956,0.533733387964869));
#3397=CARTESIAN_POINT('Ctrl Pts',(3.68132649800696,-27.086466352565,0.591025054631631));
#3398=CARTESIAN_POINT('Ctrl Pts',(3.65052759374337,-27.6986230455641,0.648316721298202));
#3399=CARTESIAN_POINT('Ctrl Pts',(3.47620739559618,-28.2694581631131,0.705608387964869));
#3400=CARTESIAN_POINT('Ctrl Pts',(3.30188719744899,-28.840293280662,0.762900054631535));
#3401=CARTESIAN_POINT('Ctrl Pts',(2.98432799528007,-29.3686991601337,0.820191721298179));
#3402=CARTESIAN_POINT('Ctrl Pts',(2.5590598063206,-29.7923985038961,0.877483387964869));
#3403=CARTESIAN_POINT('Ctrl Pts',(2.13379161736112,-30.2160978476585,0.93477505463156));
#3404=CARTESIAN_POINT('Ctrl Pts',(1.60159021920541,-30.5342421833904,0.992066721298096));
#3405=CARTESIAN_POINT('Ctrl Pts',(1.0235022923127,-30.7084439804978,1.04935838796487));
#3406=CARTESIAN_POINT('Ctrl Pts',(0.445414365419992,-30.8826457776052,1.10665005463164));
#3407=CARTESIAN_POINT('Ctrl Pts',(-0.177469626200368,-30.9125205315103,
1.16394172129828));
#3408=CARTESIAN_POINT('Ctrl Pts',(-0.772802538464799,-30.7929703781997,
1.22123338796487));
#3409=CARTESIAN_POINT('Ctrl Pts',(-1.36813545072923,-30.673420224889,1.27852505463146));
#3410=CARTESIAN_POINT('Ctrl Pts',(-1.93476784632414,-30.4046213916764,1.33581672129817));
#3411=CARTESIAN_POINT('Ctrl Pts',(-2.40611830644423,-30.0163589740654,1.39310838796487));
#3412=CARTESIAN_POINT('Ctrl Pts',(-2.87746876656431,-29.6280965564544,1.45040005463156));
#3413=CARTESIAN_POINT('Ctrl Pts',(-3.25260154395457,-29.1210720052738,1.50769172129813));
#3414=CARTESIAN_POINT('Ctrl Pts',(-3.48659133287997,-28.5532718354748,1.56498338796487));
#3415=CARTESIAN_POINT('Ctrl Pts',(-3.72058112180538,-27.9854716656758,1.62227505463161));
#3416=CARTESIAN_POINT('Ctrl Pts',(-3.81293080022416,-27.3579617136213,1.67956672129819));
#3417=CARTESIAN_POINT('Ctrl Pts',(-3.75129376366397,-26.743468206589,1.73685838796487));
#3418=CARTESIAN_POINT('Ctrl Pts',(-3.68965672710377,-26.1289746995567,1.79415005463154));
#3419=CARTESIAN_POINT('Ctrl Pts',(-3.47409763241299,-25.5286785378583,1.85144172129826));
#3420=CARTESIAN_POINT('Ctrl Pts',(-3.12814996344534,-25.0129280240762,1.90873338796487));
#3421=CARTESIAN_POINT('Ctrl Pts',(-2.7822022944777,-24.4971775102941,1.96602505463148));
#3422=CARTESIAN_POINT('Ctrl Pts',(-2.30648341649854,-24.0669891197329,2.02331672129817));
#3423=CARTESIAN_POINT('Ctrl Pts',(-1.75521636766239,-23.7735886118537,2.08060838796487));
#3424=CARTESIAN_POINT('Ctrl Pts',(-1.20394931882625,-23.4801881039745,2.13790005463157));
#3425=CARTESIAN_POINT('Ctrl Pts',(-0.578163556381755,-23.3241840203502,
2.19519172129821));
#3426=CARTESIAN_POINT('Ctrl Pts',(0.0497716862190717,-23.3252933614194,
2.25248338796487));
#3427=CARTESIAN_POINT('Ctrl Pts',(0.677706928819894,-23.3264027024885,2.30977505463153));
#3428=CARTESIAN_POINT('Ctrl Pts',(1.30659028017156,-23.4846768712254,2.36706672129824));
#3429=CARTESIAN_POINT('Ctrl Pts',(1.86290211750193,-23.7832896119458,2.42435838796487));
#3430=CARTESIAN_POINT('Ctrl Pts',(2.4192139548323,-24.0819023526662,2.4816500546315));
#3431=CARTESIAN_POINT('Ctrl Pts',(2.90186470540991,-24.520329561822,2.53894172129796));
#3432=CARTESIAN_POINT('Ctrl Pts',(3.2536412945512,-25.0487971934751,2.59623338796487));
#3433=CARTESIAN_POINT('Ctrl Pts',(3.6054178836925,-25.5772648251282,2.65352505463178));
#3434=CARTESIAN_POINT('Ctrl Pts',(3.82560278426284,-26.1947915469425,2.71081672129833));
#3435=CARTESIAN_POINT('Ctrl Pts',(3.88706258129088,-26.830121165459,2.76810838796487));
#3436=CARTESIAN_POINT('Ctrl Pts',(3.94852237831892,-27.4654507839756,2.82540005463141));
#3437=CARTESIAN_POINT('Ctrl Pts',(3.85108621864684,-28.1173730265607,2.88269172129792));
#3438=CARTESIAN_POINT('Ctrl Pts',(3.60447517969519,-28.7098458935282,2.93998338796487));
#3439=CARTESIAN_POINT('Ctrl Pts',(3.35786414074354,-29.3023187604958,2.99727505463182));
#3440=CARTESIAN_POINT('Ctrl Pts',(2.96250059030192,-29.8341882432863,3.05456672129825));
#3441=CARTESIAN_POINT('Ctrl Pts',(2.46305003729807,-30.2426416272707,3.11185838796487));
#3442=CARTESIAN_POINT('Ctrl Pts',(1.96359948429421,-30.6510950112551,3.16915005463149));
#3443=CARTESIAN_POINT('Ctrl Pts',(1.36098352674217,-30.93530946333,3.22644172129821));
#3444=CARTESIAN_POINT('Ctrl Pts',(0.7245771530364,-31.0607674873965,3.28373338796487));
#3445=CARTESIAN_POINT('Ctrl Pts',(0.0881707793306251,-31.186225511463,3.34102505463152));
#3446=CARTESIAN_POINT('Ctrl Pts',(-0.580818873102877,-31.1526345829163,
3.39831672129799));
#3447=CARTESIAN_POINT('Ctrl Pts',(-1.20452406995301,-30.9622764215647,3.45560838796487));
#3448=CARTESIAN_POINT('Ctrl Pts',(-1.82822926680315,-30.7719182602131,3.51290005463175));
#3449=CARTESIAN_POINT('Ctrl Pts',(-2.40544119057821,-30.4251058408366,3.57019172129822));
#3450=CARTESIAN_POINT('Ctrl Pts',(-2.86820753800229,-29.9607706482314,3.62748338796487));
#3451=CARTESIAN_POINT('Ctrl Pts',(-3.33097388542638,-29.4964354556262,3.68477505463152));
#3452=CARTESIAN_POINT('Ctrl Pts',(-3.67837143832636,-28.9154280131467,3.74206672129809));
#3453=CARTESIAN_POINT('Ctrl Pts',(-3.86861119866167,-28.2844700069572,3.79935838796487));
#3454=CARTESIAN_POINT('Ctrl Pts',(-4.05885095899697,-27.6535120007677,3.85665005463165));
#3455=CARTESIAN_POINT('Ctrl Pts',(-4.09151773713705,-26.9737950497155,3.91394172129795));
#3456=CARTESIAN_POINT('Ctrl Pts',(-3.96118902178175,-26.3242746467433,3.97123338796487));
#3457=CARTESIAN_POINT('Ctrl Pts',(-3.83086030642645,-25.6747542437711,4.02852505463179));
#3458=CARTESIAN_POINT('Ctrl Pts',(-3.53773294713309,-25.0566835016172,4.08581672129817));
#3459=CARTESIAN_POINT('Ctrl Pts',(-3.11442088015912,-24.5426249201597,4.14310838796487));
#3460=CARTESIAN_POINT('Ctrl Pts',(-2.69110881318516,-24.0285663387021,4.20040005463157));
#3461=CARTESIAN_POINT('Ctrl Pts',(-2.13838054880758,-23.6195373774773,4.25769172129816));
#3462=CARTESIAN_POINT('Ctrl Pts',(-1.51953687889374,-23.3644046785242,4.31498338796487));
#3463=CARTESIAN_POINT('Ctrl Pts',(-0.900693208979914,-23.1092719795712,
4.37227505463158));
#3464=CARTESIAN_POINT('Ctrl Pts',(-0.216897629946521,-23.0085731171096,
4.42956672129816));
#3465=CARTESIAN_POINT('Ctrl Pts',(0.452578924038324,-23.0756255111136,4.48685838796487));
#3466=CARTESIAN_POINT('Ctrl Pts',(1.12205547802317,-23.1426779051177,4.54415005463158));
#3467=CARTESIAN_POINT('Ctrl Pts',(1.77592690914455,-23.377406537751,4.60144172129822));
#3468=CARTESIAN_POINT('Ctrl Pts',(2.33761535938431,-23.7540489545177,4.65873338796487));
#3469=CARTESIAN_POINT('Ctrl Pts',(2.89930380962407,-24.1306913712844,4.71602505463151));
#3470=CARTESIAN_POINT('Ctrl Pts',(3.36770491189876,-24.6485714795865,4.77331672129828));
#3471=CARTESIAN_POINT('Ctrl Pts',(3.68714965883202,-25.2485638725488,4.83060838796487));
#3472=CARTESIAN_POINT('Ctrl Pts',(4.00659440576528,-25.8485562655112,4.88790005463146));
#3473=CARTESIAN_POINT('Ctrl Pts',(4.17642442602432,-26.5295382611225,4.94519172129826));
#3474=CARTESIAN_POINT('Ctrl Pts',(4.17531508496597,-27.2127225901215,5.00248338796487));
#3475=CARTESIAN_POINT('Ctrl Pts',(4.17420574390762,-27.8959069191205,5.05977505463148));
#3476=CARTESIAN_POINT('Ctrl Pts',(4.00210563848955,-28.579986503623,5.117066721298));
#3477=CARTESIAN_POINT('Ctrl Pts',(3.67744865873987,-29.1850236850955,5.17435838796487));
#3478=CARTESIAN_POINT('Ctrl Pts',(3.35279167899019,-29.790060866568,5.23165005463174));
#3479=CARTESIAN_POINT('Ctrl Pts',(2.8761517580747,-30.3148728474363,5.28894172129792));
#3480=CARTESIAN_POINT('Ctrl Pts',(2.30174618998527,-30.697344184393,5.34623338796487));
#3481=CARTESIAN_POINT('Ctrl Pts',(1.72734062189585,-31.0798155213495,5.40352505463181));
#3482=CARTESIAN_POINT('Ctrl Pts',(1.05623863063331,-31.319169959825,5.46081672129828));
#3483=CARTESIAN_POINT('Ctrl Pts',(0.365925965168119,-31.386045114318,5.51810838796487));
#3484=CARTESIAN_POINT('Ctrl Pts',(-0.324386700297069,-31.4529202688109,
5.57540005463146));
#3485=CARTESIAN_POINT('Ctrl Pts',(-1.03259456986735,-31.3471349250583,5.63269172129805));
#3486=CARTESIAN_POINT('Ctrl Pts',(-1.67611093694732,-31.0793809760956,5.68998338796487));
#3487=CARTESIAN_POINT('Ctrl Pts',(-2.3196273040273,-30.8116270271329,5.74727505463168));
#3488=CARTESIAN_POINT('Ctrl Pts',(-2.89720050000837,-30.3823672928139,5.80456672129819));
#3489=CARTESIAN_POINT('Ctrl Pts',(-3.34070353336454,-29.8402086184987,5.86185838796487));
#3490=CARTESIAN_POINT('Ctrl Pts',(-3.78420656672072,-29.2980499441836,5.91915005463154));
#3491=CARTESIAN_POINT('Ctrl Pts',(-4.09274954484339,-28.643995640032,5.97644172129792));
#3492=CARTESIAN_POINT('Ctrl Pts',(-4.22898613097863,-27.9534017756328,6.03373338796487));
#3493=CARTESIAN_POINT('Ctrl Pts',(-4.36522271711388,-27.2628079112337,6.09102505463182));
#3494=CARTESIAN_POINT('Ctrl Pts',(-4.32883976428306,-26.5369852993421,6.14831672129839));
#3495=CARTESIAN_POINT('Ctrl Pts',(-4.1224436397285,-25.860410023207,6.20560838796487));
#3496=CARTESIAN_POINT('Ctrl Pts',(-3.91604751517394,-25.183834747072,6.26290005463135));
#3497=CARTESIAN_POINT('Ctrl Pts',(-3.53998187857711,-24.5578167789666,6.32019172129842));
#3498=CARTESIAN_POINT('Ctrl Pts',(-3.03657968233749,-24.0559834278915,6.37748338796487));
#3499=CARTESIAN_POINT('Ctrl Pts',(-2.53317748609787,-23.5541500768163,6.43477505463132));
#3500=CARTESIAN_POINT('Ctrl Pts',(-1.90336399926295,-23.1774993067315,6.49206672129798));
#3501=CARTESIAN_POINT('Ctrl Pts',(-1.21953591379696,-22.9712215831745,6.54935838796487));
#3502=CARTESIAN_POINT('Ctrl Pts',(-0.535707828330976,-22.7649438596174,
6.60665005463175));
#3503=CARTESIAN_POINT('Ctrl Pts',(0.200842082192416,-22.7294850572333,6.66394172129835));
#3504=CARTESIAN_POINT('Ctrl Pts',(0.904549975853311,-22.8705923346362,6.72123338796487));
#3505=CARTESIAN_POINT('Ctrl Pts',(1.60825786951421,-23.011699612039,6.77852505463139));
#3506=CARTESIAN_POINT('Ctrl Pts',(2.27776695825421,-23.3291554974211,6.8358167212985));
#3507=CARTESIAN_POINT('Ctrl Pts',(2.83453366104116,-23.7875172137472,6.89310838796487));
#3508=CARTESIAN_POINT('Ctrl Pts',(3.39130036382812,-24.2458789300732,6.95040005463124));
#3509=CARTESIAN_POINT('Ctrl Pts',(3.83422550889456,-24.8443109076698,7.00769172129807));
#3510=CARTESIAN_POINT('Ctrl Pts',(4.11050111787622,-25.5141980776873,7.06498338796487));
#3511=CARTESIAN_POINT('Ctrl Pts',(4.38677672685788,-26.1840852477049,7.12227505463167));
#3512=CARTESIAN_POINT('Ctrl Pts',(4.49582477336048,-26.9241664537426,7.17956672129841));
#3513=CARTESIAN_POINT('Ctrl Pts',(4.42335702191342,-27.6486260546656,7.23685838796487));
#3514=CARTESIAN_POINT('Ctrl Pts',(4.35088927046636,-28.3730856555887,7.29415005463133));
#3515=CARTESIAN_POINT('Ctrl Pts',(4.09699109987682,-29.0805323561617,7.35144172129841));
#3516=CARTESIAN_POINT('Ctrl Pts',(3.68965393532396,-29.6881587428448,7.40873338796487));
#3517=CARTESIAN_POINT('Ctrl Pts',(3.2823167707711,-30.295785129528,7.46602505463132));
#3518=CARTESIAN_POINT('Ctrl Pts',(2.72227543212691,-30.8023989435457,7.52331672129839));
#3519=CARTESIAN_POINT('Ctrl Pts',(2.07355769504457,-31.1478879295178,7.58060838796487));
#3520=CARTESIAN_POINT('Ctrl Pts',(1.42483995796224,-31.4933769154898,7.63790005463135));
#3521=CARTESIAN_POINT('Ctrl Pts',(0.688661729169903,-31.6770328723976,7.69519172129708));
#3522=CARTESIAN_POINT('Ctrl Pts',(-0.0497716862192416,-31.6759235313513,
7.75248338796487));
#3523=CARTESIAN_POINT('Ctrl Pts',(-0.788205101608386,-31.674814190305,7.80977505463266));
#3524=CARTESIAN_POINT('Ctrl Pts',(-1.52748091929412,-31.4888881482022,7.8670667212985));
#3525=CARTESIAN_POINT('Ctrl Pts',(-2.18124344488441,-31.1381869294255,7.92435838796487));
#3526=CARTESIAN_POINT('Ctrl Pts',(-2.83500597047471,-30.7874857106489,7.98165005463124));
#3527=CARTESIAN_POINT('Ctrl Pts',(-3.40197918167131,-30.2726330779668,8.03894172129796));
#3528=CARTESIAN_POINT('Ctrl Pts',(-3.81514526643002,-29.6522895734456,8.09623338796487));
#3529=CARTESIAN_POINT('Ctrl Pts',(-4.22831135118872,-29.0319460689245,8.15352505463178));
#3530=CARTESIAN_POINT('Ctrl Pts',(-4.48683532758525,-28.3072688081897,8.21081672129796));
#3531=CARTESIAN_POINT('Ctrl Pts',(-4.55912583954038,-27.5619730957952,8.26810838796487));
#3532=CARTESIAN_POINT('Ctrl Pts',(-4.63141635149551,-26.8166773834008,8.32540005463178));
#3533=CARTESIAN_POINT('Ctrl Pts',(-4.51728182365348,-26.0521838868124,8.38269172129824));
#3534=CARTESIAN_POINT('Ctrl Pts',(-4.22838496469132,-25.3576240196336,8.43998338796487));
#3535=CARTESIAN_POINT('Ctrl Pts',(-3.93948810572916,-24.6630641524548,8.4972750546315));
#3536=CARTESIAN_POINT('Ctrl Pts',(-3.47633218752116,-24.0397872432635,8.55456672129809));
#3537=CARTESIAN_POINT('Ctrl Pts',(-2.89146539189475,-23.5612345605416,8.61185838796487));
#3538=CARTESIAN_POINT('Ctrl Pts',(-2.30659859626834,-23.0826818778197,8.66915005463165));
#3539=CARTESIAN_POINT('Ctrl Pts',(-1.60110594549964,-22.7498103736324,8.72644172129807));
#3540=CARTESIAN_POINT('Ctrl Pts',(-0.856324590424587,-22.6027952254392,
8.78373338796487));
#3541=CARTESIAN_POINT('Ctrl Pts',(-0.111543235349539,-22.455780077246,8.84102505463166));
#3542=CARTESIAN_POINT('Ctrl Pts',(0.671112336026928,-22.4949550543515,8.89831672129782));
#3543=CARTESIAN_POINT('Ctrl Pts',(1.4005576914376,-22.7173891421077,8.95560838796487));
#3544=CARTESIAN_POINT('Ctrl Pts',(2.13000304684828,-22.9398232298639,9.01290005463192));
#3545=CARTESIAN_POINT('Ctrl Pts',(2.80482705930729,-23.3451420836895,9.07019172129816));
#3546=CARTESIAN_POINT('Ctrl Pts',(3.34572741401944,-23.8876112835564,9.12748338796487));
#3547=CARTESIAN_POINT('Ctrl Pts',(3.88662776873157,-24.4300804834233,9.18477505463157));
#3548=CARTESIAN_POINT('Ctrl Pts',(4.292531756023,-25.1087000146355,9.24206672129765));
#3549=CARTESIAN_POINT('Ctrl Pts',(4.51484744279408,-25.8453981793633,9.29935838796487));
#3550=CARTESIAN_POINT('Ctrl Pts',(4.73716312956515,-26.582096344091,9.35665005463209));
#3551=CARTESIAN_POINT('Ctrl Pts',(4.77541395619357,-27.3754792141155,9.4139417212973));
#3552=CARTESIAN_POINT('Ctrl Pts',(4.6235281167506,-28.1333745984499,9.47123338796487));
#3553=CARTESIAN_POINT('Ctrl Pts',(4.47164227730762,-28.8912699827844,9.52852505463244));
#3554=CARTESIAN_POINT('Ctrl Pts',(4.12985786582675,-29.6122174181468,9.58581672129756));
#3555=CARTESIAN_POINT('Ctrl Pts',(3.63644650015124,-30.211692242242,9.64310838796487));
#3556=CARTESIAN_POINT('Ctrl Pts',(3.14303513447573,-30.8111670663372,9.70040005463217));
#3557=CARTESIAN_POINT('Ctrl Pts',(2.49889944364267,-31.2879883952817,9.7576917212976));
#3558=CARTESIAN_POINT('Ctrl Pts',(1.77796877353627,-31.5854069142767,9.81498338796487));
#3559=CARTESIAN_POINT('Ctrl Pts',(1.05703810342986,-31.8828254332717,9.87227505463214));
#3560=CARTESIAN_POINT('Ctrl Pts',(0.260671270356954,-32.0002226638335,9.92956672129819));
#3561=CARTESIAN_POINT('Ctrl Pts',(-0.518771377488306,-31.9223395549405,
9.98685838796487));
#3562=CARTESIAN_POINT('Ctrl Pts',(-1.29821402533357,-31.8444564460475,10.0441500546315));
#3563=CARTESIAN_POINT('Ctrl Pts',(-2.05923599538643,-31.5713887375034,10.1014417212983));
#3564=CARTESIAN_POINT('Ctrl Pts',(-2.71280031850067,-31.1333568251656,10.1587333879649));
#3565=CARTESIAN_POINT('Ctrl Pts',(-3.36636464161491,-30.6953249128279,10.2160250546314));
#3566=CARTESIAN_POINT('Ctrl Pts',(-3.91119116738902,-30.0931223438177,10.2733167212985));
#3567=CARTESIAN_POINT('Ctrl Pts',(-4.28272439239882,-29.395679262638,10.3306083879649));
#3568=CARTESIAN_POINT('Ctrl Pts',(-4.65425761740862,-28.6982361814583,10.3879000546312));
#3569=CARTESIAN_POINT('Ctrl Pts',(-4.85173820194801,-27.9068617491303,10.445191722014));
#3570=CARTESIAN_POINT('Ctrl Pts',(-4.85063030442627,-27.1131792193187,10.5024833878013));
#3571=CARTESIAN_POINT('Origin',(-4.85063016993195,-27.162950903902,11.));
#3572=CARTESIAN_POINT('Ctrl Pts',(-3.5,-27.2127225901214,0.49751661203513));
#3573=CARTESIAN_POINT('Ctrl Pts',(-3.51517840571961,-26.6400364200585,0.554808278701816));
#3574=CARTESIAN_POINT('Ctrl Pts',(-3.3870023381626,-26.0622733505101,0.612099945368435));
#3575=CARTESIAN_POINT('Ctrl Pts',(-3.12879834611319,-25.5470088669697,0.66939161203513));
#3576=CARTESIAN_POINT('Ctrl Pts',(-2.87059435406378,-25.0317443834292,0.726683278701825));
#3577=CARTESIAN_POINT('Ctrl Pts',(-2.48280922845853,-24.5799895371609,0.78397494536851));
#3578=CARTESIAN_POINT('Ctrl Pts',(-2.00932852015756,-24.2453649299115,0.84126661203513));
#3579=CARTESIAN_POINT('Ctrl Pts',(-1.5358478118566,-23.9107403226621,0.89855827870175));
#3580=CARTESIAN_POINT('Ctrl Pts',(-0.9775476488716,-23.6939306641498,0.955849945368433));
#3581=CARTESIAN_POINT('Ctrl Pts',(-0.398797555610286,-23.6216769084413,
1.01314161203513));
#3582=CARTESIAN_POINT('Ctrl Pts',(0.179952537651027,-23.5494231527329,1.07043327870183));
#3583=CARTESIAN_POINT('Ctrl Pts',(0.778050540497908,-23.6219168035854,1.12772494536847));
#3584=CARTESIAN_POINT('Ctrl Pts',(1.3257129579118,-23.8323370172714,1.18501661203513));
#3585=CARTESIAN_POINT('Ctrl Pts',(1.8733753753257,-24.0427572309574,1.24230827870179));
#3586=CARTESIAN_POINT('Ctrl Pts',(2.36953393381726,-24.3907508815125,1.29959994536854));
#3587=CARTESIAN_POINT('Ctrl Pts',(2.75552826641451,-24.837160476445,1.35689161203513));
#3588=CARTESIAN_POINT('Ctrl Pts',(3.14152259901176,-25.2835700713775,1.41418327870172));
#3589=CARTESIAN_POINT('Ctrl Pts',(3.41657284380058,-25.8275754937386,1.47147494536833));
#3590=CARTESIAN_POINT('Ctrl Pts',(3.54722708742622,-26.4066167951111,1.52876661203513));
#3591=CARTESIAN_POINT('Ctrl Pts',(3.67788133105185,-26.9856580964837,1.58605827870193));
#3592=CARTESIAN_POINT('Ctrl Pts',(3.6638371082595,-27.5986378942041,1.64334994536846));
#3593=CARTESIAN_POINT('Ctrl Pts',(3.50510331133718,-28.1742010948723,1.70064161203513));
#3594=CARTESIAN_POINT('Ctrl Pts',(3.34636951441486,-28.7497642955405,1.7579332787018));
#3595=CARTESIAN_POINT('Ctrl Pts',(3.04319861323196,-29.2867941907393,1.81522494536844));
#3596=CARTESIAN_POINT('Ctrl Pts',(2.62944759999372,-29.7220107102229,1.87251661203513));
#3597=CARTESIAN_POINT('Ctrl Pts',(2.21569658675549,-30.1572272297066,1.92980827870182));
#3598=CARTESIAN_POINT('Ctrl Pts',(1.69211920432461,-30.4897598664222,1.98709994536844));
#3599=CARTESIAN_POINT('Ctrl Pts',(1.11875936055348,-30.6795480647568,2.04439161203513));
#3600=CARTESIAN_POINT('Ctrl Pts',(0.545399516782366,-30.8693362630914,2.10168327870182));
#3601=CARTESIAN_POINT('Ctrl Pts',(-0.0766613701186385,-30.9159656984605,
2.15897494536837));
#3602=CARTESIAN_POINT('Ctrl Pts',(-0.67517186401586,-30.8123903267832,2.21626661203513));
#3603=CARTESIAN_POINT('Ctrl Pts',(-1.27368235791308,-30.7088149551059,2.27355827870189));
#3604=CARTESIAN_POINT('Ctrl Pts',(-1.84748694212142,-30.4551804406305,2.33084994536844));
#3605=CARTESIAN_POINT('Ctrl Pts',(-2.32917023898663,-30.0795086210231,2.38814161203513));
#3606=CARTESIAN_POINT('Ctrl Pts',(-2.81085353585185,-29.7038368014157,2.44543327870183));
#3607=CARTESIAN_POINT('Ctrl Pts',(-3.19946002926004,-29.2068050390794,2.50272494536839));
#3608=CARTESIAN_POINT('Ctrl Pts',(-3.44849773344619,-28.6452379198675,2.56001661203513));
#3609=CARTESIAN_POINT('Ctrl Pts',(-3.69753543763233,-28.0836708006555,2.61730827870187));
#3610=CARTESIAN_POINT('Ctrl Pts',(-3.80647844076847,-27.458622235808,2.67459994536845));
#3611=CARTESIAN_POINT('Ctrl Pts',(-3.76105072036911,-26.8425322504808,2.73189161203513));
#3612=CARTESIAN_POINT('Ctrl Pts',(-3.71562299996974,-26.2264422651536,2.7891832787018));
#3613=CARTESIAN_POINT('Ctrl Pts',(-3.51585820108909,-25.6204948140464,2.84647494536852));
#3614=CARTESIAN_POINT('Ctrl Pts',(-3.18345329806631,-25.0956953133645,2.90376661203513));
#3615=CARTESIAN_POINT('Ctrl Pts',(-2.85104839504354,-24.5708958126827,2.96105827870174));
#3616=CARTESIAN_POINT('Ctrl Pts',(-2.38659484300895,-24.1282780503191,3.01834994536843));
#3617=CARTESIAN_POINT('Ctrl Pts',(-1.84300578454046,-23.8205130327937,3.07564161203513));
#3618=CARTESIAN_POINT('Ctrl Pts',(-1.29941672607197,-23.5127480152682,3.13293327870183));
#3619=CARTESIAN_POINT('Ctrl Pts',(-0.677706928819807,-23.3404717664636,
3.19022494536847));
#3620=CARTESIAN_POINT('Ctrl Pts',(-0.0497716862189807,-23.3252933614193,
3.24751661203513));
#3621=CARTESIAN_POINT('Ctrl Pts',(0.578163556381841,-23.3101149563751,3.30480827870179));
#3622=CARTESIAN_POINT('Ctrl Pts',(1.21112287292379,-23.4521169599317,3.3620999453685));
#3623=CARTESIAN_POINT('Ctrl Pts',(1.77511270062386,-23.7363651910058,3.41939161203513));
#3624=CARTESIAN_POINT('Ctrl Pts',(2.33910252832392,-24.02061342208,3.47668327870176));
#3625=CARTESIAN_POINT('Ctrl Pts',(2.83301860484105,-24.4466112594378,3.53397494536822));
#3626=CARTESIAN_POINT('Ctrl Pts',(3.19833795993023,-24.9660299041867,3.59126661203513));
#3627=CARTESIAN_POINT('Ctrl Pts',(3.56365731501942,-25.4854485489357,3.64855827870204));
#3628=CARTESIAN_POINT('Ctrl Pts',(3.79963651139122,-26.0973239813465,3.70584994536859));
#3629=CARTESIAN_POINT('Ctrl Pts',(3.87730562458575,-26.7310571215672,3.76314161203513));
#3630=CARTESIAN_POINT('Ctrl Pts',(3.95497473778028,-27.364790261788,3.82043327870167));
#3631=CARTESIAN_POINT('Ctrl Pts',(3.87413190281369,-28.0191738915788,3.87772494536818));
#3632=CARTESIAN_POINT('Ctrl Pts',(3.64256877912899,-28.6178798091356,3.93501661203513));
#3633=CARTESIAN_POINT('Ctrl Pts',(3.41100565544429,-29.2165857266924,3.99230827870208));
#3634=CARTESIAN_POINT('Ctrl Pts',(3.02911582100773,-29.7584479983173,4.04959994536851));
#3635=CARTESIAN_POINT('Ctrl Pts',(2.53999810475567,-30.179491980313,4.10689161203513));
#3636=CARTESIAN_POINT('Ctrl Pts',(2.05088038850359,-30.6005359623087,4.16418327870175));
#3637=CARTESIAN_POINT('Ctrl Pts',(1.45543661955603,-30.8999147331016,4.22147494536847));
#3638=CARTESIAN_POINT('Ctrl Pts',(0.822207827485342,-31.041347538813,4.27876661203513));
#3639=CARTESIAN_POINT('Ctrl Pts',(0.188979035414649,-31.1827803445244,4.33605827870178));
#3640=CARTESIAN_POINT('Ctrl Pts',(-0.480833721736333,-31.1659440974169,
4.39334994536825));
#3641=CARTESIAN_POINT('Ctrl Pts',(-1.10926700171223,-30.9911723373057,4.45064161203513));
#3642=CARTESIAN_POINT('Ctrl Pts',(-1.73770028168812,-30.8164005771944,4.50793327870201));
#3643=CARTESIAN_POINT('Ctrl Pts',(-2.32353622117369,-30.4839764587754,4.56522494536848));
#3644=CARTESIAN_POINT('Ctrl Pts',(-2.79781974432916,-30.0311584419045,4.62251661203513));
#3645=CARTESIAN_POINT('Ctrl Pts',(-3.27210326748465,-29.5783404250336,4.67980827870178));
#3646=CARTESIAN_POINT('Ctrl Pts',(-3.63388912134312,-29.0059569982611,4.73709994536835));
#3647=CARTESIAN_POINT('Ctrl Pts',(-3.83971528292067,-28.379727075198,4.79439161203513));
#3648=CARTESIAN_POINT('Ctrl Pts',(-4.04554144449821,-27.7534971521348,4.85168327870191));
#3649=CARTESIAN_POINT('Ctrl Pts',(-4.09496290407286,-27.0746033058008,4.90897494536821));
#3650=CARTESIAN_POINT('Ctrl Pts',(-3.98060897036527,-26.4219053211922,4.96626661203513));
#3651=CARTESIAN_POINT('Ctrl Pts',(-3.86625503665767,-25.7692073365837,5.02355827870204));
#3652=CARTESIAN_POINT('Ctrl Pts',(-3.58829199607698,-25.1439644058301,5.08084994536843));
#3653=CARTESIAN_POINT('Ctrl Pts',(-3.17757052711683,-24.6195729876172,5.13814161203513));
#3654=CARTESIAN_POINT('Ctrl Pts',(-2.76684905815666,-24.0951815694043,5.19543327870183));
#3655=CARTESIAN_POINT('Ctrl Pts',(-2.22411358260874,-23.6726788921877,5.25272494536842));
#3656=CARTESIAN_POINT('Ctrl Pts',(-1.61150296328641,-23.402498277958,5.31001661203513));
#3657=CARTESIAN_POINT('Ctrl Pts',(-0.998892343964086,-23.1323176637283,
5.36730827870184));
#3658=CARTESIAN_POINT('Ctrl Pts',(-0.317558152137085,-23.0150254765812,
5.42459994536842));
#3659=CARTESIAN_POINT('Ctrl Pts',(0.353514880146535,-23.0658685544085,5.48189161203513));
#3660=CARTESIAN_POINT('Ctrl Pts',(1.02458791243016,-23.1167116322358,5.53918327870184));
#3661=CARTESIAN_POINT('Ctrl Pts',(1.68411063294507,-23.3356459690878,5.59647494536849));
#3662=CARTESIAN_POINT('Ctrl Pts',(2.25484807009596,-23.6987456198967,5.65376661203513));
#3663=CARTESIAN_POINT('Ctrl Pts',(2.82558550724686,-24.0618452707057,5.71105827870177));
#3664=CARTESIAN_POINT('Ctrl Pts',(3.30641598130079,-24.5684600530816,5.76834994536854));
#3665=CARTESIAN_POINT('Ctrl Pts',(3.64022523789207,-25.1607744556708,5.82564161203513));
#3666=CARTESIAN_POINT('Ctrl Pts',(3.97403449448334,-25.75308885826,5.88293327870172));
#3667=CARTESIAN_POINT('Ctrl Pts',(4.16013667989657,-26.4299948886844,5.94022494536852));
#3668=CARTESIAN_POINT('Ctrl Pts',(4.17531508496597,-27.1131792176834,5.99751661203513));
#3669=CARTESIAN_POINT('Ctrl Pts',(4.19049349003537,-27.7963635466825,6.05480827870174));
#3670=CARTESIAN_POINT('Ctrl Pts',(4.03466554977154,-28.4845190963707,6.11209994536826));
#3671=CARTESIAN_POINT('Ctrl Pts',(3.72437307967983,-29.0972342682174,6.16939161203513));
#3672=CARTESIAN_POINT('Ctrl Pts',(3.41408060958811,-29.7099494400641,6.226683278702));
#3673=CARTESIAN_POINT('Ctrl Pts',(2.94987006045165,-30.2460267468577,6.28397494536819));
#3674=CARTESIAN_POINT('Ctrl Pts',(2.38451347927363,-30.642040849772,6.34126661203513));
#3675=CARTESIAN_POINT('Ctrl Pts',(1.81915689809562,-31.0380549526863,6.39855827870207));
#3676=CARTESIAN_POINT('Ctrl Pts',(1.15370619622606,-31.2932036869398,6.45584994536854));
#3677=CARTESIAN_POINT('Ctrl Pts',(0.46499000905991,-31.3762881576128,6.51314161203513));
#3678=CARTESIAN_POINT('Ctrl Pts',(-0.223726178106243,-31.4593726282858,
6.57043327870172));
#3679=CARTESIAN_POINT('Ctrl Pts',(-0.934395434881118,-31.3701806092124,
6.62772494536832));
#3680=CARTESIAN_POINT('Ctrl Pts',(-1.58414485255466,-31.1174745755294,6.68501661203513));
#3681=CARTESIAN_POINT('Ctrl Pts',(-2.2338942702282,-30.8647685418463,6.74230827870194));
#3682=CARTESIAN_POINT('Ctrl Pts',(-2.82146025502991,-30.4489825235109,6.79959994536846));
#3683=CARTESIAN_POINT('Ctrl Pts',(-3.27755388640684,-29.9171566859563,6.85689161203513));
#3684=CARTESIAN_POINT('Ctrl Pts',(-3.73364751778377,-29.3853308484018,6.9141832787018));
#3685=CARTESIAN_POINT('Ctrl Pts',(-4.05735481460304,-28.7384487328433,6.97147494536818));
#3686=CARTESIAN_POINT('Ctrl Pts',(-4.20956618239513,-28.0510324500818,7.02876661203513));
#3687=CARTESIAN_POINT('Ctrl Pts',(-4.36177755018722,-27.3636161673202,7.08605827870208));
#3688=CARTESIAN_POINT('Ctrl Pts',(-4.34214927877063,-26.6369704507106,7.14334994536865));
#3689=CARTESIAN_POINT('Ctrl Pts',(-4.15133955546951,-25.9556670914478,7.20064161203513));
#3690=CARTESIAN_POINT('Ctrl Pts',(-3.96052983216839,-25.2743637321851,7.25793327870161));
#3691=CARTESIAN_POINT('Ctrl Pts',(-3.59885249650757,-24.6397217483839,7.31522494536868));
#3692=CARTESIAN_POINT('Ctrl Pts',(-3.10696747601062,-24.1263712215646,7.37251661203513));
#3693=CARTESIAN_POINT('Ctrl Pts',(-2.61508245551368,-23.6130206947453,7.42980827870158));
#3694=CARTESIAN_POINT('Ctrl Pts',(-1.99389298437356,-23.2219816237259,7.48709994536824));
#3695=CARTESIAN_POINT('Ctrl Pts',(-1.31479298203775,-23.0001174989155,7.54439161203513));
#3696=CARTESIAN_POINT('Ctrl Pts',(-0.635692979701941,-22.778253374105,7.60168327870201));
#3697=CARTESIAN_POINT('Ctrl Pts',(0.100033826104315,-22.7260398903107,7.65897494536861));
#3698=CARTESIAN_POINT('Ctrl Pts',(0.806919301404371,-22.8511723860526,7.71626661203513));
#3699=CARTESIAN_POINT('Ctrl Pts',(1.51380477670443,-22.9763048817946,7.77355827870165));
#3700=CARTESIAN_POINT('Ctrl Pts',(2.19048605403487,-23.2785964484885,7.83084994536837));
#3701=CARTESIAN_POINT('Ctrl Pts',(2.75758559358357,-23.7243675667894,7.88814161203513));
#3702=CARTESIAN_POINT('Ctrl Pts',(3.32468513313228,-24.1701386850904,7.94543327870189));
#3703=CARTESIAN_POINT('Ctrl Pts',(3.7810839941741,-24.758577873874,8.00272494536833));
#3704=CARTESIAN_POINT('Ctrl Pts',(4.07240751844243,-25.4222319932947,8.06001661203513));
#3705=CARTESIAN_POINT('Ctrl Pts',(4.36373104271076,-26.0858861127153,8.11730827870193));
#3706=CARTESIAN_POINT('Ctrl Pts',(4.48937241387869,-26.8235059315532,8.17459994536906));
#3707=CARTESIAN_POINT('Ctrl Pts',(4.43311397861856,-27.5495620107739,8.23189161203513));
#3708=CARTESIAN_POINT('Ctrl Pts',(4.37685554335844,-28.2756180899945,8.28918327870121));
#3709=CARTESIAN_POINT('Ctrl Pts',(4.13875166853063,-28.9887160799575,8.34647494536867));
#3710=CARTESIAN_POINT('Ctrl Pts',(3.74495726994493,-29.6053914535565,8.40376661203513));
#3711=CARTESIAN_POINT('Ctrl Pts',(3.35116287135924,-30.2220668271555,8.46105827870158));
#3712=CARTESIAN_POINT('Ctrl Pts',(2.80238685862471,-30.7411100129369,8.51834994536943));
#3713=CARTESIAN_POINT('Ctrl Pts',(2.16134711192264,-31.1009635085778,8.57564161203513));
#3714=CARTESIAN_POINT('Ctrl Pts',(1.52030736522058,-31.4608170042187,8.63293327870082));
#3715=CARTESIAN_POINT('Ctrl Pts',(0.788205101607957,-31.6607451262615,8.69022494536734));
#3716=CARTESIAN_POINT('Ctrl Pts',(0.0497716862188113,-31.6759235313513,
8.74751661203513));
#3717=CARTESIAN_POINT('Ctrl Pts',(-0.688661729170334,-31.6911019364411,
8.80480827870292));
#3718=CARTESIAN_POINT('Ctrl Pts',(-1.43201351203358,-31.521448059472,8.86209994536876));
#3719=CARTESIAN_POINT('Ctrl Pts',(-2.09345402800635,-31.1851113503655,8.91939161203513));
#3720=CARTESIAN_POINT('Ctrl Pts',(-2.75489454397912,-30.848774641259,8.9766832787015));
#3721=CARTESIAN_POINT('Ctrl Pts',(-3.33313308108255,-30.3463513803362,9.03397494536822));
#3722=CARTESIAN_POINT('Ctrl Pts',(-3.75984193180906,-29.735056862734,9.09126661203513));
#3723=CARTESIAN_POINT('Ctrl Pts',(-4.18655078253556,-29.1237623451318,9.14855827870204));
#3724=CARTESIAN_POINT('Ctrl Pts',(-4.46086905468824,-28.404736373781,9.20584994536822));
#3725=CARTESIAN_POINT('Ctrl Pts',(-4.54936888283525,-27.661037139687,9.26314161203513));
#3726=CARTESIAN_POINT('Ctrl Pts',(-4.63786871098225,-26.9173379055931,9.32043327870204));
#3727=CARTESIAN_POINT('Ctrl Pts',(-4.54032750779717,-26.1503830218042,9.3777249453685));
#3728=CARTESIAN_POINT('Ctrl Pts',(-4.26647856412511,-25.4495901040262,9.43501661203513));
#3729=CARTESIAN_POINT('Ctrl Pts',(-3.99262962045306,-24.7487971862483,9.49230827870176));
#3730=CARTESIAN_POINT('Ctrl Pts',(-3.54294741821143,-24.1155274882508,9.54959994536835));
#3731=CARTESIAN_POINT('Ctrl Pts',(-2.96841345935235,-23.6243842074993,9.60689161203513));
#3732=CARTESIAN_POINT('Ctrl Pts',(-2.39387950049327,-23.1332409267478,9.66418327870191));
#3733=CARTESIAN_POINT('Ctrl Pts',(-1.69555903830894,-22.7852051038845,9.72147494536834));
#3734=CARTESIAN_POINT('Ctrl Pts',(-0.953955264873529,-22.6222151740227,
9.77876661203513));
#3735=CARTESIAN_POINT('Ctrl Pts',(-0.212351491438118,-22.4592252441609,
9.83605827870193));
#3736=CARTESIAN_POINT('Ctrl Pts',(0.571127184652931,-22.4816455398733,9.89334994536808));
#3737=CARTESIAN_POINT('Ctrl Pts',(1.30530062319683,-22.6884932263666,9.95064161203513));
#3738=CARTESIAN_POINT('Ctrl Pts',(2.03947406174072,-22.89534091286,10.0079332787022));
#3739=CARTESIAN_POINT('Ctrl Pts',(2.72292208988536,-23.2862714657652,10.0652249453684));
#3740=CARTESIAN_POINT('Ctrl Pts',(3.27533962034631,-23.8172234898833,10.1225166120351));
#3741=CARTESIAN_POINT('Ctrl Pts',(3.82775715080726,-24.3481755140014,10.1798082787018));
#3742=CARTESIAN_POINT('Ctrl Pts',(4.24804943901783,-25.0181710295281,10.2370999453679));
#3743=CARTESIAN_POINT('Ctrl Pts',(4.48595152705308,-25.7501411111225,10.2943916120351));
#3744=CARTESIAN_POINT('Ctrl Pts',(4.72385361508833,-26.4821111927169,10.3516832787023));
#3745=CARTESIAN_POINT('Ctrl Pts',(4.7788591231067,-27.2746709580248,10.4089749453667));
#3746=CARTESIAN_POINT('Ctrl Pts',(4.64294806533411,-28.035743924001,10.4662666120351));
#3747=CARTESIAN_POINT('Ctrl Pts',(4.50703700756152,-28.7968168899771,10.5235582787035));
#3748=CARTESIAN_POINT('Ctrl Pts',(4.18041691475187,-29.5249365139219,10.5808499453678));
#3749=CARTESIAN_POINT('Ctrl Pts',(3.69959614710895,-30.1347441747844,10.6381416120351));
#3750=CARTESIAN_POINT('Ctrl Pts',(3.21877537946604,-30.7445518356469,10.6954332787024));
#3751=CARTESIAN_POINT('Ctrl Pts',(2.58463247743366,-31.2348468805496,10.7527249453679));
#3752=CARTESIAN_POINT('Ctrl Pts',(1.86993485792894,-31.5473133148429,10.8100166120351));
#3753=CARTESIAN_POINT('Ctrl Pts',(1.15523723842421,-31.8597797491362,10.8673082787024));
#3754=CARTESIAN_POINT('Ctrl Pts',(0.361331792548353,-31.9937703043426,10.9245999453685));
#3755=CARTESIAN_POINT('Ctrl Pts',(-0.419707333596513,-31.9320965116456,
10.9818916120351));
#3756=CARTESIAN_POINT('Ctrl Pts',(-1.20074645974138,-31.8704227189487,11.0391832787018));
#3757=CARTESIAN_POINT('Ctrl Pts',(-1.96741971917488,-31.613149306151,11.0964749453686));
#3758=CARTESIAN_POINT('Ctrl Pts',(-2.63003302921232,-31.1886601597866,11.1537666120351));
#3759=CARTESIAN_POINT('Ctrl Pts',(-3.29264633924977,-30.7641710134222,11.2110582787017));
#3760=CARTESIAN_POINT('Ctrl Pts',(-3.84990223677302,-30.1732337703105,11.2683499453688));
#3761=CARTESIAN_POINT('Ctrl Pts',(-4.23579997145888,-29.4834686795161,11.3256416120351));
#3762=CARTESIAN_POINT('Ctrl Pts',(-4.62169770614474,-28.7937035887216,11.3829332787015));
#3763=CARTESIAN_POINT('Ctrl Pts',(-4.83545289018665,-28.0064050826244,11.4402249455077));
#3764=CARTESIAN_POINT('Ctrl Pts',(-4.85063010478977,-27.2127235347731,11.4975165438617));
#3765=CARTESIAN_POINT('Ctrl Pts',(-3.49999867141204,-27.1131792015256,-0.497516610416937));
#3766=CARTESIAN_POINT('Ctrl Pts',(-3.49888932799759,-26.5404932488512,-0.440224943750252));
#3767=CARTESIAN_POINT('Ctrl Pts',(-3.35444114738347,-25.9668063623456,-0.382933277083632));
#3768=CARTESIAN_POINT('Ctrl Pts',(-2.80930434430968,-24.9516337619221,-0.268349943750243));
#3769=CARTESIAN_POINT('Ctrl Pts',(-2.40908999522195,-24.5111444093371,-0.211058277083598));
#3770=CARTESIAN_POINT('Ctrl Pts',(-1.44403096339936,-23.8689809726516,-0.0964749437502769));
#3771=CARTESIAN_POINT('Ctrl Pts',(-0.880079720887058,-23.6679656879623,
-0.0391832770835939));
#3772=CARTESIAN_POINT('Ctrl Pts',(0.28061299005863,-23.5558768567235,0.0754000562497192));
#3773=CARTESIAN_POINT('Ctrl Pts',(0.876249383825206,-23.6449638021555,0.132691722916406));
#3774=CARTESIAN_POINT('Ctrl Pts',(1.95910771378206,-24.0958998985319,0.247275056249719));
#3775=CARTESIAN_POINT('Ctrl Pts',(2.44527330196474,-24.4573671339349,0.304566722916428));
#3776=CARTESIAN_POINT('Ctrl Pts',(3.19208049125558,-25.370851664545,0.419150056249697));
#3777=CARTESIAN_POINT('Ctrl Pts',(3.4519663191088,-25.9220290742938,0.476441722916301));
#3778=CARTESIAN_POINT('Ctrl Pts',(3.68132515309603,-27.08646641491,0.591025056249824));
#3779=CARTESIAN_POINT('Ctrl Pts',(3.65052625709869,-27.6986228841538,0.648316722916396));
#3780=CARTESIAN_POINT('Ctrl Pts',(3.30188598195419,-28.8402927016588,0.762900056249729));
#3781=CARTESIAN_POINT('Ctrl Pts',(2.98432689255302,-29.3686983876925,0.820191722916372));
#3782=CARTESIAN_POINT('Ctrl Pts',(2.13379081833063,-30.216096764043,0.934775056249753));
#3783=CARTESIAN_POINT('Ctrl Pts',(1.60158961081322,-30.5342409823362,0.992066722916289));
#3784=CARTESIAN_POINT('Ctrl Pts',(0.445414171550833,-30.8826444452813,1.10665005624984));
#3785=CARTESIAN_POINT('Ctrl Pts',(-0.177469596581333,-30.912519185481,1.16394172291647));
#3786=CARTESIAN_POINT('Ctrl Pts',(-1.36813499365341,-30.6734189584949,1.27852505624965));
#3787=CARTESIAN_POINT('Ctrl Pts',(-1.93476718568864,-30.4046202185468,1.33581672291637));
#3788=CARTESIAN_POINT('Ctrl Pts',(-2.87746776648538,-29.6280956550586,1.45040005624976));
#3789=CARTESIAN_POINT('Ctrl Pts',(-3.25260040831661,-29.1210712820873,1.50769172291632));
#3790=CARTESIAN_POINT('Ctrl Pts',(-3.72057981489945,-27.9854713421496,1.6222750562498));
#3791=CARTESIAN_POINT('Ctrl Pts',(-3.81292945777313,-27.3579616111638,1.67956672291639));
#3792=CARTESIAN_POINT('Ctrl Pts',(-3.68965542200644,-26.1289750303032,1.79415005624974));
#3793=CARTESIAN_POINT('Ctrl Pts',(-3.47409640017873,-25.5286790803258,1.85144172291645));
#3794=CARTESIAN_POINT('Ctrl Pts',(-2.78220129939746,-24.4971784172052,1.96602505624967));
#3795=CARTESIAN_POINT('Ctrl Pts',(-2.30648258548237,-24.0669901790178,2.02331672291636));
#3796=CARTESIAN_POINT('Ctrl Pts',(-1.20394886875872,-23.4801893728762,2.13790005624977));
#3797=CARTESIAN_POINT('Ctrl Pts',(-0.578163322834367,-23.3241853462944,
2.1951917229164));
#3798=CARTESIAN_POINT('Ctrl Pts',(0.677706727587892,-23.3264040337203,2.30977505624973));
#3799=CARTESIAN_POINT('Ctrl Pts',(1.30658986109621,-23.4846781506972,2.36706672291644));
#3800=CARTESIAN_POINT('Ctrl Pts',(2.4192131498232,-24.0819034318477,2.48165005624969));
#3801=CARTESIAN_POINT('Ctrl Pts',(2.9018637326796,-24.5203304926646,2.53894172291615));
#3802=CARTESIAN_POINT('Ctrl Pts',(3.60541666501523,-25.5772653974027,2.65352505624997));
#3803=CARTESIAN_POINT('Ctrl Pts',(3.82560148759511,-26.1947919093305,2.71081672291652));
#3804=CARTESIAN_POINT('Ctrl Pts',(3.94852103377322,-27.4654507141961,2.8254000562496));
#3805=CARTESIAN_POINT('Ctrl Pts',(3.85108490425945,-28.1173727349135,2.88269172291611));
#3806=CARTESIAN_POINT('Ctrl Pts',(3.35786298785392,-29.3023180651413,2.99727505625001));
#3807=CARTESIAN_POINT('Ctrl Pts',(2.96249956859728,-29.8341873664785,3.05456672291645));
#3808=CARTESIAN_POINT('Ctrl Pts',(1.96359879532417,-30.6510938545388,3.16915005624968));
#3809=CARTESIAN_POINT('Ctrl Pts',(1.36098303900346,-30.9353082084263,3.22644172291641));
#3810=CARTESIAN_POINT('Ctrl Pts',(0.0881707169855854,-31.1862241665521,
3.34102505624972));
#3811=CARTESIAN_POINT('Ctrl Pts',(-0.580818711692515,-31.1526332462716,
3.39831672291618));
#3812=CARTESIAN_POINT('Ctrl Pts',(-1.82822868779995,-30.7719170447183,3.51290005624994));
#3813=CARTESIAN_POINT('Ctrl Pts',(-2.40544041813704,-30.4251047381095,3.57019172291641));
#3814=CARTESIAN_POINT('Ctrl Pts',(-3.33097280181086,-29.4964346565957,3.68477505624972));
#3815=CARTESIAN_POINT('Ctrl Pts',(-3.67837023727213,-28.9154274047545,3.74206672291629));
#3816=CARTESIAN_POINT('Ctrl Pts',(-4.05884962667304,-27.6535118068985,3.85665005624984));
#3817=CARTESIAN_POINT('Ctrl Pts',(-4.09151639110769,-26.9737950793345,3.91394172291615));
#3818=CARTESIAN_POINT('Ctrl Pts',(-3.83085904003235,-25.6747547008469,4.02852505624998));
#3819=CARTESIAN_POINT('Ctrl Pts',(-3.53773177400349,-25.0566841622527,4.08581672291636));
#3820=CARTESIAN_POINT('Ctrl Pts',(-2.69110791178932,-24.028567338781,4.20040005624976));
#3821=CARTESIAN_POINT('Ctrl Pts',(-2.13837982562106,-23.6195385131152,4.25769172291635));
#3822=CARTESIAN_POINT('Ctrl Pts',(-0.900692885453703,-23.1092732864771,
4.37227505624977));
#3823=CARTESIAN_POINT('Ctrl Pts',(-0.216897527488987,-23.0085744595606,
4.42956672291635));
#3824=CARTESIAN_POINT('Ctrl Pts',(1.12205514727662,-23.142679210215,4.54415005624977));
#3825=CARTESIAN_POINT('Ctrl Pts',(1.775926366677,-23.3774077699852,4.60144172291642));
#3826=CARTESIAN_POINT('Ctrl Pts',(2.89930290271304,-24.1306923663646,4.71602505624971));
#3827=CARTESIAN_POINT('Ctrl Pts',(3.36770385261388,-24.6485723106026,4.77331672291647));
#3828=CARTESIAN_POINT('Ctrl Pts',(4.00659313686357,-25.8485567155787,4.88790005624965));
#3829=CARTESIAN_POINT('Ctrl Pts',(4.17642310008015,-26.5295384946699,4.94519172291645));
#3830=CARTESIAN_POINT('Ctrl Pts',(4.17420441267586,-27.8959067178885,5.05977505624967));
#3831=CARTESIAN_POINT('Ctrl Pts',(4.00210435901772,-28.5799860845476,5.11706672291619));
#3832=CARTESIAN_POINT('Ctrl Pts',(3.3527905998087,-29.7900600615589,5.23165005624993));
#3833=CARTESIAN_POINT('Ctrl Pts',(2.87615082723203,-30.314871874706,5.28894172291612));
#3834=CARTESIAN_POINT('Ctrl Pts',(1.72734004962141,-31.0798143026723,5.40352505625001));
#3835=CARTESIAN_POINT('Ctrl Pts',(1.05623826824525,-31.3191686631573,5.46081672291647));
#3836=CARTESIAN_POINT('Ctrl Pts',(-0.324386630517576,-31.4529189242652,
5.57540005624965));
#3837=CARTESIAN_POINT('Ctrl Pts',(-1.03259427822014,-31.3471336106709,5.63269172291625));
#3838=CARTESIAN_POINT('Ctrl Pts',(-2.31962660867283,-30.8116258742433,5.74727505624988));
#3839=CARTESIAN_POINT('Ctrl Pts',(-2.89719962320057,-30.3823662711092,5.80456672291639));
#3840=CARTESIAN_POINT('Ctrl Pts',(-3.78420541000443,-29.2980492552136,5.91915005624974));
#3841=CARTESIAN_POINT('Ctrl Pts',(-4.09274828993971,-28.6439951522933,5.97644172291612));
#3842=CARTESIAN_POINT('Ctrl Pts',(-4.36522137220295,-27.2628078488887,6.09102505625001));
#3843=CARTESIAN_POINT('Ctrl Pts',(-4.32883842763837,-26.5369854607524,6.14831672291658));
#3844=CARTESIAN_POINT('Ctrl Pts',(-3.91604629967915,-25.1838353260752,6.26290005624954));
#3845=CARTESIAN_POINT('Ctrl Pts',(-3.53998077585005,-24.5578175514078,6.32019172291661));
#3846=CARTESIAN_POINT('Ctrl Pts',(-2.53317668706739,-23.5541511604319,6.43477505624951));
#3847=CARTESIAN_POINT('Ctrl Pts',(-1.90336339087076,-23.1775005077857,6.49206672291618));
#3848=CARTESIAN_POINT('Ctrl Pts',(-0.535707634461822,-22.7649451919414,
6.60665005624995));
#3849=CARTESIAN_POINT('Ctrl Pts',(0.200842052573385,-22.7294864032627,6.66394172291654));
#3850=CARTESIAN_POINT('Ctrl Pts',(1.60825741243838,-23.0117008784331,6.77852505624958));
#3851=CARTESIAN_POINT('Ctrl Pts',(2.27776629761871,-23.3291566705507,6.83581672291669));
#3852=CARTESIAN_POINT('Ctrl Pts',(3.39129936374918,-24.2458798314691,6.95040005624944));
#3853=CARTESIAN_POINT('Ctrl Pts',(3.8342243732566,-24.8443116308563,7.00769172291627));
#3854=CARTESIAN_POINT('Ctrl Pts',(4.38677541995195,-26.1840855712311,7.12227505624986));
#3855=CARTESIAN_POINT('Ctrl Pts',(4.49582343090945,-26.9241665562002,7.1795667229166));
#3856=CARTESIAN_POINT('Ctrl Pts',(4.35088796536903,-28.3730853248421,7.29415005624953));
#3857=CARTESIAN_POINT('Ctrl Pts',(4.09698986764256,-29.0805318136941,7.35144172291661));
#3858=CARTESIAN_POINT('Ctrl Pts',(3.28231577569086,-30.295784222617,7.46602505624951));
#3859=CARTESIAN_POINT('Ctrl Pts',(2.72227460111075,-30.8023978842609,7.52331672291659));
#3860=CARTESIAN_POINT('Ctrl Pts',(1.42483950789472,-31.4933756465881,7.63790005624954));
#3861=CARTESIAN_POINT('Ctrl Pts',(0.688661495622512,-31.6770315464534,7.69519172291528));
#3862=CARTESIAN_POINT('Ctrl Pts',(-0.788204900376376,-31.6748128590733,
7.80977505625085));
#3863=CARTESIAN_POINT('Ctrl Pts',(-1.52748050021878,-31.4888868687303,7.86706672291669));
#3864=CARTESIAN_POINT('Ctrl Pts',(-2.83500516546561,-30.7874846314674,7.98165005624943));
#3865=CARTESIAN_POINT('Ctrl Pts',(-3.40197820894101,-30.2726321471241,8.03894172291615));
#3866=CARTESIAN_POINT('Ctrl Pts',(-4.22831013251146,-29.0319454966501,8.15352505624997));
#3867=CARTESIAN_POINT('Ctrl Pts',(-4.48683403091752,-28.3072684458016,8.21081672291615));
#3868=CARTESIAN_POINT('Ctrl Pts',(-4.63141500694981,-26.8166774531803,8.32540005624997));
#3869=CARTESIAN_POINT('Ctrl Pts',(-4.51728050926608,-26.0521841784596,8.38269172291643));
#3870=CARTESIAN_POINT('Ctrl Pts',(-3.93948695283954,-24.6630648478093,8.49727505624969));
#3871=CARTESIAN_POINT('Ctrl Pts',(-3.47633116581651,-24.0397881200713,8.55456672291628));
#3872=CARTESIAN_POINT('Ctrl Pts',(-2.3065979072983,-23.082683034536,8.66915005624984));
#3873=CARTESIAN_POINT('Ctrl Pts',(-1.60110545776092,-22.7498116285361,8.72644172291626));
#3874=CARTESIAN_POINT('Ctrl Pts',(-0.1115431730045,-22.455781422157,8.84102505624986));
#3875=CARTESIAN_POINT('Ctrl Pts',(0.671112174616573,-22.4949563909962,8.89831672291601));
#3876=CARTESIAN_POINT('Ctrl Pts',(2.13000246784507,-22.9398244453587,9.01290005625012));
#3877=CARTESIAN_POINT('Ctrl Pts',(2.80482628686612,-23.3451431864166,9.07019172291636));
#3878=CARTESIAN_POINT('Ctrl Pts',(3.88662668511606,-24.4300812824538,9.18477505624977));
#3879=CARTESIAN_POINT('Ctrl Pts',(4.29253055496877,-25.1087006230277,9.24206672291584));
#3880=CARTESIAN_POINT('Ctrl Pts',(4.73716179724122,-26.5820965379602,9.35665005625028));
#3881=CARTESIAN_POINT('Ctrl Pts',(4.77541261016421,-27.3754791844964,9.41394172291549));
#3882=CARTESIAN_POINT('Ctrl Pts',(4.47164101091353,-28.8912695257086,9.52852505625063));
#3883=CARTESIAN_POINT('Ctrl Pts',(4.12985669269715,-29.6122167575113,9.58581672291576));
#3884=CARTESIAN_POINT('Ctrl Pts',(3.1430342330799,-30.8111660662582,9.70040005625036));
#3885=CARTESIAN_POINT('Ctrl Pts',(2.49889872045615,-31.2879872596437,9.75769172291579));
#3886=CARTESIAN_POINT('Ctrl Pts',(1.05703777990366,-31.8828241263658,9.87227505625033));
#3887=CARTESIAN_POINT('Ctrl Pts',(0.260671167899412,-32.0002213213825,9.92956672291638));
#3888=CARTESIAN_POINT('Ctrl Pts',(-1.29821369458701,-31.8444551409501,10.0441500562497));
#3889=CARTESIAN_POINT('Ctrl Pts',(-2.05923545291888,-31.5713875052691,10.1014417229165));
#3890=CARTESIAN_POINT('Ctrl Pts',(-3.36636373470387,-30.6953239177476,10.2160250562496));
#3891=CARTESIAN_POINT('Ctrl Pts',(-3.91119010810414,-30.0931215128015,10.2733167229167));
#3892=CARTESIAN_POINT('Ctrl Pts',(-4.65425634850692,-28.6982357313908,10.3879000562494));
#3893=CARTESIAN_POINT('Ctrl Pts',(-4.85173818484261,-27.906861497377,10.4451917229149));
#3894=CARTESIAN_POINT('Ctrl Pts',(-4.85062884134398,-27.1131792015253,10.5024833895831));
#3895=CARTESIAN_POINT('Ctrl Pts',(-4.49992531496781,-27.1253399927944,-0.498733179016745));
#3896=CARTESIAN_POINT('Ctrl Pts',(-4.50080577640339,-26.3890414230237,-0.441441512350059));
#3897=CARTESIAN_POINT('Ctrl Pts',(-4.31740187521755,-25.6514004960575,-0.38414984568344));
#3898=CARTESIAN_POINT('Ctrl Pts',(-3.62152187059884,-24.3457650353575,-0.26956651235005));
#3899=CARTESIAN_POINT('Ctrl Pts',(-3.10966424169642,-23.7790447241712,-0.212274845683405));
#3900=CARTESIAN_POINT('Ctrl Pts',(-1.87473833045347,-22.9517757677986,-0.0976915123500845));
#3901=CARTESIAN_POINT('Ctrl Pts',(-1.15282164350167,-22.6920629943005,-0.0403998456834014));
#3902=CARTESIAN_POINT('Ctrl Pts',(0.333130544922134,-22.5439400354353,0.0741834876499117));
#3903=CARTESIAN_POINT('Ctrl Pts',(1.09574982783323,-22.6557248123599,0.131475154316599));
#3904=CARTESIAN_POINT('Ctrl Pts',(2.48244777760786,-23.2282079016538,0.246058487649911));
#3905=CARTESIAN_POINT('Ctrl Pts',(3.10517944279315,-23.68840802634,0.30335015431662));
#3906=CARTESIAN_POINT('Ctrl Pts',(4.06265239793424,-24.85231643994,0.41793348764989));
#3907=CARTESIAN_POINT('Ctrl Pts',(4.3964363912496,-25.5549452872785,0.475225154316493));
#3908=CARTESIAN_POINT('Ctrl Pts',(4.69353684255108,-27.0395439300089,0.589808487650017));
#3909=CARTESIAN_POINT('Ctrl Pts',(4.65651659660415,-27.8201039966141,0.647100154316588));
#3910=CARTESIAN_POINT('Ctrl Pts',(4.21669610116961,-29.276064051845,0.761683487649922));
#3911=CARTESIAN_POINT('Ctrl Pts',(3.8142653646997,-29.950055727301,0.818975154316564));
#3912=CARTESIAN_POINT('Ctrl Pts',(2.73516012282014,-31.0316512891878,0.933558487649946));
#3913=CARTESIAN_POINT('Ctrl Pts',(2.05948004468961,-31.4381826698554,0.990850154316524));
#3914=CARTESIAN_POINT('Ctrl Pts',(0.591324807038797,-31.8853828510085,1.10543348764999));
#3915=CARTESIAN_POINT('Ctrl Pts',(-0.199761447971984,-31.9255726377888,
1.16272515431667));
#3916=CARTESIAN_POINT('Ctrl Pts',(-1.71214091388154,-31.6265370785213,1.27730848764984));
#3917=CARTESIAN_POINT('Ctrl Pts',(-2.43197693509141,-31.2875452940623,1.33460015431656));
#3918=CARTESIAN_POINT('Ctrl Pts',(-3.63015067419501,-30.306507524294,1.44918348764995));
#3919=CARTESIAN_POINT('Ctrl Pts',(-4.10730825861232,-29.6653586276362,1.50647515431652));
#3920=CARTESIAN_POINT('Ctrl Pts',(-4.70418801790555,-28.2289649290438,1.62105848764999));
#3921=CARTESIAN_POINT('Ctrl Pts',(-4.82328976434201,-27.4350737035586,1.67835015431658));
#3922=CARTESIAN_POINT('Ctrl Pts',(-4.67190249432477,-25.8800475050968,1.79293348764993));
#3923=CARTESIAN_POINT('Ctrl Pts',(-4.40150502792665,-25.1204053228213,1.85022515431664));
#3924=CARTESIAN_POINT('Ctrl Pts',(-3.53112225622387,-23.8146158747871,1.96480848764987));
#3925=CARTESIAN_POINT('Ctrl Pts',(-2.93192505802151,-23.2697474697807,2.02210015431647));
#3926=CARTESIAN_POINT('Ctrl Pts',(-1.54268043071708,-22.5251840572753,2.13668348765005));
#3927=CARTESIAN_POINT('Ctrl Pts',(-0.753936727410522,-22.3262485075428,
2.19397515431668));
#3928=CARTESIAN_POINT('Ctrl Pts',(0.82915854962663,-22.3244875853603,2.30855848764983));
#3929=CARTESIAN_POINT('Ctrl Pts',(1.62199572723047,-22.5217174227832,2.36585015431672));
#3930=CARTESIAN_POINT('Ctrl Pts',(3.02508187654173,-23.2696859056385,2.48043348764979));
#3931=CARTESIAN_POINT('Ctrl Pts',(3.63396341774869,-23.8197562460487,2.53772515431626));
#3932=CARTESIAN_POINT('Ctrl Pts',(4.52262186996503,-25.1465580304901,2.65230848765025));
#3933=CARTESIAN_POINT('Ctrl Pts',(4.80150418123824,-25.9220499865487,2.70960015431671));
#3934=CARTESIAN_POINT('Ctrl Pts',(4.96045785508009,-27.5179682692268,2.8241834876498));
#3935=CARTESIAN_POINT('Ctrl Pts',(4.84032389411636,-28.3368731787678,2.88147515431622));
#3936=CARTESIAN_POINT('Ctrl Pts',(4.22555498467076,-29.8256581291208,2.99605848765029));
#3937=CARTESIAN_POINT('Ctrl Pts',(3.7314586763185,-30.4940935072009,3.05335015431664));
#3938=CARTESIAN_POINT('Ctrl Pts',(2.48213401980284,-31.5216657613235,3.16793348764987));
#3939=CARTESIAN_POINT('Ctrl Pts',(1.72806682617598,-31.8797782805327,3.2252251543166));
#3940=CARTESIAN_POINT('Ctrl Pts',(0.13509320172947,-32.1984358560416,3.33980848764991));
#3941=CARTESIAN_POINT('Ctrl Pts',(-0.702299823999385,-32.1586235858217,
3.39710015431637));
#3942=CARTESIAN_POINT('Ctrl Pts',(-2.26400003813965,-31.6867271638891,3.51168348765014));
#3943=CARTESIAN_POINT('Ctrl Pts',(-2.98679775763238,-31.2550432103659,3.5689751543166));
#3944=CARTESIAN_POINT('Ctrl Pts',(-4.14652732706892,-30.0978039609755,3.68355848764991));
#3945=CARTESIAN_POINT('Ctrl Pts',(-4.58231192474403,-29.3733178387791,3.74085015431648));
#3946=CARTESIAN_POINT('Ctrl Pts',(-5.06158803244764,-27.7994224422382,3.85543348765003));
#3947=CARTESIAN_POINT('Ctrl Pts',(-5.10456984344478,-26.9515032280969,3.91272515431634));
#3948=CARTESIAN_POINT('Ctrl Pts',(-4.78397716002945,-25.3307487804658,4.02730848765017));
#3949=CARTESIAN_POINT('Ctrl Pts',(-4.42065684961388,-24.5594744129683,4.08460015431674));
#3950=CARTESIAN_POINT('Ctrl Pts',(-3.36951978092995,-23.275884430953,4.19918348764977));
#3951=CARTESIAN_POINT('Ctrl Pts',(-2.68266717130709,-22.764830662879,4.25647515431655));
#3952=CARTESIAN_POINT('Ctrl Pts',(-1.14418647221071,-22.1256650834116,4.37105848764996));
#3953=CARTESIAN_POINT('Ctrl Pts',(-0.294009620031413,-21.9982141529788,
4.42835015431673));
#3954=CARTESIAN_POINT('Ctrl Pts',(1.3709826726307,-22.1604321379097,4.54293348764978));
#3955=CARTESIAN_POINT('Ctrl Pts',(2.18420012405877,-22.4499991421574,4.60022515431661));
#3956=CARTESIAN_POINT('Ctrl Pts',(3.58186544525391,-23.3817714096182,4.7148084876499));
#3957=CARTESIAN_POINT('Ctrl Pts',(4.16494656178229,-24.0231298379359,4.77210015431648));
#3958=CARTESIAN_POINT('Ctrl Pts',(4.96159845253322,-25.5098251537481,4.88668348765003));
#3959=CARTESIAN_POINT('Ctrl Pts',(5.17435993882992,-26.3537650899519,4.94397515431683));
#3960=CARTESIAN_POINT('Ctrl Pts',(5.17612086103765,-28.0473585400691,5.05855848764968));
#3961=CARTESIAN_POINT('Ctrl Pts',(4.96506508699686,-28.8953919505567,5.11585015431639));
#3962=CARTESIAN_POINT('Ctrl Pts',(4.16500812595277,-30.3959287884026,5.23043348765012));
#3963=CARTESIAN_POINT('Ctrl Pts',(3.57672507396265,-31.0469715596972,5.28772515431631));
#3964=CARTESIAN_POINT('Ctrl Pts',(2.15804741641932,-31.9970195077,5.4023084876502));
#3965=CARTESIAN_POINT('Ctrl Pts',(1.32898019116406,-32.2950713567837,5.45960015431648));
#3966=CARTESIAN_POINT('Ctrl Pts',(-0.376904185685347,-32.4648557455888,
5.57418348765003));
#3967=CARTESIAN_POINT('Ctrl Pts',(-1.25209472194662,-32.3363726005772,5.63147515431663));
#3968=CARTESIAN_POINT('Ctrl Pts',(-2.84296667278025,-31.6793178710107,5.74605848764988));
#3969=CARTESIAN_POINT('Ctrl Pts',(-3.55710576383776,-31.1513253789313,5.80335015431639));
#3970=CARTESIAN_POINT('Ctrl Pts',(-4.65477731687436,-29.8165844795914,5.91793348765012));
#3971=CARTESIAN_POINT('Ctrl Pts',(-5.03721836201938,-29.0110789395971,5.97522515431631));
#3972=CARTESIAN_POINT('Ctrl Pts',(-5.37743306171915,-27.3097303335012,6.0898084876502));
#3973=CARTESIAN_POINT('Ctrl Pts',(-5.33482876722501,-26.4155043485724,6.14710015431696));
#3974=CARTESIAN_POINT('Ctrl Pts',(-4.83085641881337,-24.7480639756086,6.26168348764955));
#3975=CARTESIAN_POINT('Ctrl Pts',(-4.36991924819774,-23.9764602120055,6.31897515431661));
#3976=CARTESIAN_POINT('Ctrl Pts',(-3.13454599135584,-22.7385966350808,6.4335584876499));
#3977=CARTESIAN_POINT('Ctrl Pts',(-2.36125382501729,-22.2735588203518,6.49085015431656));
#3978=CARTESIAN_POINT('Ctrl Pts',(-0.681618269679574,-21.7622067861288,
6.60543348764995));
#3979=CARTESIAN_POINT('Ctrl Pts',(0.223133903687647,-21.7164329509015,6.66272515431674));
#3980=CARTESIAN_POINT('Ctrl Pts',(1.95226333294297,-22.0585827584601,6.77730848764977));
#3981=CARTESIAN_POINT('Ctrl Pts',(2.77497604680507,-22.4462315948605,6.83460015431688));
#3982=CARTESIAN_POINT('Ctrl Pts',(4.14398227167528,-23.5674679624083,6.94918348764963));
#3983=CARTESIAN_POINT('Ctrl Pts',(4.68893222344454,-24.3000242850548,7.00647515431646));
#3984=CARTESIAN_POINT('Ctrl Pts',(5.37038362306584,-25.9405919845896,7.12105848765005));
#3985=CARTESIAN_POINT('Ctrl Pts',(5.50618373750129,-26.8470544635367,7.17835015431679));
#3986=CARTESIAN_POINT('Ctrl Pts',(5.33313503766439,-28.6220128503173,7.29293348764972));
#3987=CARTESIAN_POINT('Ctrl Pts',(5.02439849553529,-29.4888055709765,7.3502251543168));
#3988=CARTESIAN_POINT('Ctrl Pts',(4.03123673237243,-30.9783467652573,7.46480848764971));
#3989=CARTESIAN_POINT('Ctrl Pts',(3.34771707388356,-31.5996405933702,7.52210015431658));
#3990=CARTESIAN_POINT('Ctrl Pts',(1.76357106961933,-32.4483809623168,7.63668348764993));
#3991=CARTESIAN_POINT('Ctrl Pts',(0.864434900460165,-32.6749683852002,7.69397515431566));
#3992=CARTESIAN_POINT('Ctrl Pts',(-0.939656722676682,-32.676729307438,7.80855848765085));
#3993=CARTESIAN_POINT('Ctrl Pts',(-1.84288636612563,-32.4518475967632,7.86585015431688));
#3994=CARTESIAN_POINT('Ctrl Pts',(-3.44087389241161,-31.5997021575577,7.98043348764962));
#3995=CARTESIAN_POINT('Ctrl Pts',(-4.13407789386612,-30.9732063939501,8.03772515431634));
#3996=CARTESIAN_POINT('Ctrl Pts',(-5.14551533760529,-29.4626528633526,8.15230848765016));
#3997=CARTESIAN_POINT('Ctrl Pts',(-5.46273672453315,-28.5800103688324,8.20960015431635));
#3998=CARTESIAN_POINT('Ctrl Pts',(-5.64335182828418,-26.7641598979005,8.32418348765016));
#3999=CARTESIAN_POINT('Ctrl Pts',(-5.50651949921481,-25.8326837348359,8.38147515431663));
#4000=CARTESIAN_POINT('Ctrl Pts',(-4.80717894956453,-24.139724783599,8.49605848764988));
#4001=CARTESIAN_POINT('Ctrl Pts',(-4.24529027372504,-23.379881979507,8.55335015431647));
#4002=CARTESIAN_POINT('Ctrl Pts',(-2.82513313158961,-22.2121111275932,8.66793348765004));
#4003=CARTESIAN_POINT('Ctrl Pts',(-1.96818924517237,-21.8053415564794,8.72522515431646));
#4004=CARTESIAN_POINT('Ctrl Pts',(-0.158465657509371,-21.4435697326178,
8.83980848765005));
#4005=CARTESIAN_POINT('Ctrl Pts',(0.792593286692538,-21.4889660513795,8.8971001543162));
#4006=CARTESIAN_POINT('Ctrl Pts',(2.56577381841575,-22.0250143262545,9.01168348765031));
#4007=CARTESIAN_POINT('Ctrl Pts',(3.38618362619219,-22.5152047139933,9.06897515431655));
#4008=CARTESIAN_POINT('Ctrl Pts',(4.70218121054346,-23.828711978241,9.18355848764996));
#4009=CARTESIAN_POINT('Ctrl Pts',(5.19647224236993,-24.6508101887781,9.24085015431603));
#4010=CARTESIAN_POINT('Ctrl Pts',(5.73990020308659,-26.4361859028455,9.35543348765047));
#4011=CARTESIAN_POINT('Ctrl Pts',(5.78846606254352,-27.3977710355077,9.41272515431568));
#4012=CARTESIAN_POINT('Ctrl Pts',(5.42475913086839,-29.2352754463162,9.52730848765082));
#4013=CARTESIAN_POINT('Ctrl Pts',(5.01278176845109,-30.1094265066166,9.58460015431595));
#4014=CARTESIAN_POINT('Ctrl Pts',(3.82144610207693,-31.5638489742655,9.69918348765055));
#4015=CARTESIAN_POINT('Ctrl Pts',(3.04318606635087,-32.1426951097914,9.75647515431598));
#4016=CARTESIAN_POINT('Ctrl Pts',(1.30053136645192,-32.86643232952,9.87105848765053));
#4017=CARTESIAN_POINT('Ctrl Pts',(0.337783260665778,-33.0105816279838,9.92835015431657));
#4018=CARTESIAN_POINT('Ctrl Pts',(-1.54714122016509,-32.826702213236,10.0429334876499));
#4019=CARTESIAN_POINT('Ctrl Pts',(-2.4675092101147,-32.4987961332167,10.1002251543167));
#4020=CARTESIAN_POINT('Ctrl Pts',(-4.04892627743074,-31.4442448743743,10.2148084876498));
#4021=CARTESIAN_POINT('Ctrl Pts',(-4.70843281716765,-30.7185639856579,10.2721001543169));
#4022=CARTESIAN_POINT('Ctrl Pts',(-5.60926166428151,-29.0369672930318,10.3866834876496));
#4023=CARTESIAN_POINT('Ctrl Pts',(-5.84967502356038,-28.082634904679,10.4439751543151));
#4024=CARTESIAN_POINT('Ctrl Pts',(-5.85055548489976,-27.125339992794,10.5012668209833));
#4025=CARTESIAN_POINT('Ctrl Pts',(-4.49992531496781,-27.2248833652324,0.496300045053516));
#4026=CARTESIAN_POINT('Ctrl Pts',(-4.5170935228935,-26.4885847954605,0.553591711720202));
#4027=CARTESIAN_POINT('Ctrl Pts',(-4.34996178652419,-25.7468679032987,0.610883378386821));
#4028=CARTESIAN_POINT('Ctrl Pts',(-3.68281080117209,-24.4258764618724,0.725466711720211));
#4029=CARTESIAN_POINT('Ctrl Pts',(-3.18338254408968,-23.8478908247253,0.782758378386896));
#4030=CARTESIAN_POINT('Ctrl Pts',(-1.96655460663691,-22.9935363364864,0.897341711720136));
#4031=CARTESIAN_POINT('Ctrl Pts',(-1.25028920909816,-22.7180292671551,0.954633378386819));
#4032=CARTESIAN_POINT('Ctrl Pts',(0.232470022735047,-22.537487675991,1.06921671172021));
#4033=CARTESIAN_POINT('Ctrl Pts',(0.997550692859376,-22.6326791281778,1.12650837838686));
#4034=CARTESIAN_POINT('Ctrl Pts',(2.39671474379638,-23.1750663869683,1.24109171172017));
#4035=CARTESIAN_POINT('Ctrl Pts',(3.02943919783654,-23.6217927956222,1.29838337838692));
#4036=CARTESIAN_POINT('Ctrl Pts',(4.01209334897545,-24.7650355357426,1.41296671172011));
#4037=CARTESIAN_POINT('Ctrl Pts',(4.36104166103753,-25.4604921944619,1.47025837838671));
#4038=CARTESIAN_POINT('Ctrl Pts',(4.69009167559614,-26.9387356739276,1.58484171172032));
#4039=CARTESIAN_POINT('Ctrl Pts',(4.66982611111995,-27.7201188452534,1.64213337838685));
#4040=CARTESIAN_POINT('Ctrl Pts',(4.26117841813581,-29.1855350667241,1.75671671172018));
#4041=CARTESIAN_POINT('Ctrl Pts',(3.87313598265158,-29.8681507579074,1.81400837838683));
#4042=CARTESIAN_POINT('Ctrl Pts',(2.8170650922145,-30.9727806712352,1.92859171172021));
#4043=CARTESIAN_POINT('Ctrl Pts',(2.15000902980881,-31.3937003528865,1.98588337838683));
#4044=CARTESIAN_POINT('Ctrl Pts',(0.691309958401167,-31.8720733364954,2.10046671172021));
#4045=CARTESIAN_POINT('Ctrl Pts',(-0.0989531918895839,-31.929017804739,
2.15775837838676));
#4046=CARTESIAN_POINT('Ctrl Pts',(-1.61768782106606,-31.6619318087381,2.27234171172027));
#4047=CARTESIAN_POINT('Ctrl Pts',(-2.34469603088869,-31.3381043430165,2.32963337838682));
#4048=CARTESIAN_POINT('Ctrl Pts',(-3.56353544348255,-30.3822477692553,2.44421671172021));
#4049=CARTESIAN_POINT('Ctrl Pts',(-4.05416674391711,-29.751091661441,2.50150837838678));
#4050=CARTESIAN_POINT('Ctrl Pts',(-4.68114233373318,-28.3271640640242,2.61609171172026));
#4051=CARTESIAN_POINT('Ctrl Pts',(-4.81683740488648,-27.535734225746,2.67338337838684));
#4052=CARTESIAN_POINT('Ctrl Pts',(-4.69786876719058,-25.977515070693,2.78796671172019));
#4053=CARTESIAN_POINT('Ctrl Pts',(-4.44326559660206,-25.2122215990087,2.8452583783869));
#4054=CARTESIAN_POINT('Ctrl Pts',(-3.59996835679039,-23.8883341771763,2.95984171172013));
#4055=CARTESIAN_POINT('Ctrl Pts',(-3.01203648453192,-23.3310364003662,3.01713337838681));
#4056=CARTESIAN_POINT('Ctrl Pts',(-1.6381478379628,-22.5577439685697,3.13171671172022));
#4057=CARTESIAN_POINT('Ctrl Pts',(-0.853480099848572,-22.3425362536569,
3.18900837838685));
#4058=CARTESIAN_POINT('Ctrl Pts',(0.729615177188581,-22.3081998392462,3.30359171172018));
#4059=CARTESIAN_POINT('Ctrl Pts',(1.5265283199834,-22.4891575114895,3.36088337838689));
#4060=CARTESIAN_POINT('Ctrl Pts',(2.94497045003267,-23.2083969750522,3.47546671172014));
#4061=CARTESIAN_POINT('Ctrl Pts',(3.56511731717984,-23.7460379436645,3.53275837838669));
#4062=CARTESIAN_POINT('Ctrl Pts',(4.48086130129196,-25.0547417542976,3.64734171172034));
#4063=CARTESIAN_POINT('Ctrl Pts',(4.77553790836679,-25.8245824209521,3.70463337838689));
#4064=CARTESIAN_POINT('Ctrl Pts',(4.96691021454127,-27.4173077470399,3.81921671172015));
#4065=CARTESIAN_POINT('Ctrl Pts',(4.86336957828356,-28.2386740437859,3.87650837838657));
#4066=CARTESIAN_POINT('Ctrl Pts',(4.27869649937114,-29.7399250953174,3.99109171172046));
#4067=CARTESIAN_POINT('Ctrl Pts',(3.7980739070243,-30.4183532622312,4.0483833783869));
#4068=CARTESIAN_POINT('Ctrl Pts',(2.56941492401223,-31.4711067123778,4.16296671172013));
#4069=CARTESIAN_POINT('Ctrl Pts',(1.82251991899126,-31.8443835503049,4.22025837838686));
#4070=CARTESIAN_POINT('Ctrl Pts',(0.235901457812061,-32.1949906891023,4.33484171172017));
#4071=CARTESIAN_POINT('Ctrl Pts',(-0.602314672632131,-32.1719331003238,
4.39213337838664));
#4072=CARTESIAN_POINT('Ctrl Pts',(-2.17347105302534,-31.731209480869,4.5067167117204));
#4073=CARTESIAN_POINT('Ctrl Pts',(-2.90489278822714,-31.3139138283048,4.56400837838686));
#4074=CARTESIAN_POINT('Ctrl Pts',(-4.0876567091279,-30.1797089303828,4.67859171172017));
#4075=CARTESIAN_POINT('Ctrl Pts',(-4.5378296077608,-29.4638468238943,4.73588337838674));
#4076=CARTESIAN_POINT('Ctrl Pts',(-5.04827851794888,-27.8994075936046,4.85046671172029));
#4077=CARTESIAN_POINT('Ctrl Pts',(-5.10801501038022,-27.0523114841814,4.9077583783866));
#4078=CARTESIAN_POINT('Ctrl Pts',(-4.81937189026103,-25.4252018732791,5.02234171172043));
#4079=CARTESIAN_POINT('Ctrl Pts',(-4.47121589855777,-24.6467553171812,5.07963337838682));
#4080=CARTESIAN_POINT('Ctrl Pts',(-3.44526002590146,-23.3424996616552,5.19421671172021));
#4081=CARTESIAN_POINT('Ctrl Pts',(-2.76840020510825,-22.8179721775895,5.25150837838681));
#4082=CARTESIAN_POINT('Ctrl Pts',(-1.24238560719488,-22.1487107675687,5.36609171172022));
#4083=CARTESIAN_POINT('Ctrl Pts',(-0.394670142221978,-22.0046665124503,
5.42338337838681));
#4084=CARTESIAN_POINT('Ctrl Pts',(1.27351510703769,-22.1344658650278,5.53796671172023));
#4085=CARTESIAN_POINT('Ctrl Pts',(2.09238384786002,-22.4082385734949,5.59525837838687));
#4086=CARTESIAN_POINT('Ctrl Pts',(3.50814714287596,-23.3129253090387,5.70984171172016));
#4087=CARTESIAN_POINT('Ctrl Pts',(4.10365763118507,-23.9430184114309,5.76713337838693));
#4088=CARTESIAN_POINT('Ctrl Pts',(4.92903854125055,-25.4143577464969,5.8817167117201));
#4089=CARTESIAN_POINT('Ctrl Pts',(5.15807219270217,-26.2542217175139,5.93900837838691));
#4090=CARTESIAN_POINT('Ctrl Pts',(5.1924086071654,-27.947815167631,6.05359171172013));
#4091=CARTESIAN_POINT('Ctrl Pts',(4.99762499827922,-28.7999245433053,6.11088337838665));
#4092=CARTESIAN_POINT('Ctrl Pts',(4.22629705655031,-30.315817361898,6.22546671172039));
#4093=CARTESIAN_POINT('Ctrl Pts',(3.65044337633885,-30.978125459117,6.28275837838657));
#4094=CARTESIAN_POINT('Ctrl Pts',(2.24986369261982,-31.9552589390383,6.39734171172046));
#4095=CARTESIAN_POINT('Ctrl Pts',(1.42644775675681,-32.2691050839008,6.45463337838693));
#4096=CARTESIAN_POINT('Ctrl Pts',(-0.276243663494525,-32.4713081050615,
6.56921671172011));
#4097=CARTESIAN_POINT('Ctrl Pts',(-1.1538955869619,-32.3594182847329,6.6265083783867));
#4098=CARTESIAN_POINT('Ctrl Pts',(-2.75723363897965,-31.7324593857226,6.74109171172033));
#4099=CARTESIAN_POINT('Ctrl Pts',(-3.48136551885855,-31.2179406096298,6.79838337838684));
#4100=CARTESIAN_POINT('Ctrl Pts',(-4.60421826793817,-29.9038653838081,6.91296671172019));
#4101=CARTESIAN_POINT('Ctrl Pts',(-5.00182363177902,-29.1055320324077,6.97025837838657));
#4102=CARTESIAN_POINT('Ctrl Pts',(-5.37398789479249,-27.4105385895884,7.08484171172046));
#4103=CARTESIAN_POINT('Ctrl Pts',(-5.34813828171182,-26.5154894999401,7.14213337838704));
#4104=CARTESIAN_POINT('Ctrl Pts',(-4.87533873580858,-24.8385929607225,7.25671671172));
#4105=CARTESIAN_POINT('Ctrl Pts',(-4.42878986612819,-24.0583651814228,7.31400837838707));
#4106=CARTESIAN_POINT('Ctrl Pts',(-3.21645096077164,-22.7974672530097,7.42859171171997));
#4107=CARTESIAN_POINT('Ctrl Pts',(-2.45178281012867,-22.3180411373462,7.48588337838663));
#4108=CARTESIAN_POINT('Ctrl Pts',(-0.781603421049769,-21.7755163006163,
7.6004667117204));
#4109=CARTESIAN_POINT('Ctrl Pts',(0.12232564759955,-21.7129877839796,7.657758378387));
#4110=CARTESIAN_POINT('Ctrl Pts',(1.85781024013319,-22.023188028215,7.77234171172004));
#4111=CARTESIAN_POINT('Ctrl Pts',(2.68769514258573,-22.3956725459287,7.82963337838637));
#4112=CARTESIAN_POINT('Ctrl Pts',(4.07736704097944,-23.4917277174247,7.94421671172066));
#4113=CARTESIAN_POINT('Ctrl Pts',(4.6357907087237,-24.2142912512598,8.00150837838672));
#4114=CARTESIAN_POINT('Ctrl Pts',(5.34733793891911,-25.8423928495992,8.11609171172032));
#4115=CARTESIAN_POINT('Ctrl Pts',(5.4997313780195,-26.746393941348,8.17338337838705));
#4116=CARTESIAN_POINT('Ctrl Pts',(5.35910131055647,-28.5245452847223,8.28796671171998));
#4117=CARTESIAN_POINT('Ctrl Pts',(5.06615906418831,-29.3969892947731,8.34525837838706));
#4118=CARTESIAN_POINT('Ctrl Pts',(4.10008283296135,-30.904628462884,8.45984171171997));
#4119=CARTESIAN_POINT('Ctrl Pts',(3.42782850038057,-31.5383516627646,8.51713337838782));
#4120=CARTESIAN_POINT('Ctrl Pts',(1.85903847687845,-32.4158210510425,8.63171671171921));
#4121=CARTESIAN_POINT('Ctrl Pts',(0.963978272898216,-32.6586806390649,8.68900837838573));
#4122=CARTESIAN_POINT('Ctrl Pts',(-0.840113350238634,-32.6930170535733,
8.80359171172131));
#4123=CARTESIAN_POINT('Ctrl Pts',(-1.74741895886588,-32.4844075080322,8.86088337838715));
#4124=CARTESIAN_POINT('Ctrl Pts',(-3.36076246591524,-31.6609910881686,8.97546671171988));
#4125=CARTESIAN_POINT('Ctrl Pts',(-4.06523179327696,-31.0469246963195,9.03275837838661));
#4126=CARTESIAN_POINT('Ctrl Pts',(-5.10375476895253,-29.5544691395598,9.14734171172043));
#4127=CARTESIAN_POINT('Ctrl Pts',(-5.43677045163593,-28.6774779344237,9.20463337838661));
#4128=CARTESIAN_POINT('Ctrl Pts',(-5.64980418777113,-26.8648204200928,9.31921671172042));
#4129=CARTESIAN_POINT('Ctrl Pts',(-5.5295651833589,-25.9308828698286,9.37650837838689));
#4130=CARTESIAN_POINT('Ctrl Pts',(-4.86032046428803,-24.2254578173917,9.49109171172014));
#4131=CARTESIAN_POINT('Ctrl Pts',(-4.3119055044145,-23.4556222244942,9.54838337838673));
#4132=CARTESIAN_POINT('Ctrl Pts',(-2.91241403581534,-22.2626701765213,9.6629667117203));
#4133=CARTESIAN_POINT('Ctrl Pts',(-2.06264233798167,-21.8407362867315,9.72025837838672));
#4134=CARTESIAN_POINT('Ctrl Pts',(-0.259273913597949,-21.4470148995327,
9.83484171172031));
#4135=CARTESIAN_POINT('Ctrl Pts',(0.692608135318521,-21.4756565369004,9.89213337838646));
#4136=CARTESIAN_POINT('Ctrl Pts',(2.47524483330821,-21.9805320092516,10.0067167117206));
#4137=CARTESIAN_POINT('Ctrl Pts',(3.30427865677026,-22.456334096069,10.0640083783868));
#4138=CARTESIAN_POINT('Ctrl Pts',(4.64331059261914,-23.746807008819,10.1785917117202));
#4139=CARTESIAN_POINT('Ctrl Pts',(5.15198992536476,-24.5602812036706,10.2358833783863));
#4140=CARTESIAN_POINT('Ctrl Pts',(5.72659068860977,-26.3362007514714,10.3504667117207));
#4141=CARTESIAN_POINT('Ctrl Pts',(5.79191122945707,-27.2969627794171,10.4077583783851));
#4142=CARTESIAN_POINT('Ctrl Pts',(5.46015386112188,-29.1408223535089,10.5223417117219));
#4143=CARTESIAN_POINT('Ctrl Pts',(5.0633408173762,-30.0221456023925,10.5796333783862));
#4144=CARTESIAN_POINT('Ctrl Pts',(3.89718634706722,-31.4972337435744,10.6942167117208));
#4145=CARTESIAN_POINT('Ctrl Pts',(3.12891910014267,-32.0895535950602,10.7515083783862));
#4146=CARTESIAN_POINT('Ctrl Pts',(1.39873050144544,-32.8433866453836,10.8660917117208));
#4147=CARTESIAN_POINT('Ctrl Pts',(0.438443782857998,-33.004129268492,10.9233833783868));
#4148=CARTESIAN_POINT('Ctrl Pts',(-1.44967365457374,-32.8526684861381,11.0379667117202));
#4149=CARTESIAN_POINT('Ctrl Pts',(-2.37569293390397,-32.5405567018643,11.095258378387));
#4150=CARTESIAN_POINT('Ctrl Pts',(-3.97520797506477,-31.5130909749686,11.2098417117201));
#4151=CARTESIAN_POINT('Ctrl Pts',(-4.64714388655123,-30.7986754121516,11.2671333783872));
#4152=CARTESIAN_POINT('Ctrl Pts',(-5.57670175301804,-29.1324347002942,11.3817167117199));
#4153=CARTESIAN_POINT('Ctrl Pts',(-5.83338727717491,-28.1821782771171,11.4390083783853));
#4154=CARTESIAN_POINT('Ctrl Pts',(-5.85055548489977,-27.224883365232,11.4963000450535));
#4155=CARTESIAN_POINT('Ctrl Pts',(-3.5,-27.2127225901214,0.49751661203513));
#4156=CARTESIAN_POINT('Ctrl Pts',(-3.51517840571961,-26.6400364200585,0.554808278701816));
#4157=CARTESIAN_POINT('Ctrl Pts',(-3.3870023381626,-26.0622733505102,0.612099945368435));
#4158=CARTESIAN_POINT('Ctrl Pts',(-2.87059435406378,-25.0317443834292,0.726683278701825));
#4159=CARTESIAN_POINT('Ctrl Pts',(-2.48280922845853,-24.5799895371609,0.78397494536851));
#4160=CARTESIAN_POINT('Ctrl Pts',(-1.5358478118566,-23.9107403226621,0.89855827870175));
#4161=CARTESIAN_POINT('Ctrl Pts',(-0.9775476488716,-23.6939306641498,0.955849945368433));
#4162=CARTESIAN_POINT('Ctrl Pts',(0.179952537651027,-23.5494231527329,1.07043327870183));
#4163=CARTESIAN_POINT('Ctrl Pts',(0.778050540497913,-23.6219168035854,1.12772494536847));
#4164=CARTESIAN_POINT('Ctrl Pts',(1.8733753753257,-24.0427572309574,1.24230827870179));
#4165=CARTESIAN_POINT('Ctrl Pts',(2.36953393381726,-24.3907508815125,1.29959994536854));
#4166=CARTESIAN_POINT('Ctrl Pts',(3.14152259901176,-25.2835700713775,1.41418327870172));
#4167=CARTESIAN_POINT('Ctrl Pts',(3.41657284380058,-25.8275754937386,1.47147494536833));
#4168=CARTESIAN_POINT('Ctrl Pts',(3.67788133105185,-26.9856580964836,1.58605827870193));
#4169=CARTESIAN_POINT('Ctrl Pts',(3.6638371082595,-27.5986378942041,1.64334994536846));
#4170=CARTESIAN_POINT('Ctrl Pts',(3.34636951441486,-28.7497642955404,1.7579332787018));
#4171=CARTESIAN_POINT('Ctrl Pts',(3.04319861323196,-29.2867941907393,1.81522494536844));
#4172=CARTESIAN_POINT('Ctrl Pts',(2.21569658675549,-30.1572272297066,1.92980827870182));
#4173=CARTESIAN_POINT('Ctrl Pts',(1.69211920432461,-30.4897598664222,1.98709994536844));
#4174=CARTESIAN_POINT('Ctrl Pts',(0.545399516782365,-30.8693362630914,2.10168327870182));
#4175=CARTESIAN_POINT('Ctrl Pts',(-0.0766613701186401,-30.9159656984605,
2.15897494536837));
#4176=CARTESIAN_POINT('Ctrl Pts',(-1.27368235791308,-30.7088149551059,2.27355827870189));
#4177=CARTESIAN_POINT('Ctrl Pts',(-1.84748694212142,-30.4551804406305,2.33084994536843));
#4178=CARTESIAN_POINT('Ctrl Pts',(-2.81085353585185,-29.7038368014157,2.44543327870183));
#4179=CARTESIAN_POINT('Ctrl Pts',(-3.19946002926004,-29.2068050390794,2.50272494536839));
#4180=CARTESIAN_POINT('Ctrl Pts',(-3.69753543763233,-28.0836708006555,2.61730827870187));
#4181=CARTESIAN_POINT('Ctrl Pts',(-3.80647844076847,-27.458622235808,2.67459994536846));
#4182=CARTESIAN_POINT('Ctrl Pts',(-3.71562299996974,-26.2264422651536,2.7891832787018));
#4183=CARTESIAN_POINT('Ctrl Pts',(-3.51585820108909,-25.6204948140464,2.84647494536852));
#4184=CARTESIAN_POINT('Ctrl Pts',(-2.85104839504354,-24.5708958126827,2.96105827870174));
#4185=CARTESIAN_POINT('Ctrl Pts',(-2.38659484300895,-24.1282780503191,3.01834994536843));
#4186=CARTESIAN_POINT('Ctrl Pts',(-1.29941672607197,-23.5127480152682,3.13293327870183));
#4187=CARTESIAN_POINT('Ctrl Pts',(-0.677706928819807,-23.3404717664636,
3.19022494536847));
#4188=CARTESIAN_POINT('Ctrl Pts',(0.578163556381843,-23.3101149563751,3.30480827870179));
#4189=CARTESIAN_POINT('Ctrl Pts',(1.2111228729238,-23.4521169599317,3.3620999453685));
#4190=CARTESIAN_POINT('Ctrl Pts',(2.33910252832393,-24.02061342208,3.47668327870176));
#4191=CARTESIAN_POINT('Ctrl Pts',(2.83301860484105,-24.4466112594378,3.53397494536822));
#4192=CARTESIAN_POINT('Ctrl Pts',(3.56365731501942,-25.4854485489357,3.64855827870204));
#4193=CARTESIAN_POINT('Ctrl Pts',(3.79963651139122,-26.0973239813465,3.70584994536859));
#4194=CARTESIAN_POINT('Ctrl Pts',(3.95497473778028,-27.364790261788,3.82043327870167));
#4195=CARTESIAN_POINT('Ctrl Pts',(3.87413190281369,-28.0191738915788,3.87772494536818));
#4196=CARTESIAN_POINT('Ctrl Pts',(3.41100565544429,-29.2165857266924,3.99230827870208));
#4197=CARTESIAN_POINT('Ctrl Pts',(3.02911582100773,-29.7584479983173,4.04959994536851));
#4198=CARTESIAN_POINT('Ctrl Pts',(2.05088038850359,-30.6005359623087,4.16418327870175));
#4199=CARTESIAN_POINT('Ctrl Pts',(1.45543661955604,-30.8999147331016,4.22147494536847));
#4200=CARTESIAN_POINT('Ctrl Pts',(0.188979035414647,-31.1827803445244,4.33605827870178));
#4201=CARTESIAN_POINT('Ctrl Pts',(-0.480833721736332,-31.1659440974169,
4.39334994536825));
#4202=CARTESIAN_POINT('Ctrl Pts',(-1.73770028168812,-30.8164005771944,4.50793327870201));
#4203=CARTESIAN_POINT('Ctrl Pts',(-2.32353622117369,-30.4839764587754,4.56522494536848));
#4204=CARTESIAN_POINT('Ctrl Pts',(-3.27210326748465,-29.5783404250336,4.67980827870178));
#4205=CARTESIAN_POINT('Ctrl Pts',(-3.63388912134312,-29.0059569982611,4.73709994536835));
#4206=CARTESIAN_POINT('Ctrl Pts',(-4.04554144449821,-27.7534971521348,4.85168327870191));
#4207=CARTESIAN_POINT('Ctrl Pts',(-4.09496290407286,-27.0746033058008,4.90897494536821));
#4208=CARTESIAN_POINT('Ctrl Pts',(-3.86625503665767,-25.7692073365837,5.02355827870204));
#4209=CARTESIAN_POINT('Ctrl Pts',(-3.58829199607698,-25.1439644058301,5.08084994536843));
#4210=CARTESIAN_POINT('Ctrl Pts',(-2.76684905815666,-24.0951815694044,5.19543327870183));
#4211=CARTESIAN_POINT('Ctrl Pts',(-2.22411358260874,-23.6726788921877,5.25272494536842));
#4212=CARTESIAN_POINT('Ctrl Pts',(-0.998892343964084,-23.1323176637283,
5.36730827870184));
#4213=CARTESIAN_POINT('Ctrl Pts',(-0.317558152137087,-23.0150254765812,
5.42459994536842));
#4214=CARTESIAN_POINT('Ctrl Pts',(1.02458791243016,-23.1167116322358,5.53918327870184));
#4215=CARTESIAN_POINT('Ctrl Pts',(1.68411063294507,-23.3356459690878,5.59647494536849));
#4216=CARTESIAN_POINT('Ctrl Pts',(2.82558550724685,-24.0618452707057,5.71105827870177));
#4217=CARTESIAN_POINT('Ctrl Pts',(3.30641598130079,-24.5684600530816,5.76834994536854));
#4218=CARTESIAN_POINT('Ctrl Pts',(3.97403449448334,-25.75308885826,5.88293327870172));
#4219=CARTESIAN_POINT('Ctrl Pts',(4.16013667989657,-26.4299948886844,5.94022494536852));
#4220=CARTESIAN_POINT('Ctrl Pts',(4.19049349003537,-27.7963635466824,6.05480827870174));
#4221=CARTESIAN_POINT('Ctrl Pts',(4.03466554977154,-28.4845190963707,6.11209994536826));
#4222=CARTESIAN_POINT('Ctrl Pts',(3.41408060958811,-29.7099494400641,6.226683278702));
#4223=CARTESIAN_POINT('Ctrl Pts',(2.94987006045165,-30.2460267468577,6.28397494536819));
#4224=CARTESIAN_POINT('Ctrl Pts',(1.81915689809562,-31.0380549526863,6.39855827870207));
#4225=CARTESIAN_POINT('Ctrl Pts',(1.15370619622606,-31.2932036869398,6.45584994536854));
#4226=CARTESIAN_POINT('Ctrl Pts',(-0.223726178106239,-31.4593726282858,
6.57043327870172));
#4227=CARTESIAN_POINT('Ctrl Pts',(-0.934395434881124,-31.3701806092125,
6.62772494536832));
#4228=CARTESIAN_POINT('Ctrl Pts',(-2.2338942702282,-30.8647685418463,6.74230827870194));
#4229=CARTESIAN_POINT('Ctrl Pts',(-2.82146025502993,-30.4489825235109,6.79959994536845));
#4230=CARTESIAN_POINT('Ctrl Pts',(-3.73364751778378,-29.3853308484018,6.91418327870181));
#4231=CARTESIAN_POINT('Ctrl Pts',(-4.05735481460304,-28.7384487328433,6.97147494536818));
#4232=CARTESIAN_POINT('Ctrl Pts',(-4.36177755018722,-27.3636161673202,7.08605827870208));
#4233=CARTESIAN_POINT('Ctrl Pts',(-4.34214927877062,-26.6369704507106,7.14334994536865));
#4234=CARTESIAN_POINT('Ctrl Pts',(-3.96052983216839,-25.2743637321851,7.25793327870161));
#4235=CARTESIAN_POINT('Ctrl Pts',(-3.59885249650756,-24.6397217483839,7.31522494536868));
#4236=CARTESIAN_POINT('Ctrl Pts',(-2.61508245551368,-23.6130206947453,7.42980827870158));
#4237=CARTESIAN_POINT('Ctrl Pts',(-1.99389298437356,-23.2219816237259,7.48709994536824));
#4238=CARTESIAN_POINT('Ctrl Pts',(-0.635692979701946,-22.778253374105,7.60168327870201));
#4239=CARTESIAN_POINT('Ctrl Pts',(0.10003382610432,-22.7260398903107,7.65897494536861));
#4240=CARTESIAN_POINT('Ctrl Pts',(1.51380477670442,-22.9763048817946,7.77355827870165));
#4241=CARTESIAN_POINT('Ctrl Pts',(2.19048605403487,-23.2785964484885,7.83084994536837));
#4242=CARTESIAN_POINT('Ctrl Pts',(3.32468513313227,-24.1701386850904,7.94543327870189));
#4243=CARTESIAN_POINT('Ctrl Pts',(3.78108399417411,-24.758577873874,8.00272494536833));
#4244=CARTESIAN_POINT('Ctrl Pts',(4.36373104271076,-26.0858861127153,8.11730827870193));
#4245=CARTESIAN_POINT('Ctrl Pts',(4.48937241387869,-26.8235059315532,8.17459994536905));
#4246=CARTESIAN_POINT('Ctrl Pts',(4.37685554335844,-28.2756180899945,8.28918327870121));
#4247=CARTESIAN_POINT('Ctrl Pts',(4.13875166853063,-28.9887160799575,8.34647494536867));
#4248=CARTESIAN_POINT('Ctrl Pts',(3.35116287135924,-30.2220668271555,8.46105827870158));
#4249=CARTESIAN_POINT('Ctrl Pts',(2.80238685862471,-30.741110012937,8.51834994536944));
#4250=CARTESIAN_POINT('Ctrl Pts',(1.52030736522058,-31.4608170042187,8.63293327870083));
#4251=CARTESIAN_POINT('Ctrl Pts',(0.788205101607952,-31.6607451262615,8.69022494536734));
#4252=CARTESIAN_POINT('Ctrl Pts',(-0.688661729170329,-31.6911019364411,
8.80480827870292));
#4253=CARTESIAN_POINT('Ctrl Pts',(-1.43201351203358,-31.521448059472,8.86209994536876));
#4254=CARTESIAN_POINT('Ctrl Pts',(-2.75489454397912,-30.848774641259,8.9766832787015));
#4255=CARTESIAN_POINT('Ctrl Pts',(-3.33313308108255,-30.3463513803362,9.03397494536822));
#4256=CARTESIAN_POINT('Ctrl Pts',(-4.18655078253556,-29.1237623451318,9.14855827870204));
#4257=CARTESIAN_POINT('Ctrl Pts',(-4.46086905468824,-28.404736373781,9.20584994536822));
#4258=CARTESIAN_POINT('Ctrl Pts',(-4.63786871098225,-26.9173379055931,9.32043327870204));
#4259=CARTESIAN_POINT('Ctrl Pts',(-4.54032750779717,-26.1503830218042,9.3777249453685));
#4260=CARTESIAN_POINT('Ctrl Pts',(-3.99262962045306,-24.7487971862483,9.49230827870176));
#4261=CARTESIAN_POINT('Ctrl Pts',(-3.54294741821142,-24.1155274882508,9.54959994536835));
#4262=CARTESIAN_POINT('Ctrl Pts',(-2.39387950049328,-23.1332409267478,9.66418327870191));
#4263=CARTESIAN_POINT('Ctrl Pts',(-1.69555903830893,-22.7852051038846,9.72147494536834));
#4264=CARTESIAN_POINT('Ctrl Pts',(-0.212351491438122,-22.4592252441609,
9.83605827870193));
#4265=CARTESIAN_POINT('Ctrl Pts',(0.571127184652916,-22.4816455398733,9.89334994536808));
#4266=CARTESIAN_POINT('Ctrl Pts',(2.03947406174072,-22.8953409128601,10.0079332787022));
#4267=CARTESIAN_POINT('Ctrl Pts',(2.72292208988536,-23.2862714657652,10.0652249453684));
#4268=CARTESIAN_POINT('Ctrl Pts',(3.82775715080726,-24.3481755140014,10.1798082787018));
#4269=CARTESIAN_POINT('Ctrl Pts',(4.24804943901783,-25.0181710295281,10.2370999453679));
#4270=CARTESIAN_POINT('Ctrl Pts',(4.72385361508833,-26.4821111927169,10.3516832787023));
#4271=CARTESIAN_POINT('Ctrl Pts',(4.7788591231067,-27.2746709580248,10.4089749453667));
#4272=CARTESIAN_POINT('Ctrl Pts',(4.50703700756152,-28.7968168899771,10.5235582787035));
#4273=CARTESIAN_POINT('Ctrl Pts',(4.18041691475187,-29.5249365139219,10.5808499453678));
#4274=CARTESIAN_POINT('Ctrl Pts',(3.21877537946603,-30.7445518356469,10.6954332787024));
#4275=CARTESIAN_POINT('Ctrl Pts',(2.58463247743365,-31.2348468805496,10.7527249453679));
#4276=CARTESIAN_POINT('Ctrl Pts',(1.15523723842422,-31.8597797491362,10.8673082787024));
#4277=CARTESIAN_POINT('Ctrl Pts',(0.361331792548347,-31.9937703043426,10.9245999453685));
#4278=CARTESIAN_POINT('Ctrl Pts',(-1.20074645974137,-31.8704227189487,11.0391832787018));
#4279=CARTESIAN_POINT('Ctrl Pts',(-1.96741971917488,-31.6131493061509,11.0964749453686));
#4280=CARTESIAN_POINT('Ctrl Pts',(-3.29264633924976,-30.7641710134222,11.2110582787017));
#4281=CARTESIAN_POINT('Ctrl Pts',(-3.84990223677302,-30.1732337703105,11.2683499453688));
#4282=CARTESIAN_POINT('Ctrl Pts',(-4.62169770614474,-28.7937035887216,11.3829332787015));
#4283=CARTESIAN_POINT('Ctrl Pts',(-4.83545176440121,-28.0064051033624,11.440224945367));
#4284=CARTESIAN_POINT('Ctrl Pts',(-4.85063016993195,-27.212722590121,11.4975166120351));
#4285=CARTESIAN_POINT('Ctrl Pts',(-2.50007867078019,-27.2005618634838,0.498733174167452));
#4286=CARTESIAN_POINT('Ctrl Pts',(-2.51326728222517,-26.7914874409635,0.556024840834138));
#4287=CARTESIAN_POINT('Ctrl Pts',(-2.42404672820137,-26.3776775405011,0.613316507500758));
#4288=CARTESIAN_POINT('Ctrl Pts',(-2.05838114448734,-25.6376098899689,0.727899840834147));
#4289=CARTESIAN_POINT('Ctrl Pts',(-1.78223870534463,-25.3120853314176,0.785191507500833));
#4290=CARTESIAN_POINT('Ctrl Pts',(-1.10514273389326,-24.8279406528208,0.899774840834072));
#4291=CARTESIAN_POINT('Ctrl Pts',(-0.704807175805364,-24.6698281711569,
0.957066507500755));
#4292=CARTESIAN_POINT('Ctrl Pts',(0.1274352619041,-24.5613545958537,1.07164984083415));
#4293=CARTESIAN_POINT('Ctrl Pts',(0.558551263074086,-24.6111505358464,1.1289415075008));
#4294=CARTESIAN_POINT('Ctrl Pts',(1.35003809290966,-24.9104446162912,1.24352484083411));
#4295=CARTESIAN_POINT('Ctrl Pts',(1.70963130021051,-25.1597059023008,1.30081650750086));
#4296=CARTESIAN_POINT('Ctrl Pts',(2.27095531918287,-25.8021025401101,1.41539984083405));
#4297=CARTESIAN_POINT('Ctrl Pts',(2.4721077912595,-26.1946573298044,1.47269150750065));
#4298=CARTESIAN_POINT('Ctrl Pts',(2.66567502122425,-27.0325803320048,1.58727484083426));
#4299=CARTESIAN_POINT('Ctrl Pts',(2.65785211531719,-27.4771574273834,1.64456650750079));
#4300=CARTESIAN_POINT('Ctrl Pts',(2.43156425716401,-28.313995261359,1.75914984083412));
#4301=CARTESIAN_POINT('Ctrl Pts',(2.21326455198061,-28.7054399408851,1.81644150750076));
#4302=CARTESIAN_POINT('Ctrl Pts',(1.61433047837882,-29.3416770390113,1.93102484083414));
#4303=CARTESIAN_POINT('Ctrl Pts',(1.23423120401018,-29.5858229831059,1.98831650750076));
#4304=CARTESIAN_POINT('Ctrl Pts',(0.399489656769248,-29.8666031866432,2.10289984083414));
#4305=CARTESIAN_POINT('Ctrl Pts',(-0.0543696372039125,-29.902917630254,
2.16019150750069));
#4306=CARTESIAN_POINT('Ctrl Pts',(-0.929678265981594,-29.7557019006409,
2.27477484083421));
#4307=CARTESIAN_POINT('Ctrl Pts',(-1.3502798352523,-29.5722600576195,2.33206650750076));
#4308=CARTESIAN_POINT('Ctrl Pts',(-2.05817462844563,-29.0254285377532,2.44664984083415));
#4309=CARTESIAN_POINT('Ctrl Pts',(-2.344756721503,-28.6625205862691,2.50394150750071));
#4310=CARTESIAN_POINT('Ctrl Pts',(-2.71393246223352,-27.8401785078621,2.61852484083419));
#4311=CARTESIAN_POINT('Ctrl Pts',(-2.79612350398746,-27.3815105532419,2.67581650750078));
#4312=CARTESIAN_POINT('Ctrl Pts',(-2.73338114802542,-26.4753684673789,2.79039984083413));
#4313=CARTESIAN_POINT('Ctrl Pts',(-2.58845450226437,-26.0287664016884,2.84769150750084));
#4314=CARTESIAN_POINT('Ctrl Pts',(-2.10213141852588,-25.2534547274672,2.96227484083406));
#4315=CARTESIAN_POINT('Ctrl Pts',(-1.76115569452495,-24.9255165224303,3.01956650750075));
#4316=CARTESIAN_POINT('Ctrl Pts',(-0.960686964378836,-24.467748255277,3.13414984083416));
#4317=CARTESIAN_POINT('Ctrl Pts',(-0.501934458430937,-24.3384033014538,
3.19144150750079));
#4318=CARTESIAN_POINT('Ctrl Pts',(0.426712539268184,-24.3120260798245,3.30602484083412));
#4319=CARTESIAN_POINT('Ctrl Pts',(0.895718683084721,-24.4150725699735,3.36331650750083));
#4320=CARTESIAN_POINT('Ctrl Pts',(1.73323702163241,-24.8328266315758,3.47789984083408));
#4321=CARTESIAN_POINT('Ctrl Pts',(2.10092281068118,-25.1471817826938,3.53519150750045));
#4322=CARTESIAN_POINT('Ctrl Pts',(2.64645698476389,-25.9161536267569,3.64977484083445));
#4323=CARTESIAN_POINT('Ctrl Pts',(2.82373900440322,-26.3700644545806,3.707066507501));
#4324=CARTESIAN_POINT('Ctrl Pts',(2.94304329464034,-27.3122729858732,3.82164984083391));
#4325=CARTESIAN_POINT('Ctrl Pts',(2.8848981704904,-27.7996746143093,3.8789415075005));
#4326=CARTESIAN_POINT('Ctrl Pts',(2.54331827017279,-28.6932484441219,3.9935248408344));
#4327=CARTESIAN_POINT('Ctrl Pts',(2.26016080009324,-29.098545364816,4.05081650750084));
#4328=CARTESIAN_POINT('Ctrl Pts',(1.53234791989732,-29.7299686823744,4.16539984083407));
#4329=CARTESIAN_POINT('Ctrl Pts',(1.08835478333162,-29.9554496805941,4.2226915075008));
#4330=CARTESIAN_POINT('Ctrl Pts',(0.142056800052153,-30.1705740346633,4.33727484083411));
#4331=CARTESIAN_POINT('Ctrl Pts',(-0.359353255069153,-30.1599591044282,
4.39456650750057));
#4332=CARTESIAN_POINT('Ctrl Pts',(-1.30193124735312,-29.90159531999,4.50914984083433));
#4333=CARTESIAN_POINT('Ctrl Pts',(-1.74218197143407,-29.6540423974143,4.5664415075008));
#4334=CARTESIAN_POINT('Ctrl Pts',(-2.45655307667468,-28.9769743167667,4.6810248408341));
#4335=CARTESIAN_POINT('Ctrl Pts',(-2.72995223807354,-28.5480689977977,4.73831650750067));
#4336=CARTESIAN_POINT('Ctrl Pts',(-3.04280836800334,-27.6075872922707,4.85289984083423));
#4337=CARTESIAN_POINT('Ctrl Pts',(-3.08191483583748,-27.0968950385639,4.91019150750054));
#4338=CARTESIAN_POINT('Ctrl Pts',(-2.91314198222165,-26.1132114286668,5.02477484083437));
#4339=CARTESIAN_POINT('Ctrl Pts',(-2.70537161297122,-25.6411715125808,5.08206650750075));
#4340=CARTESIAN_POINT('Ctrl Pts',(-2.088440794589,-24.847860476929,5.19664984083415));
#4341=CARTESIAN_POINT('Ctrl Pts',(-1.67982912966058,-24.527382199886,5.25394150750074));
#4342=CARTESIAN_POINT('Ctrl Pts',(-0.755400051308564,-24.1159206391859,
5.36852484083416));
#4343=CARTESIAN_POINT('Ctrl Pts',(-0.240446469424114,-24.025380413375,5.42581650750074));
#4344=CARTESIAN_POINT('Ctrl Pts',(0.7756617100578,-24.0989534841673,5.54039984083416));
#4345=CARTESIAN_POINT('Ctrl Pts',(1.27583904542581,-24.2630496679924,5.59769150750081));
#4346=CARTESIAN_POINT('Ctrl Pts',(2.14302659233962,-24.8107622471434,5.71227484083409));
#4347=CARTESIAN_POINT('Ctrl Pts',(2.50917750925817,-25.1938992016932,5.76956650750086));
#4348=CARTESIAN_POINT('Ctrl Pts',(3.01903425440591,-26.0918186198254,5.88414984083404));
#4349=CARTESIAN_POINT('Ctrl Pts',(3.16220514490754,-26.6057673592151,5.94144150750084));
#4350=CARTESIAN_POINT('Ctrl Pts',(3.18858236658479,-27.644912529427,6.05602484083406));
#4351=CARTESIAN_POINT('Ctrl Pts',(3.07170993966424,-28.1691149066568,6.11331650750058));
#4352=CARTESIAN_POINT('Ctrl Pts',(2.60186740015778,-29.1040839332475,6.22789984083432));
#4353=CARTESIAN_POINT('Ctrl Pts',(2.2492995370817,-29.5139309527772,6.28519150750051));
#4354=CARTESIAN_POINT('Ctrl Pts',(1.38845182038838,-30.1208546223513,6.39977484083439));
#4355=CARTESIAN_POINT('Ctrl Pts',(0.880965722855629,-30.3173061799665,6.45706650750086));
#4356=CARTESIAN_POINT('Ctrl Pts',(-0.171208902055053,-30.4474411851313,
6.57164984083404));
#4357=CARTESIAN_POINT('Ctrl Pts',(-0.714896157737991,-30.3809468768386,
6.62894150750064));
#4358=CARTESIAN_POINT('Ctrl Pts',(-1.71055698753139,-29.9970811566254,6.74352484083427));
#4359=CARTESIAN_POINT('Ctrl Pts',(-2.16155762161384,-29.680027502494,6.80081650750078));
#4360=CARTESIAN_POINT('Ctrl Pts',(-2.86308023776419,-28.8667983798979,6.91539984083413));
#4361=CARTESIAN_POINT('Ctrl Pts',(-3.11288976212293,-28.3713668964897,6.97269150750051));
#4362=CARTESIAN_POINT('Ctrl Pts',(-3.34957124029864,-27.316693932087,7.0872748408344));
#4363=CARTESIAN_POINT('Ctrl Pts',(-3.33616428574757,-26.7584509172524,7.14456650750097));
#4364=CARTESIAN_POINT('Ctrl Pts',(-3.0457245749983,-25.7101327666455,7.25914984083393));
#4365=CARTESIAN_POINT('Ctrl Pts',(-2.76891843505522,-25.2210759980313,7.316441507501));
#4366=CARTESIAN_POINT('Ctrl Pts',(-2.01371634733806,-24.4285708856475,7.4310248408339));
#4367=CARTESIAN_POINT('Ctrl Pts',(-1.53600498378822,-24.1259185069575,7.48831650750057));
#4368=CARTESIAN_POINT('Ctrl Pts',(-0.48978311995981,-23.7809864506379,7.60289984083434));
#4369=CARTESIAN_POINT('Ctrl Pts',(0.0777420934653123,-23.7390879585698,
7.66019150750093));
#4370=CARTESIAN_POINT('Ctrl Pts',(1.16980068449715,-23.9294179362069,7.77477484083397));
#4371=CARTESIAN_POINT('Ctrl Pts',(1.69327894738216,-24.1615168316733,7.83206650750108));
#4372=CARTESIAN_POINT('Ctrl Pts',(2.57200622550959,-24.848546948579,7.94664984083383));
#4373=CARTESIAN_POINT('Ctrl Pts',(2.92638068652453,-25.3028623269368,8.00394150750066));
#4374=CARTESIAN_POINT('Ctrl Pts',(3.38012806720446,-26.3293784052561,8.11852484083425));
#4375=CARTESIAN_POINT('Ctrl Pts',(3.47901747707488,-26.9006176143865,8.17581650750176));
#4376=CARTESIAN_POINT('Ctrl Pts',(3.39461369143692,-28.0266918875018,8.29039984083314));
#4377=CARTESIAN_POINT('Ctrl Pts',(3.2113479695612,-28.5804444925376,8.347691507501));
#4378=CARTESIAN_POINT('Ctrl Pts',(2.60224589498633,-29.5395079121489,8.4622748408339));
#4379=CARTESIAN_POINT('Ctrl Pts',(2.17694770990781,-29.943871540951,8.51956650750176));
#4380=CARTESIAN_POINT('Ctrl Pts',(1.1815776037604,-30.5058167640846,8.63414984083314));
#4381=CARTESIAN_POINT('Ctrl Pts',(0.612432630957585,-30.6628135912745,8.69144150749966));
#4382=CARTESIAN_POINT('Ctrl Pts',(-0.537210711795104,-30.6891908129884,
8.80602484083524));
#4383=CARTESIAN_POINT('Ctrl Pts',(-1.11660932242181,-30.5584924493121,8.86331650750108));
#4384=CARTESIAN_POINT('Ctrl Pts',(-2.14902903706022,-30.0365614318812,8.97789984083382));
#4385=CARTESIAN_POINT('Ctrl Pts',(-2.60103728706707,-29.6457808568702,9.03519150750054));
#4386=CARTESIAN_POINT('Ctrl Pts',(-3.26935045213561,-28.6930572675207,9.14977484083436));
#4387=CARTESIAN_POINT('Ctrl Pts',(-3.48497154772812,-28.1319959002986,9.20706650750054));
#4388=CARTESIAN_POINT('Ctrl Pts',(-3.62593726781443,-26.9698551817563,9.32164984083436));
#4389=CARTESIAN_POINT('Ctrl Pts',(-3.55109377538202,-26.3698822988422,9.37894150750082));
#4390=CARTESIAN_POINT('Ctrl Pts',(-3.12494223527345,-25.2721344690503,9.49352484083408));
#4391=CARTESIAN_POINT('Ctrl Pts',(-2.77399239711041,-24.7754301215948,9.55081650750067));
#4392=CARTESIAN_POINT('Ctrl Pts',(-1.87534703207357,-24.0038082068396,9.66539984083423));
#4393=CARTESIAN_POINT('Ctrl Pts',(-1.328477201847,-23.7296701563417,9.72269150750066));
#4394=CARTESIAN_POINT('Ctrl Pts',(-0.165429256313216,-23.4714315540725,
9.83727484083425));
#4395=CARTESIAN_POINT('Ctrl Pts',(0.449646718215928,-23.487630532928,9.8945665075004));
#4396=CARTESIAN_POINT('Ctrl Pts',(1.60370502717545,-23.8101461699985,10.0091498408345));
#4397=CARTESIAN_POINT('Ctrl Pts',(2.14156784031432,-24.1162055272932,10.0664415075007));
#4398=CARTESIAN_POINT('Ctrl Pts',(3.01220695982868,-24.9495416221013,10.1810248408342));
#4399=CARTESIAN_POINT('Ctrl Pts',(3.344112555819,-25.4760590302157,10.2383165075002));
#4400=CARTESIAN_POINT('Ctrl Pts',(3.7211205385227,-26.6280210523566,10.3528998408347));
#4401=CARTESIAN_POINT('Ctrl Pts',(3.76581105482833,-27.2523792254888,10.4101915074991));
#4402=CARTESIAN_POINT('Ctrl Pts',(3.55392395316851,-28.4528127976668,10.5247748408358));
#4403=CARTESIAN_POINT('Ctrl Pts',(3.29749653150255,-29.0277294073495,10.5820665075001));
#4404=CARTESIAN_POINT('Ctrl Pts',(2.54036711604196,-29.9918729279439,10.6966498408348));
#4405=CARTESIAN_POINT('Ctrl Pts',(2.040348024276,-30.3801435729391,10.7539415075002));
#4406=CARTESIAN_POINT('Ctrl Pts',(0.911744945978275,-30.8761767735908,10.8685248408347));
#4407=CARTESIAN_POINT('Ctrl Pts',(0.284220109610612,-30.9834153675301,10.9258165075008));
#4408=CARTESIAN_POINT('Ctrl Pts',(-0.951820257144186,-30.8881808670358,
11.0403998408341));
#4409=CARTESIAN_POINT('Ctrl Pts',(-1.55914813184147,-30.6857456071259,11.0976915075009));
#4410=CARTESIAN_POINT('Ctrl Pts',(-2.61008742415662,-30.015254037105,11.212274840834));
#4411=CARTESIAN_POINT('Ctrl Pts',(-3.05266376483645,-29.5477946215084,11.2695665075011));
#4412=CARTESIAN_POINT('Ctrl Pts',(-3.6666974659612,-28.4549738273466,11.3841498408338));
#4413=CARTESIAN_POINT('Ctrl Pts',(-3.83752022944408,-27.8306326302477,11.4414415074993));
#4414=CARTESIAN_POINT('Ctrl Pts',(-3.85070884071214,-27.2005618634835,11.4987331741675));
#4415=CARTESIAN_POINT('Ctrl Pts',(-2.50007468503749,-27.1010187070962,-0.496297400879471));
#4416=CARTESIAN_POINT('Ctrl Pts',(-2.49697558534321,-26.6919449367377,-0.439005734212785));
#4417=CARTESIAN_POINT('Ctrl Pts',(-2.39148306502197,-26.2822116441738,-0.381714067546166));
#4418=CARTESIAN_POINT('Ctrl Pts',(-1.99708913925533,-25.5575010913513,-0.267130734212776));
#4419=CARTESIAN_POINT('Ctrl Pts',(-1.70851780633352,-25.2432423319883,-0.209839067546131));
#4420=CARTESIAN_POINT('Ctrl Pts',(-1.01332498488648,-24.7861838511185,-0.0952557342128104));
#4421=CARTESIAN_POINT('Ctrl Pts',(-0.607338782057628,-24.6438658572855,
-0.0379640675461273));
#4422=CARTESIAN_POINT('Ctrl Pts',(0.22809530726186,-24.5678109717687,0.0766192657871858));
#4423=CARTESIAN_POINT('Ctrl Pts',(0.656749262161081,-24.6342001019302,0.133910932453873));
#4424=CARTESIAN_POINT('Ctrl Pts',(1.43576881284334,-24.9635894484093,0.248494265787185));
#4425=CARTESIAN_POINT('Ctrl Pts',(1.78536871348538,-25.226324021095,0.305785932453894));
#4426=CARTESIAN_POINT('Ctrl Pts',(2.32151076365989,-25.8893852792693,0.420369265787164));
#4427=CARTESIAN_POINT('Ctrl Pts',(2.50749866272339,-26.2891116348328,0.477660932453768));
#4428=CARTESIAN_POINT('Ctrl Pts',(2.6691161443131,-27.1333885072357,0.592244265787291));
#4429=CARTESIAN_POINT('Ctrl Pts',(2.64453862625626,-27.577141828817,0.649535932453863));
#4430=CARTESIAN_POINT('Ctrl Pts',(2.38707841193931,-28.4045222689121,0.764119265787196));
#4431=CARTESIAN_POINT('Ctrl Pts',(2.15439078230601,-28.7873423753173,0.821410932453838));
#4432=CARTESIAN_POINT('Ctrl Pts',(1.53242332955732,-29.4005442496924,0.93599426578722));
#4433=CARTESIAN_POINT('Ctrl Pts',(1.14370063429288,-29.6303015787241,0.993285932453714));
#4434=CARTESIAN_POINT('Ctrl Pts',(0.299504189499764,-29.8799086688388,1.10786926578734));
#4435=CARTESIAN_POINT('Ctrl Pts',(-0.155177536543765,-29.8994684343923,
1.16516093245394));
#4436=CARTESIAN_POINT('Ctrl Pts',(-1.02412973658168,-29.7203034653188,1.27974426578712));
#4437=CARTESIAN_POINT('Ctrl Pts',(-1.43755852562162,-29.5216976236493,1.33703593245383));
#4438=CARTESIAN_POINT('Ctrl Pts',(-2.1247866819161,-28.9496857898884,1.45161926578722));
#4439=CARTESIAN_POINT('Ctrl Pts',(-2.39789468808455,-28.576785610739,1.50891093245379));
#4440=CARTESIAN_POINT('Ctrl Pts',(-2.73697416446945,-27.7419786632607,1.62349426578727));
#4441=CARTESIAN_POINT('Ctrl Pts',(-2.80257181896535,-27.280849991177,1.68078593245385));
#4442=CARTESIAN_POINT('Ctrl Pts',(-2.70741102889003,-26.3779021530229,1.7953692657872));
#4443=CARTESIAN_POINT('Ctrl Pts',(-2.54669034787763,-25.9369519968831,1.85266093245392));
#4444=CARTESIAN_POINT('Ctrl Pts',(-2.03328251568525,-25.1797393416946,1.96724426578714));
#4445=CARTESIAN_POINT('Ctrl Pts',(-1.6810419878648,-24.8642309325484,2.02453593245391));
#4446=CARTESIAN_POINT('Ctrl Pts',(-0.86521846062969,-24.4351922371926,2.13911926578715));
#4447=CARTESIAN_POINT('Ctrl Pts',(-0.402390649877755,-24.322119576435,2.19641093245378));
#4448=CARTESIAN_POINT('Ctrl Pts',(0.526255043490125,-24.3283177763288,2.31099426578728));
#4449=CARTESIAN_POINT('Ctrl Pts',(0.991184579421847,-24.4476362331387,2.36828593245382));
#4450=CARTESIAN_POINT('Ctrl Pts',(1.81334582024015,-24.8941186368221,2.48286926578724));
#4451=CARTESIAN_POINT('Ctrl Pts',(2.16976581012525,-25.2209026816946,2.54016093245371));
#4452=CARTESIAN_POINT('Ctrl Pts',(2.68821378645142,-26.007971375774,2.65474426578735));
#4453=CARTESIAN_POINT('Ctrl Pts',(2.84970131829056,-26.4675328483271,2.71203593245399));
#4454=CARTESIAN_POINT('Ctrl Pts',(2.93658691870944,-27.4129330312322,2.82661926578707));
#4455=CARTESIAN_POINT('Ctrl Pts',(2.86184860442354,-27.897872613403,2.88391093245367));
#4456=CARTESIAN_POINT('Ctrl Pts',(2.49017343803774,-28.7789791640489,2.99849426578739));
#4457=CARTESIAN_POINT('Ctrl Pts',(2.19354268131092,-29.1742827781052,3.05578593245391));
#4458=CARTESIAN_POINT('Ctrl Pts',(1.44506518072621,-29.7805241268371,3.17036926578715));
#4459=CARTESIAN_POINT('Ctrl Pts',(0.993900478307379,-29.9908405520754,3.22766093245387));
#4460=CARTESIAN_POINT('Ctrl Pts',(0.0412486248171475,-30.1740151577347,
3.34224426578718));
#4461=CARTESIAN_POINT('Ctrl Pts',(-0.459337656509201,-30.1466456153845,
3.39953593245365));
#4462=CARTESIAN_POINT('Ctrl Pts',(-1.39245825489971,-29.8571094747481,3.51411926578741));
#4463=CARTESIAN_POINT('Ctrl Pts',(-1.82408440587509,-29.5951686277527,3.57141093245388));
#4464=CARTESIAN_POINT('Ctrl Pts',(-2.51542028734699,-28.8950671679322,3.68599426578718));
#4465=CARTESIAN_POINT('Ctrl Pts',(-2.77443083370738,-28.4575384280859,3.74328593245375));
#4466=CARTESIAN_POINT('Ctrl Pts',(-3.05611385018328,-27.5076018249958,3.85786926578731));
#4467=CARTESIAN_POINT('Ctrl Pts',(-3.07846563998978,-26.9960871392191,3.91516093245361));
#4468=CARTESIAN_POINT('Ctrl Pts',(-2.87774354688549,-26.0187599580717,4.02974426578744));
#4469=CARTESIAN_POINT('Ctrl Pts',(-2.65480917901121,-25.5538928222013,4.08703593245365));
#4470=CARTESIAN_POINT('Ctrl Pts',(-2.01269804671401,-24.7812484234687,4.20161926578741));
#4471=CARTESIAN_POINT('Ctrl Pts',(-1.59409415413557,-24.4742442332878,4.25891093245382));
#4472=CARTESIAN_POINT('Ctrl Pts',(-0.657200206702104,-24.0928789369666,
4.37349426578724));
#4473=CARTESIAN_POINT('Ctrl Pts',(-0.139785907354555,-24.0189320983815,
4.43078593245364));
#4474=CARTESIAN_POINT('Ctrl Pts',(0.873128024409321,-24.1249236033184,4.54536926578742));
#4475=CARTESIAN_POINT('Ctrl Pts',(1.36765345024244,-24.3048138223663,4.60266093245389));
#4476=CARTESIAN_POINT('Ctrl Pts',(2.21674197810085,-24.8796111499969,4.71724426578717));
#4477=CARTESIAN_POINT('Ctrl Pts',(2.57046309915192,-25.2740129083479,4.77453593245413));
#4478=CARTESIAN_POINT('Ctrl Pts',(3.05159027247857,-26.1872871235801,4.88911926578693));
#4479=CARTESIAN_POINT('Ctrl Pts',(3.1784888699414,-26.7053111677683,4.94641093245373));
#4480=CARTESIAN_POINT('Ctrl Pts',(3.17229067006551,-27.7444550336489,5.06099426578732));
#4481=CARTESIAN_POINT('Ctrl Pts',(3.03914627651117,-28.2645808029984,5.11828593245366));
#4482=CARTESIAN_POINT('Ctrl Pts',(2.54057539489944,-29.1841927318507,5.2328692657874));
#4483=CARTESIAN_POINT('Ctrl Pts',(2.17557863808745,-29.5827739522296,5.29016093245358));
#4484=CARTESIAN_POINT('Ctrl Pts',(1.29663407136474,-30.1626114240305,5.40474426578747));
#4485=CARTESIAN_POINT('Ctrl Pts',(0.783497329111631,-30.3432684938695,5.46203593245413));
#4486=CARTESIAN_POINT('Ctrl Pts',(-0.271868947416543,-30.4409848091847,
5.57661926578693));
#4487=CARTESIAN_POINT('Ctrl Pts',(-0.813094156837556,-30.3578973107856,
5.63391093245353));
#4488=CARTESIAN_POINT('Ctrl Pts',(-1.7962877074525,-29.9439363244765,5.74849426578753));
#4489=CARTESIAN_POINT('Ctrl Pts',(-2.23729503491243,-29.613409383722,5.80578593245404));
#4490=CARTESIAN_POINT('Ctrl Pts',(-2.91363568221747,-28.7795156407165,5.92036926578702));
#4491=CARTESIAN_POINT('Ctrl Pts',(-3.14828063361543,-28.2769125914658,5.97766093245358));
#4492=CARTESIAN_POINT('Ctrl Pts',(-3.35301236335888,-27.2158857568516,6.09224426578747));
#4493=CARTESIAN_POINT('Ctrl Pts',(-3.32285079671477,-26.6584665158089,6.14953593245386));
#4494=CARTESIAN_POINT('Ctrl Pts',(-3.00123872974546,-25.6196057591023,6.2641192657872));
#4495=CARTESIAN_POINT('Ctrl Pts',(-2.71004466540204,-25.1391735635767,6.32141093245427));
#4496=CARTESIAN_POINT('Ctrl Pts',(-1.93180919849512,-24.3697036749888,6.43599426578679));
#4497=CARTESIAN_POINT('Ctrl Pts',(-1.44547441408027,-24.0814399113125,6.49328593245345));
#4498=CARTESIAN_POINT('Ctrl Pts',(-0.389797652680968,-23.7676809684691,
6.60786926578761));
#4499=CARTESIAN_POINT('Ctrl Pts',(0.178549992812208,-23.7425371544047,6.66516093245401));
#4500=CARTESIAN_POINT('Ctrl Pts',(1.26425215509018,-23.9648163715558,6.77974426578705));
#4501=CARTESIAN_POINT('Ctrl Pts',(1.7805576377681,-24.2120792656227,6.83703593245416));
#4502=CARTESIAN_POINT('Ctrl Pts',(2.63861827896344,-24.9242896964646,6.9516192657869));
#4503=CARTESIAN_POINT('Ctrl Pts',(2.9795186531323,-25.3885973024572,7.00891093245373));
#4504=CARTESIAN_POINT('Ctrl Pts',(3.40316976941416,-26.4275782498672,7.12349426578732));
#4505=CARTESIAN_POINT('Ctrl Pts',(3.4854657920787,-27.0012781764557,7.18078593245407));
#4506=CARTESIAN_POINT('Ctrl Pts',(3.36864357227559,-28.1241582018537,7.29536926578699));
#4507=CARTESIAN_POINT('Ctrl Pts',(3.16958381519666,-28.6722588973589,7.35266093245407));
#4508=CARTESIAN_POINT('Ctrl Pts',(2.53339699212349,-29.6132232979053,7.46724426578698));
#4509=CARTESIAN_POINT('Ctrl Pts',(2.09683400325949,-30.0051571308579,7.52453593245425));
#4510=CARTESIAN_POINT('Ctrl Pts',(1.08610909999943,-30.538372782144,7.63911926578681));
#4511=CARTESIAN_POINT('Ctrl Pts',(0.512888822404401,-30.6790973163175,7.69641093245254));
#4512=CARTESIAN_POINT('Ctrl Pts',(-0.636753216017042,-30.67289911646,7.81099426578851));
#4513=CARTESIAN_POINT('Ctrl Pts',(-1.21207521877181,-30.5259287861701,7.86828593245416));
#4514=CARTESIAN_POINT('Ctrl Pts',(-2.22913783565509,-29.9752694266119,7.9828692657869));
#4515=CARTESIAN_POINT('Ctrl Pts',(-2.66988028653065,-29.5720599578842,8.04016093245362));
#4516=CARTESIAN_POINT('Ctrl Pts',(-3.31110725380362,-28.6012395184888,8.15474426578744));
#4517=CARTESIAN_POINT('Ctrl Pts',(-3.51093386164047,-28.034527506556,8.21203593245362));
#4518=CARTESIAN_POINT('Ctrl Pts',(-3.61948089185851,-26.8691951363934,8.32661926578744));
#4519=CARTESIAN_POINT('Ctrl Pts',(-3.52804420933835,-26.2716842997393,8.3839109324539));
#4520=CARTESIAN_POINT('Ctrl Pts',(-3.07179740311519,-25.1864037491325,8.49849426578716));
#4521=CARTESIAN_POINT('Ctrl Pts',(-2.70737427834283,-24.6996927082866,8.55578593245375));
#4522=CARTESIAN_POINT('Ctrl Pts',(-1.78806429288772,-23.9532527623958,8.67036926578731));
#4523=CARTESIAN_POINT('Ctrl Pts',(-1.2340228968259,-23.6942792848374,8.72766093245373));
#4524=CARTESIAN_POINT('Ctrl Pts',(-0.0646210810750642,-23.467990431024,
8.84224426578733));
#4525=CARTESIAN_POINT('Ctrl Pts',(0.549631119664167,-23.5009440219499,8.89953593245347));
#4526=CARTESIAN_POINT('Ctrl Pts',(1.69423203471385,-23.8546320152623,9.01411926578758));
#4527=CARTESIAN_POINT('Ctrl Pts',(2.22347027477345,-24.1750792969402,9.07141093245382));
#4528=CARTESIAN_POINT('Ctrl Pts',(3.07107417048285,-25.0314487709504,9.18599426578724));
#4529=CARTESIAN_POINT('Ctrl Pts',(3.38859115147477,-25.5665895999213,9.2432859324533));
#4530=CARTESIAN_POINT('Ctrl Pts',(3.73442602068069,-26.7280065196379,9.35786926578775));
#4531=CARTESIAN_POINT('Ctrl Pts',(3.76236185900407,-27.3531871248382,9.41516093245296));
#4532=CARTESIAN_POINT('Ctrl Pts',(3.5185255178089,-28.5472642682574,9.5297442657881));
#4533=CARTESIAN_POINT('Ctrl Pts',(3.24693409756131,-29.1150080977418,9.58703593245323));
#4534=CARTESIAN_POINT('Ctrl Pts',(2.46462436814819,-30.0584849813914,9.70161926578783));
#4535=CARTESIAN_POINT('Ctrl Pts',(1.95461304876198,-30.4332815395597,9.75891093245325));
#4536=CARTESIAN_POINT('Ctrl Pts',(0.813545101360808,-30.8992184757877,9.8734942657878));
#4537=CARTESIAN_POINT('Ctrl Pts',(0.183559547541048,-30.9898636825423,9.93078593245385));
#4538=CARTESIAN_POINT('Ctrl Pts',(-1.0492865714957,-30.8622107478662,10.0453692657872));
#4539=CARTESIAN_POINT('Ctrl Pts',(-1.65096253667027,-30.6439814527683,10.102660932454));
#4540=CARTESIAN_POINT('Ctrl Pts',(-2.68380280990567,-29.9464051342351,10.2172442657871));
#4541=CARTESIAN_POINT('Ctrl Pts',(-3.11394935474709,-29.4676809148667,10.2745359324542));
#4542=CARTESIAN_POINT('Ctrl Pts',(-3.69925348401698,-28.3595053235791,10.3891192657869));
#4543=CARTESIAN_POINT('Ctrl Pts',(-3.85380395473586,-27.7310888216945,10.4464109324524));
#4544=CARTESIAN_POINT('Ctrl Pts',(-3.85070485496943,-27.1010187070959,10.5037025991205));
#4545=CARTESIAN_POINT('Ctrl Pts',(-3.49999867141204,-27.1131792015256,-0.497516610416937));
#4546=CARTESIAN_POINT('Ctrl Pts',(-3.49888932799759,-26.5404932488512,-0.440224943750252));
#4547=CARTESIAN_POINT('Ctrl Pts',(-3.35444114738347,-25.9668063623456,-0.382933277083632));
#4548=CARTESIAN_POINT('Ctrl Pts',(-2.80930434430968,-24.9516337619221,-0.268349943750243));
#4549=CARTESIAN_POINT('Ctrl Pts',(-2.40908999522195,-24.5111444093371,-0.211058277083598));
#4550=CARTESIAN_POINT('Ctrl Pts',(-1.44403096339936,-23.8689809726516,-0.0964749437502769));
#4551=CARTESIAN_POINT('Ctrl Pts',(-0.880079720887058,-23.6679656879623,
-0.0391832770835939));
#4552=CARTESIAN_POINT('Ctrl Pts',(0.28061299005863,-23.5558768567235,0.0754000562497192));
#4553=CARTESIAN_POINT('Ctrl Pts',(0.876249383825206,-23.6449638021555,0.132691722916406));
#4554=CARTESIAN_POINT('Ctrl Pts',(1.95910771378206,-24.0958998985319,0.247275056249719));
#4555=CARTESIAN_POINT('Ctrl Pts',(2.44527330196474,-24.4573671339349,0.304566722916428));
#4556=CARTESIAN_POINT('Ctrl Pts',(3.19208049125558,-25.370851664545,0.419150056249697));
#4557=CARTESIAN_POINT('Ctrl Pts',(3.4519663191088,-25.9220290742938,0.476441722916301));
#4558=CARTESIAN_POINT('Ctrl Pts',(3.68132515309603,-27.08646641491,0.591025056249824));
#4559=CARTESIAN_POINT('Ctrl Pts',(3.65052625709869,-27.6986228841538,0.648316722916396));
#4560=CARTESIAN_POINT('Ctrl Pts',(3.30188598195419,-28.8402927016588,0.762900056249729));
#4561=CARTESIAN_POINT('Ctrl Pts',(2.98432689255302,-29.3686983876925,0.820191722916372));
#4562=CARTESIAN_POINT('Ctrl Pts',(2.13379081833063,-30.216096764043,0.934775056249753));
#4563=CARTESIAN_POINT('Ctrl Pts',(1.60158961081322,-30.5342409823362,0.992066722916289));
#4564=CARTESIAN_POINT('Ctrl Pts',(0.445414171550833,-30.8826444452813,1.10665005624984));
#4565=CARTESIAN_POINT('Ctrl Pts',(-0.177469596581333,-30.912519185481,1.16394172291647));
#4566=CARTESIAN_POINT('Ctrl Pts',(-1.36813499365341,-30.6734189584949,1.27852505624965));
#4567=CARTESIAN_POINT('Ctrl Pts',(-1.93476718568864,-30.4046202185468,1.33581672291637));
#4568=CARTESIAN_POINT('Ctrl Pts',(-2.87746776648538,-29.6280956550586,1.45040005624976));
#4569=CARTESIAN_POINT('Ctrl Pts',(-3.25260040831661,-29.1210712820873,1.50769172291632));
#4570=CARTESIAN_POINT('Ctrl Pts',(-3.72057981489945,-27.9854713421496,1.6222750562498));
#4571=CARTESIAN_POINT('Ctrl Pts',(-3.81292945777313,-27.3579616111638,1.67956672291639));
#4572=CARTESIAN_POINT('Ctrl Pts',(-3.68965542200644,-26.1289750303032,1.79415005624974));
#4573=CARTESIAN_POINT('Ctrl Pts',(-3.47409640017873,-25.5286790803258,1.85144172291645));
#4574=CARTESIAN_POINT('Ctrl Pts',(-2.78220129939746,-24.4971784172052,1.96602505624967));
#4575=CARTESIAN_POINT('Ctrl Pts',(-2.30648258548237,-24.0669901790178,2.02331672291636));
#4576=CARTESIAN_POINT('Ctrl Pts',(-1.20394886875872,-23.4801893728762,2.13790005624977));
#4577=CARTESIAN_POINT('Ctrl Pts',(-0.578163322834367,-23.3241853462944,
2.1951917229164));
#4578=CARTESIAN_POINT('Ctrl Pts',(0.677706727587892,-23.3264040337203,2.30977505624973));
#4579=CARTESIAN_POINT('Ctrl Pts',(1.30658986109621,-23.4846781506972,2.36706672291644));
#4580=CARTESIAN_POINT('Ctrl Pts',(2.4192131498232,-24.0819034318477,2.48165005624969));
#4581=CARTESIAN_POINT('Ctrl Pts',(2.9018637326796,-24.5203304926646,2.53894172291615));
#4582=CARTESIAN_POINT('Ctrl Pts',(3.60541666501523,-25.5772653974027,2.65352505624997));
#4583=CARTESIAN_POINT('Ctrl Pts',(3.82560148759511,-26.1947919093305,2.71081672291652));
#4584=CARTESIAN_POINT('Ctrl Pts',(3.94852103377322,-27.4654507141961,2.8254000562496));
#4585=CARTESIAN_POINT('Ctrl Pts',(3.85108490425945,-28.1173727349135,2.88269172291611));
#4586=CARTESIAN_POINT('Ctrl Pts',(3.35786298785392,-29.3023180651413,2.99727505625001));
#4587=CARTESIAN_POINT('Ctrl Pts',(2.96249956859728,-29.8341873664785,3.05456672291645));
#4588=CARTESIAN_POINT('Ctrl Pts',(1.96359879532417,-30.6510938545388,3.16915005624968));
#4589=CARTESIAN_POINT('Ctrl Pts',(1.36098303900346,-30.9353082084263,3.22644172291641));
#4590=CARTESIAN_POINT('Ctrl Pts',(0.0881707169855854,-31.1862241665521,
3.34102505624972));
#4591=CARTESIAN_POINT('Ctrl Pts',(-0.580818711692515,-31.1526332462716,
3.39831672291618));
#4592=CARTESIAN_POINT('Ctrl Pts',(-1.82822868779995,-30.7719170447183,3.51290005624994));
#4593=CARTESIAN_POINT('Ctrl Pts',(-2.40544041813704,-30.4251047381095,3.57019172291641));
#4594=CARTESIAN_POINT('Ctrl Pts',(-3.33097280181086,-29.4964346565957,3.68477505624972));
#4595=CARTESIAN_POINT('Ctrl Pts',(-3.67837023727213,-28.9154274047545,3.74206672291629));
#4596=CARTESIAN_POINT('Ctrl Pts',(-4.05884962667304,-27.6535118068985,3.85665005624984));
#4597=CARTESIAN_POINT('Ctrl Pts',(-4.09151639110769,-26.9737950793345,3.91394172291615));
#4598=CARTESIAN_POINT('Ctrl Pts',(-3.83085904003235,-25.6747547008469,4.02852505624998));
#4599=CARTESIAN_POINT('Ctrl Pts',(-3.53773177400349,-25.0566841622527,4.08581672291636));
#4600=CARTESIAN_POINT('Ctrl Pts',(-2.69110791178932,-24.028567338781,4.20040005624976));
#4601=CARTESIAN_POINT('Ctrl Pts',(-2.13837982562106,-23.6195385131152,4.25769172291635));
#4602=CARTESIAN_POINT('Ctrl Pts',(-0.900692885453703,-23.1092732864771,
4.37227505624977));
#4603=CARTESIAN_POINT('Ctrl Pts',(-0.216897527488987,-23.0085744595606,
4.42956672291635));
#4604=CARTESIAN_POINT('Ctrl Pts',(1.12205514727662,-23.142679210215,4.54415005624977));
#4605=CARTESIAN_POINT('Ctrl Pts',(1.775926366677,-23.3774077699852,4.60144172291642));
#4606=CARTESIAN_POINT('Ctrl Pts',(2.89930290271304,-24.1306923663646,4.71602505624971));
#4607=CARTESIAN_POINT('Ctrl Pts',(3.36770385261388,-24.6485723106026,4.77331672291647));
#4608=CARTESIAN_POINT('Ctrl Pts',(4.00659313686357,-25.8485567155787,4.88790005624965));
#4609=CARTESIAN_POINT('Ctrl Pts',(4.17642310008015,-26.5295384946699,4.94519172291645));
#4610=CARTESIAN_POINT('Ctrl Pts',(4.17420441267586,-27.8959067178885,5.05977505624967));
#4611=CARTESIAN_POINT('Ctrl Pts',(4.00210435901772,-28.5799860845476,5.11706672291619));
#4612=CARTESIAN_POINT('Ctrl Pts',(3.3527905998087,-29.7900600615589,5.23165005624993));
#4613=CARTESIAN_POINT('Ctrl Pts',(2.87615082723203,-30.314871874706,5.28894172291612));
#4614=CARTESIAN_POINT('Ctrl Pts',(1.72734004962141,-31.0798143026723,5.40352505625001));
#4615=CARTESIAN_POINT('Ctrl Pts',(1.05623826824525,-31.3191686631573,5.46081672291647));
#4616=CARTESIAN_POINT('Ctrl Pts',(-0.324386630517576,-31.4529189242652,
5.57540005624965));
#4617=CARTESIAN_POINT('Ctrl Pts',(-1.03259427822014,-31.3471336106709,5.63269172291625));
#4618=CARTESIAN_POINT('Ctrl Pts',(-2.31962660867283,-30.8116258742433,5.74727505624988));
#4619=CARTESIAN_POINT('Ctrl Pts',(-2.89719962320057,-30.3823662711092,5.80456672291639));
#4620=CARTESIAN_POINT('Ctrl Pts',(-3.78420541000443,-29.2980492552136,5.91915005624974));
#4621=CARTESIAN_POINT('Ctrl Pts',(-4.09274828993971,-28.6439951522933,5.97644172291612));
#4622=CARTESIAN_POINT('Ctrl Pts',(-4.36522137220295,-27.2628078488887,6.09102505625001));
#4623=CARTESIAN_POINT('Ctrl Pts',(-4.32883842763837,-26.5369854607524,6.14831672291658));
#4624=CARTESIAN_POINT('Ctrl Pts',(-3.91604629967915,-25.1838353260752,6.26290005624954));
#4625=CARTESIAN_POINT('Ctrl Pts',(-3.53998077585005,-24.5578175514078,6.32019172291661));
#4626=CARTESIAN_POINT('Ctrl Pts',(-2.53317668706739,-23.5541511604319,6.43477505624951));
#4627=CARTESIAN_POINT('Ctrl Pts',(-1.90336339087076,-23.1775005077857,6.49206672291618));
#4628=CARTESIAN_POINT('Ctrl Pts',(-0.535707634461822,-22.7649451919414,
6.60665005624995));
#4629=CARTESIAN_POINT('Ctrl Pts',(0.200842052573385,-22.7294864032627,6.66394172291654));
#4630=CARTESIAN_POINT('Ctrl Pts',(1.60825741243838,-23.0117008784331,6.77852505624958));
#4631=CARTESIAN_POINT('Ctrl Pts',(2.27776629761871,-23.3291566705507,6.83581672291669));
#4632=CARTESIAN_POINT('Ctrl Pts',(3.39129936374918,-24.2458798314691,6.95040005624944));
#4633=CARTESIAN_POINT('Ctrl Pts',(3.8342243732566,-24.8443116308563,7.00769172291627));
#4634=CARTESIAN_POINT('Ctrl Pts',(4.38677541995195,-26.1840855712311,7.12227505624986));
#4635=CARTESIAN_POINT('Ctrl Pts',(4.49582343090945,-26.9241665562002,7.1795667229166));
#4636=CARTESIAN_POINT('Ctrl Pts',(4.35088796536903,-28.3730853248421,7.29415005624953));
#4637=CARTESIAN_POINT('Ctrl Pts',(4.09698986764256,-29.0805318136941,7.35144172291661));
#4638=CARTESIAN_POINT('Ctrl Pts',(3.28231577569086,-30.295784222617,7.46602505624951));
#4639=CARTESIAN_POINT('Ctrl Pts',(2.72227460111075,-30.8023978842609,7.52331672291659));
#4640=CARTESIAN_POINT('Ctrl Pts',(1.42483950789472,-31.4933756465881,7.63790005624954));
#4641=CARTESIAN_POINT('Ctrl Pts',(0.688661495622512,-31.6770315464534,7.69519172291528));
#4642=CARTESIAN_POINT('Ctrl Pts',(-0.788204900376376,-31.6748128590733,
7.80977505625085));
#4643=CARTESIAN_POINT('Ctrl Pts',(-1.52748050021878,-31.4888868687303,7.86706672291669));
#4644=CARTESIAN_POINT('Ctrl Pts',(-2.83500516546561,-30.7874846314674,7.98165005624943));
#4645=CARTESIAN_POINT('Ctrl Pts',(-3.40197820894101,-30.2726321471241,8.03894172291615));
#4646=CARTESIAN_POINT('Ctrl Pts',(-4.22831013251146,-29.0319454966501,8.15352505624997));
#4647=CARTESIAN_POINT('Ctrl Pts',(-4.48683403091752,-28.3072684458016,8.21081672291615));
#4648=CARTESIAN_POINT('Ctrl Pts',(-4.63141500694981,-26.8166774531803,8.32540005624997));
#4649=CARTESIAN_POINT('Ctrl Pts',(-4.51728050926608,-26.0521841784596,8.38269172291643));
#4650=CARTESIAN_POINT('Ctrl Pts',(-3.93948695283954,-24.6630648478093,8.49727505624969));
#4651=CARTESIAN_POINT('Ctrl Pts',(-3.47633116581651,-24.0397881200713,8.55456672291628));
#4652=CARTESIAN_POINT('Ctrl Pts',(-2.3065979072983,-23.082683034536,8.66915005624984));
#4653=CARTESIAN_POINT('Ctrl Pts',(-1.60110545776092,-22.7498116285361,8.72644172291626));
#4654=CARTESIAN_POINT('Ctrl Pts',(-0.1115431730045,-22.455781422157,8.84102505624986));
#4655=CARTESIAN_POINT('Ctrl Pts',(0.671112174616573,-22.4949563909962,8.89831672291601));
#4656=CARTESIAN_POINT('Ctrl Pts',(2.13000246784507,-22.9398244453587,9.01290005625012));
#4657=CARTESIAN_POINT('Ctrl Pts',(2.80482628686612,-23.3451431864166,9.07019172291636));
#4658=CARTESIAN_POINT('Ctrl Pts',(3.88662668511606,-24.4300812824538,9.18477505624977));
#4659=CARTESIAN_POINT('Ctrl Pts',(4.29253055496877,-25.1087006230277,9.24206672291584));
#4660=CARTESIAN_POINT('Ctrl Pts',(4.73716179724122,-26.5820965379602,9.35665005625028));
#4661=CARTESIAN_POINT('Ctrl Pts',(4.77541261016421,-27.3754791844964,9.41394172291549));
#4662=CARTESIAN_POINT('Ctrl Pts',(4.47164101091353,-28.8912695257086,9.52852505625063));
#4663=CARTESIAN_POINT('Ctrl Pts',(4.12985669269715,-29.6122167575113,9.58581672291576));
#4664=CARTESIAN_POINT('Ctrl Pts',(3.1430342330799,-30.8111660662582,9.70040005625036));
#4665=CARTESIAN_POINT('Ctrl Pts',(2.49889872045615,-31.2879872596437,9.75769172291579));
#4666=CARTESIAN_POINT('Ctrl Pts',(1.05703777990366,-31.8828241263658,9.87227505625033));
#4667=CARTESIAN_POINT('Ctrl Pts',(0.260671167899412,-32.0002213213825,9.92956672291638));
#4668=CARTESIAN_POINT('Ctrl Pts',(-1.29821369458701,-31.8444551409501,10.0441500562497));
#4669=CARTESIAN_POINT('Ctrl Pts',(-2.05923545291888,-31.5713875052691,10.1014417229165));
#4670=CARTESIAN_POINT('Ctrl Pts',(-3.36636373470387,-30.6953239177476,10.2160250562496));
#4671=CARTESIAN_POINT('Ctrl Pts',(-3.91119010810414,-30.0931215128015,10.2733167229167));
#4672=CARTESIAN_POINT('Ctrl Pts',(-4.65425634850692,-28.6982357313908,10.3879000562494));
#4673=CARTESIAN_POINT('Ctrl Pts',(-4.85173818484261,-27.906861497377,10.4451917229149));
#4674=CARTESIAN_POINT('Ctrl Pts',(-4.85062884134398,-27.1131792015253,10.5024833895831));
#4675=CARTESIAN_POINT('Origin',(-3.5,-27.1629509039024,-4.33680868994202E-16));
#4676=CARTESIAN_POINT('Origin',(-4.85063016993195,-27.162950903902,11.));
#4677=CARTESIAN_POINT('Origin',(-3.5,-27.1629509039024,-4.33680868994202E-16));
#4678=CARTESIAN_POINT('Ctrl Pts',(-3.49996080530815,-27.2127230666419,22.4975165628198));
#4679=CARTESIAN_POINT('Ctrl Pts',(-3.49923858446785,-27.7853227106402,22.4402329418509));
#4680=CARTESIAN_POINT('Ctrl Pts',(-3.35442400014962,-28.3588108293565,22.3829524076267));
#4681=CARTESIAN_POINT('Ctrl Pts',(-2.53805890913148,-29.8820941336696,22.2111092614391));
#4682=CARTESIAN_POINT('Ctrl Pts',(-1.46143501137141,-30.6017071597437,22.0965431123954));
#4683=CARTESIAN_POINT('Ctrl Pts',(0.859993909463204,-30.8281716102345,21.8674140533199));
#4684=CARTESIAN_POINT('Ctrl Pts',(2.07105132984979,-30.3269875071567,21.7528496294383));
#4685=CARTESIAN_POINT('Ctrl Pts',(3.56717700801455,-28.5011027334814,21.5237158877512));
#4686=CARTESIAN_POINT('Ctrl Pts',(3.82655802944863,-27.2003585446699,21.4091531369767));
#4687=CARTESIAN_POINT('Ctrl Pts',(3.13176866916735,-24.9149704304093,21.1800148858282));
#4688=CARTESIAN_POINT('Ctrl Pts',(2.18340277243941,-23.9654078612039,21.0654537578317));
#4689=CARTESIAN_POINT('Ctrl Pts',(-0.129624475723444,-23.26492626726,20.8363111624828));
#4690=CARTESIAN_POINT('Ctrl Pts',(-1.46146161962901,-23.5287714044906,20.7217516085899));
#4691=CARTESIAN_POINT('Ctrl Pts',(-3.35087032746474,-25.0803824700087,20.4926048268444));
#4692=CARTESIAN_POINT('Ctrl Pts',(-3.87760724316326,-26.3487572317876,20.3780467999886));
#4693=CARTESIAN_POINT('Ctrl Pts',(-3.63476056023195,-28.8097599072106,20.1488959825923));
#4694=CARTESIAN_POINT('Ctrl Pts',(-2.86424004281594,-29.965541294796,20.0343394372402));
#4695=CARTESIAN_POINT('Ctrl Pts',(-0.658453525508203,-31.1444028451946,
19.8051847283177));
#4696=CARTESIAN_POINT('Ctrl Pts',(0.746295607863299,-31.1460497722331,19.6906296204221));
#4697=CARTESIAN_POINT('Ctrl Pts',(2.97686521751534,-29.9539838567283,19.4614711577696));
#4698=CARTESIAN_POINT('Ctrl Pts',(3.76753534062837,-28.7739677375461,19.3469174447372));
#4699=CARTESIAN_POINT('Ctrl Pts',(4.01866309430747,-26.2291292657398,19.1177553601879));
#4700=CARTESIAN_POINT('Ctrl Pts',(3.47096346939119,-24.9015823386939,19.0032030007967));
#4701=CARTESIAN_POINT('Ctrl Pts',(1.47301680764982,-23.2609008561182,18.7740374205694));
#4702=CARTESIAN_POINT('Ctrl Pts',(0.0495864900580295,-22.9755165719832,
18.6594863749187));
#4703=CARTESIAN_POINT('Ctrl Pts',(-2.45153366210842,-23.7331018039879,18.4303174198824));
#4704=CARTESIAN_POINT('Ctrl Pts',(-3.49083915992615,-24.7690401632385,18.3157676493834));
#4705=CARTESIAN_POINT('Ctrl Pts',(-4.25889868811986,-27.2963083875918,18.0865954352922));
#4706=CARTESIAN_POINT('Ctrl Pts',(-3.97206991737307,-28.7513902818761,17.9720469025882));
#4707=CARTESIAN_POINT('Ctrl Pts',(-2.27985145267618,-30.8159510369377,17.7428715404485));
#4708=CARTESIAN_POINT('Ctrl Pts',(-0.896239671425334,-31.3920117915409,
17.6283242093665));
#4709=CARTESIAN_POINT('Ctrl Pts',(1.11729400206607,-31.1951401445063,17.4564404065291));
#4710=CARTESIAN_POINT('Ctrl Pts',(1.77292736544793,-30.9607175289896,17.3991671837723));
#4711=CARTESIAN_POINT('Ctrl Pts',(2.90077819546148,-30.2083455155492,17.2845772407366));
#4712=CARTESIAN_POINT('Ctrl Pts',(3.37094068270095,-29.6898924273955,17.2273043052763));
#4713=CARTESIAN_POINT('Ctrl Pts',(4.01431528178035,-28.4885418055165,17.1127136336125));
#4714=CARTESIAN_POINT('Ctrl Pts',(4.18547814755316,-27.8061836720571,17.0554409812454));
#4715=CARTESIAN_POINT('Ctrl Pts',(4.18663754642286,-26.4363906879155,16.9408495931827));
#4716=CARTESIAN_POINT('Ctrl Pts',(4.0150884896742,-25.7504104196397,16.8835772197774));
#4717=CARTESIAN_POINT('Ctrl Pts',(3.36714801944677,-24.5356000655517,16.7689851273202));
#4718=CARTESIAN_POINT('Ctrl Pts',(2.89009172502227,-24.0087892511978,16.7117130288065));
#4719=CARTESIAN_POINT('Ctrl Pts',(1.7402086697919,-23.2389101700822,16.5971202437039));
#4720=CARTESIAN_POINT('Ctrl Pts',(1.06776209555002,-22.9979372337308,16.5398484160816));
#4721=CARTESIAN_POINT('Ctrl Pts',(-0.31623274086958,-22.8602643582168,16.4252549498493));
#4722=CARTESIAN_POINT('Ctrl Pts',(-1.02644456351773,-22.9652272065363,16.3679833891743));
#4723=CARTESIAN_POINT('Ctrl Pts',(-2.31841804031954,-23.4988447092972,16.2533892531115));
#4724=CARTESIAN_POINT('Ctrl Pts',(-2.8982081868341,-23.9283243595328,16.1961179554988));
#4725=CARTESIAN_POINT('Ctrl Pts',(-3.79057690805528,-25.0133430809505,16.0815231606726));
#4726=CARTESIAN_POINT('Ctrl Pts',(-4.10102526300207,-25.6686660718134,16.024252122308));
#4727=CARTESIAN_POINT('Ctrl Pts',(-4.37797862822859,-27.0530885949626,15.909656679556));
#4728=CARTESIAN_POINT('Ctrl Pts',(-4.34271119481323,-27.7809795875592,15.8523858966855));
#4729=CARTESIAN_POINT('Ctrl Pts',(-3.93237495733071,-29.1392105157473,15.7377898166423));
#4730=CARTESIAN_POINT('Ctrl Pts',(-3.55632299466167,-29.7676390000464,15.6805192855666));
#4731=CARTESIAN_POINT('Ctrl Pts',(-2.54926136464863,-30.7770591329649,15.5659225786565));
#4732=CARTESIAN_POINT('Ctrl Pts',(-1.91829944896927,-31.1558975036044,15.5086522957306));
#4733=CARTESIAN_POINT('Ctrl Pts',(-0.547625232561448,-31.5734932671083,
15.3940549721839));
#4734=CARTESIAN_POINT('Ctrl Pts',(0.191015893047531,-31.6103769951178,15.3367849338207));
#4735=CARTESIAN_POINT('Ctrl Pts',(1.60357971999462,-31.3312243440256,15.222187003658));
#4736=CARTESIAN_POINT('Ctrl Pts',(2.27566348949658,-31.0140495365735,15.1649172063298));
#4737=CARTESIAN_POINT('Ctrl Pts',(3.39529563646339,-30.0975823003571,15.0503186793825));
#4738=CARTESIAN_POINT('Ctrl Pts',(3.84068011604263,-29.498165831456,14.9930491196166));
#4739=CARTESIAN_POINT('Ctrl Pts',(4.39882341638518,-28.1556730779471,14.8784500055221));
#4740=CARTESIAN_POINT('Ctrl Pts',(4.50961669585736,-27.4135215250066,14.8211806798972));
#4741=CARTESIAN_POINT('Ctrl Pts',(4.36838003559756,-25.9594643878227,14.706580988118));
#4742=CARTESIAN_POINT('Ctrl Pts',(4.11506029041641,-25.249312658991,14.64931189327));
#4743=CARTESIAN_POINT('Ctrl Pts',(3.30121940653211,-24.0276707334375,14.5347116330704));
#4744=CARTESIAN_POINT('Ctrl Pts',(2.74039982125199,-23.5183420501783,14.4774427656859));
#4745=CARTESIAN_POINT('Ctrl Pts',(1.44062797695419,-22.8212395033473,14.3628419461743));
#4746=CARTESIAN_POINT('Ctrl Pts',(0.702445412717409,-22.6355127980759,14.3055733029845));
#4747=CARTESIAN_POINT('Ctrl Pts',(-0.779466818671152,-22.6333745501127,
14.1909719330902));
#4748=CARTESIAN_POINT('Ctrl Pts',(-1.52154027083034,-22.8183992461163,14.133703510881));
#4749=CARTESIAN_POINT('Ctrl Pts',(-2.83568124304263,-23.5183337811168,14.0191015993632));
#4750=CARTESIAN_POINT('Ctrl Pts',(-3.40560315083273,-24.0337181522913,13.961833394971));
#4751=CARTESIAN_POINT('Ctrl Pts',(-4.23856228598614,-25.2762788645662,13.8472309504247));
#4752=CARTESIAN_POINT('Ctrl Pts',(-4.49948190557238,-26.0028485522343,13.789962960732));
#4753=CARTESIAN_POINT('Ctrl Pts',(-4.6490886604143,-27.4983069550493,13.6753599915962));
#4754=CARTESIAN_POINT('Ctrl Pts',(-4.53619916170288,-28.2656495705488,13.6180922135344));
#4755=CARTESIAN_POINT('Ctrl Pts',(-3.96055736820013,-29.661540425932,13.5034887280845));
#4756=CARTESIAN_POINT('Ctrl Pts',(-3.49715379610915,-30.2879729181394,13.4462211586326));
#4757=CARTESIAN_POINT('Ctrl Pts',(-2.32608670582391,-31.2521669466145,13.3316171649959));
#4758=CARTESIAN_POINT('Ctrl Pts',(-1.61885949052411,-31.5877524818146,13.2743498011764));
#4759=CARTESIAN_POINT('Ctrl Pts',(-0.124696310905245,-31.8874771910156,
13.1597453073302));
#4760=CARTESIAN_POINT('Ctrl Pts',(0.660815950487942,-31.8499065009576,13.1024781462114));
#4761=CARTESIAN_POINT('Ctrl Pts',(2.12655441499977,-31.4079152525417,12.9878731599857));
#4762=CARTESIAN_POINT('Ctrl Pts',(2.80470906709709,-31.0026671109796,12.9306061986817));
#4763=CARTESIAN_POINT('Ctrl Pts',(3.89400923429049,-29.9170086021089,12.8160007277616));
#4764=CARTESIAN_POINT('Ctrl Pts',(4.30293326762064,-29.2368576811396,12.7587339634332));
#4765=CARTESIAN_POINT('Ctrl Pts',(4.7539165316201,-27.7592163768989,12.6441280153592));
#4766=CARTESIAN_POINT('Ctrl Pts',(4.79414098254103,-26.9630153236094,12.5868614452008));
#4767=CARTESIAN_POINT('Ctrl Pts',(4.49400280036036,-25.4403847040206,12.4722550273998));
#4768=CARTESIAN_POINT('Ctrl Pts',(4.15263788850493,-24.7159678807397,12.4149886486516));
#4769=CARTESIAN_POINT('Ctrl Pts',(3.16577605609634,-23.509168568218,12.3003817683865));
#4770=CARTESIAN_POINT('Ctrl Pts',(2.52035612956819,-23.0290393182234,12.2431155783337));
#4771=CARTESIAN_POINT('Ctrl Pts',(1.07469387470518,-22.4272153063553,12.1285082427589));
#4772=CARTESIAN_POINT('Ctrl Pts',(0.275594950052222,-22.3074707664612,12.0712422387231));
#4773=CARTESIAN_POINT('Ctrl Pts',(-1.84866925673703,-22.5128307999096,11.915740909639));
#4774=CARTESIAN_POINT('Ctrl Pts',(-3.12603843365803,-23.2394090136764,11.8175868796768));
#4775=CARTESIAN_POINT('Ctrl Pts',(-4.3320981071104,-24.8804056714019,11.6703283443192));
#4776=CARTESIAN_POINT('Ctrl Pts',(-4.61674384788206,-25.5146057311216,11.6212316068295));
#4777=CARTESIAN_POINT('Ctrl Pts',(-4.83246869871424,-26.5137556598953,11.5476071541803));
#4778=CARTESIAN_POINT('Ctrl Pts',(-4.86977624768409,-26.8545749239038,11.5230638633071));
#4779=CARTESIAN_POINT('Ctrl Pts',(-4.87146626433893,-27.5373932865771,11.4739653075255));
#4780=CARTESIAN_POINT('Ctrl Pts',(-4.84802535953691,-27.8775521427343,11.449426192242));
#4781=CARTESIAN_POINT('Ctrl Pts',(-4.83316291400662,-28.2179621014742,11.4248820703399));
#4782=CARTESIAN_POINT('Ctrl Pts',(-3.4999738703761,-27.2127229078506,22.4975165797347));
#4783=CARTESIAN_POINT('Ctrl Pts',(-3.49925167603735,-27.7853247308279,22.440232944449));
#4784=CARTESIAN_POINT('Ctrl Pts',(-3.35443660091437,-28.3588149144678,22.3829524301632));
#4785=CARTESIAN_POINT('Ctrl Pts',(-2.53806849928542,-29.8821040197979,22.2111092380756));
#4786=CARTESIAN_POINT('Ctrl Pts',(-1.46144078073265,-30.6017196666142,22.0965431306844));
#4787=CARTESIAN_POINT('Ctrl Pts',(0.859996801537081,-30.8281850765549,21.8674140111125));
#4788=CARTESIAN_POINT('Ctrl Pts',(2.07105852363703,-30.3269992526889,21.7528496283989));
#4789=CARTESIAN_POINT('Ctrl Pts',(3.56718981158329,-28.5011078101942,21.5237158269035));
#4790=CARTESIAN_POINT('Ctrl Pts',(3.82657179215288,-27.2003590887291,21.4091531168235));
#4791=CARTESIAN_POINT('Ctrl Pts',(3.13178000345364,-24.9149626050602,21.1800148065395));
#4792=CARTESIAN_POINT('Ctrl Pts',(2.18341087092642,-23.965396720214,21.0654537187747));
#4793=CARTESIAN_POINT('Ctrl Pts',(-0.129624685393233,-23.2649124957247,
20.8363110649486));
#4794=CARTESIAN_POINT('Ctrl Pts',(-1.46146638375645,-23.5287584813108,20.7217515508348));
#4795=CARTESIAN_POINT('Ctrl Pts',(-3.35088189452712,-25.0803749934778,20.4926047112563));
#4796=CARTESIAN_POINT('Ctrl Pts',(-3.87762063512896,-26.3487540133528,20.3780467237371));
#4797=CARTESIAN_POINT('Ctrl Pts',(-3.63477320284824,-28.8097653712122,20.1488958491381));
#4798=CARTESIAN_POINT('Ctrl Pts',(-2.86425015889221,-29.9655506417163,20.0343393426895));
#4799=CARTESIAN_POINT('Ctrl Pts',(-0.658456006019151,-31.1444163926324,
19.8051845771816));
#4800=CARTESIAN_POINT('Ctrl Pts',(0.746297759417265,-31.1460633761619,19.690629507766));
#4801=CARTESIAN_POINT('Ctrl Pts',(2.97687510367843,-29.9539934454761,19.4614709891321));
#4802=CARTESIAN_POINT('Ctrl Pts',(3.76754784711476,-28.7739735063694,19.3469173141651));
#4803=CARTESIAN_POINT('Ctrl Pts',(4.01867655925237,-26.2291263727762,19.1177551742263));
#4804=CARTESIAN_POINT('Ctrl Pts',(3.47097521400111,-24.9015751449147,19.0032028524946));
#4805=CARTESIAN_POINT('Ctrl Pts',(1.4730218826762,-23.260888053339,18.7740372174575));
#4806=CARTESIAN_POINT('Ctrl Pts',(0.0495870334641008,-22.9755028102541,
18.6594862090688));
#4807=CARTESIAN_POINT('Ctrl Pts',(-2.45154148772098,-23.733090471763,18.4303171997907));
#4808=CARTESIAN_POINT('Ctrl Pts',(-3.49085030038139,-24.7690320660619,18.3157674661644));
#4809=CARTESIAN_POINT('Ctrl Pts',(-4.25891245790086,-27.2963085987281,18.086595198388));
#4810=CARTESIAN_POINT('Ctrl Pts',(-3.97208283893911,-28.7513950463358,17.9720467021754));
#4811=CARTESIAN_POINT('Ctrl Pts',(-2.27985892683281,-30.8159626032593,17.7428712868959));
#4812=CARTESIAN_POINT('Ctrl Pts',(-0.896242888528564,-31.3920251821923,
17.6283239919319));
#4813=CARTESIAN_POINT('Ctrl Pts',(1.11729729633126,-31.1951529721948,17.4564401496407));
#4814=CARTESIAN_POINT('Ctrl Pts',(1.77293266626044,-30.9607296662042,17.3991669448048));
#4815=CARTESIAN_POINT('Ctrl Pts',(2.90078714764444,-30.2083552754577,17.2845769755984));
#4816=CARTESIAN_POINT('Ctrl Pts',(3.37095107897927,-29.6899006325071,17.2273040579683));
#4817=CARTESIAN_POINT('Ctrl Pts',(4.01432777756716,-28.4885461927946,17.1127133602641));
#4818=CARTESIAN_POINT('Ctrl Pts',(4.18549118397379,-27.8061860074247,17.0554407256377));
#4819=CARTESIAN_POINT('Ctrl Pts',(4.18665063468174,-26.4363886665888,16.9408493116638));
#4820=CARTESIAN_POINT('Ctrl Pts',(4.01510108746783,-25.7504063338809,16.8835769559103));
#4821=CARTESIAN_POINT('Ctrl Pts',(3.36715860920047,-24.5355921131514,16.7689848376699));
#4822=CARTESIAN_POINT('Ctrl Pts',(2.89010090908047,-24.0087797093735,16.71171275672));
#4823=CARTESIAN_POINT('Ctrl Pts',(1.74021426019986,-23.2388981648313,16.5971199459608));
#4824=CARTESIAN_POINT('Ctrl Pts',(1.06776569703458,-22.9979244893974,16.5398481358153));
#4825=CARTESIAN_POINT('Ctrl Pts',(-0.316233469917037,-22.8602511354241,
16.4252546440519));
#4826=CARTESIAN_POINT('Ctrl Pts',(-1.02644739499413,-22.9652142695065,16.3679831007674));
#4827=CARTESIAN_POINT('Ctrl Pts',(-2.31842491646956,-23.4988333917331,16.2533889392978));
#4828=CARTESIAN_POINT('Ctrl Pts',(-2.89821678241042,-23.9283142850487,16.1961176589903));
#4829=CARTESIAN_POINT('Ctrl Pts',(-3.79058830723667,-25.0133363413519,16.0815228388804));
#4830=CARTESIAN_POINT('Ctrl Pts',(-4.10103759256865,-25.6686612390088,16.0242518177364));
#4831=CARTESIAN_POINT('Ctrl Pts',(-4.37799185824023,-27.0530880248399,15.9096563498227));
#4832=CARTESIAN_POINT('Ctrl Pts',(-4.34272434648572,-27.7809811376122,15.852385584089));
#4833=CARTESIAN_POINT('Ctrl Pts',(-3.93238689367438,-29.1392162495564,15.7377894790049));
#4834=CARTESIAN_POINT('Ctrl Pts',(-3.5563338624862,-29.7676465667086,15.680518964983));
#4835=CARTESIAN_POINT('Ctrl Pts',(-2.54926918843734,-30.7770698163966,15.5659222331516));
#4836=CARTESIAN_POINT('Ctrl Pts',(-1.91830546644135,-31.155909299737,15.5086519671974));
#4837=CARTESIAN_POINT('Ctrl Pts',(-0.547627096231643,-31.5735063769721,
15.394054618848));
#4838=CARTESIAN_POINT('Ctrl Pts',(0.191016146883062,-31.6103902347893,15.3367845973752));
#4839=CARTESIAN_POINT('Ctrl Pts',(1.60358425638348,-31.3312367841738,15.2221866425272));
#4840=CARTESIAN_POINT('Ctrl Pts',(2.27566995450071,-31.0140610930252,15.1649168620087));
#4841=CARTESIAN_POINT('Ctrl Pts',(3.39530550137407,-30.0975911329029,15.0503183104925));
#4842=CARTESIAN_POINT('Ctrl Pts',(3.84069126522877,-29.4981729755389,14.9930487674564));
#4843=CARTESIAN_POINT('Ctrl Pts',(4.39883627990966,-28.1556762170847,14.8784496289083));
#4844=CARTESIAN_POINT('Ctrl Pts',(4.50962989605486,-27.4135225696958,14.8211803199342));
#4845=CARTESIAN_POINT('Ctrl Pts',(4.36839285973953,-25.9594610923935,14.7065806038156));
#4846=CARTESIAN_POINT('Ctrl Pts',(4.11507242416446,-25.2493073577679,14.6493115255399));
#4847=CARTESIAN_POINT('Ctrl Pts',(3.30122916269765,-24.0276617819218,14.5347112411141));
#4848=CARTESIAN_POINT('Ctrl Pts',(2.7404080230466,-23.5183316552038,14.4774423902243));
#4849=CARTESIAN_POINT('Ctrl Pts',(1.44063236119846,-22.8212270099635,14.3628415465987));
#4850=CARTESIAN_POINT('Ctrl Pts',(0.70244774573194,-22.6354997644271,14.3055729198267));
#4851=CARTESIAN_POINT('Ctrl Pts',(-0.779468841558015,-22.6333614654686,
14.1909715259295));
#4852=CARTESIAN_POINT('Ctrl Pts',(-1.52154435736691,-22.8183866519466,14.1337031200619));
#4853=CARTESIAN_POINT('Ctrl Pts',(-2.83568919509919,-23.5183231953511,14.0191011846514));
#4854=CARTESIAN_POINT('Ctrl Pts',(-3.40561269160967,-24.0337089718608,13.9618329965252));
#4855=CARTESIAN_POINT('Ctrl Pts',(-4.2385742890103,-25.2762732775619,13.8472305281954));
#4856=CARTESIAN_POINT('Ctrl Pts',(-4.49949464722015,-26.0028449534998,13.7899625546938));
#4857=CARTESIAN_POINT('Ctrl Pts',(-4.64910187957824,-27.4983076860702,13.6753595618827));
#4858=CARTESIAN_POINT('Ctrl Pts',(-4.53621209500216,-28.2656524031987,13.6180917999378));
#4859=CARTESIAN_POINT('Ctrl Pts',(-3.96056868157127,-29.661547302102,13.5034882909199));
#4860=CARTESIAN_POINT('Ctrl Pts',(-3.49716386668666,-30.2879815129736,13.4462207375114));
#4861=CARTESIAN_POINT('Ctrl Pts',(-2.32609344166591,-31.2521783437993,13.3316167204129));
#4862=CARTESIAN_POINT('Ctrl Pts',(-1.61886432018724,-31.5877648088394,13.274349372564));
#4863=CARTESIAN_POINT('Ctrl Pts',(-0.124696878631275,-31.88749041744,13.1597448553615));
#4864=CARTESIAN_POINT('Ctrl Pts',(0.66081750213183,-31.8499196488467,13.1024777101411));
#4865=CARTESIAN_POINT('Ctrl Pts',(2.12656014922713,-31.4079271845322,12.9878727006634));
#4866=CARTESIAN_POINT('Ctrl Pts',(2.80471663336618,-31.0026779746561,12.9306057551862));
#4867=CARTESIAN_POINT('Ctrl Pts',(3.89401991600716,-29.9170164218118,12.8160002611176));
#4868=CARTESIAN_POINT('Ctrl Pts',(4.30294506141158,-29.2368636950917,12.7587335125451));
#4869=CARTESIAN_POINT('Ctrl Pts',(4.75392963799469,-27.7592182377462,12.6441275414253));
#4870=CARTESIAN_POINT('Ctrl Pts',(4.79415421843191,-26.9630150677512,12.5868609869525));
#4871=CARTESIAN_POINT('Ctrl Pts',(4.49401523604375,-25.4403801667867,12.4722545462074));
#4872=CARTESIAN_POINT('Ctrl Pts',(4.15264944060989,-24.7159614157411,12.4149881830751));
#4873=CARTESIAN_POINT('Ctrl Pts',(3.16578488425683,-23.5091587046932,12.3003812799668));
#4874=CARTESIAN_POINT('Ctrl Pts',(2.52036326977255,-23.029028171125,12.2431151054609));
#4875=CARTESIAN_POINT('Ctrl Pts',(1.07469701059825,-22.4272024461661,12.1285077471428));
#4876=CARTESIAN_POINT('Ctrl Pts',(0.275595992279665,-22.3074575699848,12.0712417585854));
#4877=CARTESIAN_POINT('Ctrl Pts',(-1.84867410165387,-22.5128181147607,11.9157403987775));
#4878=CARTESIAN_POINT('Ctrl Pts',(-3.126046686507,-23.239398259682,11.8175863798246));
#4879=CARTESIAN_POINT('Ctrl Pts',(-4.33210964259808,-24.8803992898634,11.6703278427641));
#4880=CARTESIAN_POINT('Ctrl Pts',(-4.61675618009252,-25.5146010763329,11.6212310968322));
#4881=CARTESIAN_POINT('Ctrl Pts',(-4.83248163235518,-26.5137536581576,11.5476066464927));
#4882=CARTESIAN_POINT('Ctrl Pts',(-4.86978929142209,-26.8545738310615,11.5230633554386));
#4883=CARTESIAN_POINT('Ctrl Pts',(-4.87147933058113,-27.5373940588702,11.473964789632));
#4884=CARTESIAN_POINT('Ctrl Pts',(-4.84803840451156,-27.877552675042,11.4494256757284));
#4885=CARTESIAN_POINT('Ctrl Pts',(-4.83317595898128,-28.217962633782,11.4248815538263));
#4886=CARTESIAN_POINT('Ctrl Pts',(-3.4999869352734,-27.2127227490105,22.4975165961398));
#4887=CARTESIAN_POINT('Ctrl Pts',(-3.49926476744378,-27.7853267509384,22.4402329465374));
#4888=CARTESIAN_POINT('Ctrl Pts',(-3.35444920153117,-28.3588189994771,22.3829524521897));
#4889=CARTESIAN_POINT('Ctrl Pts',(-2.53807808935145,-29.8821139057597,22.2111092142027));
#4890=CARTESIAN_POINT('Ctrl Pts',(-1.46144655006658,-30.6017321733,22.0965431484635));
#4891=CARTESIAN_POINT('Ctrl Pts',(0.859999693521789,-30.8281985427089,21.867413968396));
#4892=CARTESIAN_POINT('Ctrl Pts',(2.07106571728588,-30.3270109980947,21.7528496268498));
#4893=CARTESIAN_POINT('Ctrl Pts',(3.56720261496358,-28.5011128868879,21.5237157655468));
#4894=CARTESIAN_POINT('Ctrl Pts',(3.82658555467438,-27.2003596328324,21.4091530961607));
#4895=CARTESIAN_POINT('Ctrl Pts',(3.1317913376183,-24.9149547798571,21.180014726742));
#4896=CARTESIAN_POINT('Ctrl Pts',(2.18341896934776,-23.9653855794009,21.0654536792084));
#4897=CARTESIAN_POINT('Ctrl Pts',(-0.129624895009774,-23.2648987243724,
20.8363109669058));
#4898=CARTESIAN_POINT('Ctrl Pts',(-1.46147114777366,-23.5287455582848,20.7217514925706));
#4899=CARTESIAN_POINT('Ctrl Pts',(-3.35089346140745,-25.0803675170051,20.4926045951597));
#4900=CARTESIAN_POINT('Ctrl Pts',(-3.87763402690497,-26.3487507949125,20.3780466469766));
#4901=CARTESIAN_POINT('Ctrl Pts',(-3.63478584531403,-28.8097708350949,20.1488957151756));
#4902=CARTESIAN_POINT('Ctrl Pts',(-2.86426027486676,-29.9655599884758,20.0343392476302));
#4903=CARTESIAN_POINT('Ctrl Pts',(-0.658458486544607,-31.1444299398784,
19.8051844255374));
#4904=CARTESIAN_POINT('Ctrl Pts',(0.746299910894372,-31.1460769799159,19.6906293946012));
#4905=CARTESIAN_POINT('Ctrl Pts',(2.97688498967388,-29.9540030341285,19.4614708199869));
#4906=CARTESIAN_POINT('Ctrl Pts',(3.76756035341267,-28.7739792751586,19.3469171830846));
#4907=CARTESIAN_POINT('Ctrl Pts',(4.01869002402406,-26.2291234798987,19.1177549877571));
#4908=CARTESIAN_POINT('Ctrl Pts',(3.47098695847717,-24.9015679512733,19.0032027036843));
#4909=CARTESIAN_POINT('Ctrl Pts',(1.47302695767718,-23.2608752507521,18.7740370138381));
#4910=CARTESIAN_POINT('Ctrl Pts',(0.0495875769098387,-22.9754890487136,
18.6594860427109));
#4911=CARTESIAN_POINT('Ctrl Pts',(-2.45154931318775,-23.733079139667,18.4303169791917));
#4912=CARTESIAN_POINT('Ctrl Pts',(-3.49086144065754,-24.7690239689578,18.3157672824377));
#4913=CARTESIAN_POINT('Ctrl Pts',(-4.25892622749306,-27.2963088098151,18.0865949609766));
#4914=CARTESIAN_POINT('Ctrl Pts',(-3.97209576034448,-28.7513998106872,17.9720465012551));
#4915=CARTESIAN_POINT('Ctrl Pts',(-2.27986640092468,-30.8159741693962,17.7428710328365));
#4916=CARTESIAN_POINT('Ctrl Pts',(-0.896246105632028,-31.3920385726492,
17.6283237739899));
#4917=CARTESIAN_POINT('Ctrl Pts',(1.11730059050837,-31.1951657997167,17.4564398922454));
#4918=CARTESIAN_POINT('Ctrl Pts',(1.77293796695974,-30.9607418032691,17.3991667053302));
#4919=CARTESIAN_POINT('Ctrl Pts',(2.90079609967118,-30.2083650352605,17.2845767099533));
#4920=CARTESIAN_POINT('Ctrl Pts',(3.37096147508705,-29.6899088375397,17.2273038101533));
#4921=CARTESIAN_POINT('Ctrl Pts',(4.01434027316612,-28.4885505800527,17.1127130864091));
#4922=CARTESIAN_POINT('Ctrl Pts',(4.18550422020648,-27.8061883428027,17.0554404695231));
#4923=CARTESIAN_POINT('Ctrl Pts',(4.18666372276521,-26.4363866453329,16.9408490296383));
#4924=CARTESIAN_POINT('Ctrl Pts',(4.01511368510023,-25.7504022482198,16.8835766915364));
#4925=CARTESIAN_POINT('Ctrl Pts',(3.36716919883249,-24.5355841608964,16.768984547513));
#4926=CARTESIAN_POINT('Ctrl Pts',(2.89011009304215,-24.0087701677114,16.7117124841267));
#4927=CARTESIAN_POINT('Ctrl Pts',(1.74021985056861,-23.238886159766,16.5971196477113));
#4928=CARTESIAN_POINT('Ctrl Pts',(1.06776929851019,-22.9979117452528,16.5398478550424));
#4929=CARTESIAN_POINT('Ctrl Pts',(-0.316234198911765,-22.8602379128138,
16.4252543377482));
#4930=CARTESIAN_POINT('Ctrl Pts',(-1.02645022638954,-22.9652013326477,16.367982811854));
#4931=CARTESIAN_POINT('Ctrl Pts',(-2.31843179248706,-23.4988220743056,16.253388624978));
#4932=CARTESIAN_POINT('Ctrl Pts',(-2.89822537783462,-23.9283042106777,16.1961173619753));
#4933=CARTESIAN_POINT('Ctrl Pts',(-3.7905997062367,-25.0133296018116,16.0815225165821));
#4934=CARTESIAN_POINT('Ctrl Pts',(-4.10104992194752,-25.6686564062324,16.0242515126585));
#4935=CARTESIAN_POINT('Ctrl Pts',(-4.37800508806418,-27.0530874546831,15.9096560195834));
#4936=CARTESIAN_POINT('Ctrl Pts',(-4.34273749797898,-27.7809826876019,15.8523852709862));
#4937=CARTESIAN_POINT('Ctrl Pts',(-3.93239882986814,-29.1392219832472,15.7377891408615));
#4938=CARTESIAN_POINT('Ctrl Pts',(-3.55634473018214,-29.7676541332304,15.6805186438933));
#4939=CARTESIAN_POINT('Ctrl Pts',(-2.5492770121493,-30.7770804996531,15.5659218871409));
#4940=CARTESIAN_POINT('Ctrl Pts',(-1.91831148386587,-31.1559210956849,15.5086516381582));
#4941=CARTESIAN_POINT('Ctrl Pts',(-0.547628959916488,-31.573519486645,15.3940542650064));
#4942=CARTESIAN_POINT('Ctrl Pts',(0.191016400673711,-31.6104034742754,15.3367842604237));
#4943=CARTESIAN_POINT('Ctrl Pts',(1.60358879266949,-31.3312492241601,15.2221862808907));
#4944=CARTESIAN_POINT('Ctrl Pts',(2.27567641937781,-31.0140726493341,15.1649165171817));
#4945=CARTESIAN_POINT('Ctrl Pts',(3.39531536611764,-30.0975999653541,15.0503179410969));
#4946=CARTESIAN_POINT('Ctrl Pts',(3.84070241423541,-29.4981801195554,14.9930484147904));
#4947=CARTESIAN_POINT('Ctrl Pts',(4.39884914324192,-28.1556793562174,14.8784492517891));
#4948=CARTESIAN_POINT('Ctrl Pts',(4.50964309606246,-27.4135236144109,14.8211799594654));
#4949=CARTESIAN_POINT('Ctrl Pts',(4.36840568370932,-25.9594577970506,14.7065802190078));
#4950=CARTESIAN_POINT('Ctrl Pts',(4.11508455775685,-25.249302056657,14.6493111573042));
#4951=CARTESIAN_POINT('Ctrl Pts',(3.30123891875162,-24.0276528305633,14.5347108486526));
#4952=CARTESIAN_POINT('Ctrl Pts',(2.74041622475651,-23.5183212604017,14.4774420142573));
#4953=CARTESIAN_POINT('Ctrl Pts',(1.44063674541817,-22.8212145167712,14.3628411465179));
#4954=CARTESIAN_POINT('Ctrl Pts',(0.702450078752852,-22.6354867309707,14.3055725361634));
#4955=CARTESIAN_POINT('Ctrl Pts',(-0.779470864376416,-22.6333483810052,
14.1909711182638));
#4956=CARTESIAN_POINT('Ctrl Pts',(-1.52154844380728,-22.818374057944,14.1337027287374));
#4957=CARTESIAN_POINT('Ctrl Pts',(-2.83569714701013,-23.5183126097129,14.0191007694346));
#4958=CARTESIAN_POINT('Ctrl Pts',(-3.40562223222298,-24.0336997915325,13.9618325975741));
#4959=CARTESIAN_POINT('Ctrl Pts',(-4.23858629184574,-25.2762676906016,13.8472301054612));
#4960=CARTESIAN_POINT('Ctrl Pts',(-4.49950738867518,-26.0028413547787,13.7899621481505));
#4961=CARTESIAN_POINT('Ctrl Pts',(-4.64911509855466,-27.4983084170412,13.6753591316644));
#4962=CARTESIAN_POINT('Ctrl Pts',(-4.53622502812489,-28.2656552357695,13.6180913858362));
#4963=CARTESIAN_POINT('Ctrl Pts',(-3.96057999480023,-29.6615541781397,13.5034878532506));
#4964=CARTESIAN_POINT('Ctrl Pts',(-3.49717393714537,-30.2879901076548,13.4462203158853));
#4965=CARTESIAN_POINT('Ctrl Pts',(-2.32610017744464,-31.2521897408003,13.3316162753254));
#4966=CARTESIAN_POINT('Ctrl Pts',(-1.61886914981746,-31.5877771356732,13.2743489434468));
#4967=CARTESIAN_POINT('Ctrl Pts',(-0.124697446388046,-31.8875036436721,
13.1597444028882));
#4968=CARTESIAN_POINT('Ctrl Pts',(0.660819053714784,-31.8499327965513,13.1024772735659));
#4969=CARTESIAN_POINT('Ctrl Pts',(2.12656588333675,-31.4079391163672,12.9878722408366));
#4970=CARTESIAN_POINT('Ctrl Pts',(2.80472419949459,-31.0026888381985,12.930605311186));
#4971=CARTESIAN_POINT('Ctrl Pts',(3.89403059754656,-29.9170242414328,12.8159997939693));
#4972=CARTESIAN_POINT('Ctrl Pts',(4.302956855015,-29.2368697089914,12.7587330611525));
#4973=CARTESIAN_POINT('Ctrl Pts',(4.75394274417405,-27.7592200986048,12.6441270669872));
#4974=CARTESIAN_POINT('Ctrl Pts',(4.79416745413243,-26.963014811935,12.5868605281998));
#4975=CARTESIAN_POINT('Ctrl Pts',(4.49402767155989,-25.4403756296546,12.4722540645109));
#4976=CARTESIAN_POINT('Ctrl Pts',(4.15266099256647,-24.7159549508694,12.4149877169943));
#4977=CARTESIAN_POINT('Ctrl Pts',(3.16579371231746,-23.509148841337,12.300380791043));
#4978=CARTESIAN_POINT('Ctrl Pts',(2.52037040990553,-23.0290170242085,12.2431146320838));
#4979=CARTESIAN_POINT('Ctrl Pts',(1.07470014648255,-22.427189586173,12.1285072510228));
#4980=CARTESIAN_POINT('Ctrl Pts',(0.275597034529758,-22.3074443737027,12.0712412779435));
#4981=CARTESIAN_POINT('Ctrl Pts',(-1.84867894646398,-22.5128054297831,11.9157398874122));
#4982=CARTESIAN_POINT('Ctrl Pts',(-3.12605493920518,-23.2393875058207,11.8175858794686));
#4983=CARTESIAN_POINT('Ctrl Pts',(-4.33212117789959,-24.8803929083851,11.670327340705));
#4984=CARTESIAN_POINT('Ctrl Pts',(-4.61676851210983,-25.5145964215772,11.621230586331));
#4985=CARTESIAN_POINT('Ctrl Pts',(-4.83249456580181,-26.5137516564125,11.5476061383012));
#4986=CARTESIAN_POINT('Ctrl Pts',(-4.86980233496674,-26.8545727381983,11.5230628470662));
#4987=CARTESIAN_POINT('Ctrl Pts',(-4.87149239663453,-27.5373948311151,11.4739642712348));
#4988=CARTESIAN_POINT('Ctrl Pts',(-4.8480514492971,-27.8775532073051,11.4494251587111));
#4989=CARTESIAN_POINT('Ctrl Pts',(-4.83318900376681,-28.2179631660451,11.424881036809));
#4990=CARTESIAN_POINT('Ctrl Pts',(-3.5,-27.2127225901214,22.4975166120351));
#4991=CARTESIAN_POINT('Ctrl Pts',(-3.49927785868713,-27.7853287709716,22.4402329481162));
#4992=CARTESIAN_POINT('Ctrl Pts',(-3.35446180200001,-28.3588230843844,22.3829524737063));
#4993=CARTESIAN_POINT('Ctrl Pts',(-2.53808767932955,-29.8821237915549,22.2111091898206));
#4994=CARTESIAN_POINT('Ctrl Pts',(-1.46145231937317,-30.6017446798008,22.0965431657326));
#4995=CARTESIAN_POINT('Ctrl Pts',(0.860002585417323,-30.8282120086964,21.8674139251703));
#4996=CARTESIAN_POINT('Ctrl Pts',(2.07107291079633,-30.3270227433741,21.752849624791));
#4997=CARTESIAN_POINT('Ctrl Pts',(3.56721541815537,-28.5011179635623,21.5237157036811));
#4998=CARTESIAN_POINT('Ctrl Pts',(3.82659931701312,-27.20036017698,21.4091530749885));
#4999=CARTESIAN_POINT('Ctrl Pts',(3.13180267166131,-24.9149469548,21.1800146464357));
#5000=CARTESIAN_POINT('Ctrl Pts',(2.18342706770339,-23.9653744387647,21.0654536391327));
#5001=CARTESIAN_POINT('Ctrl Pts',(-0.129625104573071,-23.2648849532031,
20.8363108683544));
#5002=CARTESIAN_POINT('Ctrl Pts',(-1.46147591168062,-23.5287326354126,20.7217514337973));
#5003=CARTESIAN_POINT('Ctrl Pts',(-3.35090502810569,-25.0803600405907,20.4926044785548));
#5004=CARTESIAN_POINT('Ctrl Pts',(-3.87764741849126,-26.3487475764667,20.3780465697071));
#5005=CARTESIAN_POINT('Ctrl Pts',(-3.63479848762931,-28.8097762988588,20.148895580705));
#5006=CARTESIAN_POINT('Ctrl Pts',(-2.86427039073957,-29.9655693350743,20.0343391520621));
#5007=CARTESIAN_POINT('Ctrl Pts',(-0.65846096708456,-31.1444434869326,19.8051842733852));
#5008=CARTESIAN_POINT('Ctrl Pts',(0.74630206229462,-31.1460905834951,19.6906292809279));
#5009=CARTESIAN_POINT('Ctrl Pts',(2.97689487550167,-29.9540126226856,19.4614706503338));
#5010=CARTESIAN_POINT('Ctrl Pts',(3.76757285952208,-28.7739850439139,19.3469170514958));
#5011=CARTESIAN_POINT('Ctrl Pts',(4.0187034886225,-26.2291205871072,19.1177548007802));
#5012=CARTESIAN_POINT('Ctrl Pts',(3.47099870281935,-24.9015607577697,19.0032025543658));
#5013=CARTESIAN_POINT('Ctrl Pts',(1.47303203265274,-23.2608624483575,18.7740368097113));
#5014=CARTESIAN_POINT('Ctrl Pts',(0.0495881203952384,-22.9754752873616,
18.6594858758451));
#5015=CARTESIAN_POINT('Ctrl Pts',(-2.45155713850874,-23.7330678076998,18.4303167580854));
#5016=CARTESIAN_POINT('Ctrl Pts',(-3.49087258075457,-24.7690158719264,18.3157670982032));
#5017=CARTESIAN_POINT('Ctrl Pts',(-4.25893999689643,-27.296309020853,18.0865947230583));
#5018=CARTESIAN_POINT('Ctrl Pts',(-3.97210868158914,-28.7514045749302,17.9720462998272));
#5019=CARTESIAN_POINT('Ctrl Pts',(-2.27987387495177,-30.8159857353485,17.7428707782702));
#5020=CARTESIAN_POINT('Ctrl Pts',(-0.896249322735714,-31.3920519629118,
17.6283235555406));
#5021=CARTESIAN_POINT('Ctrl Pts',(1.11730388459739,-31.1951786270721,17.4564396343434));
#5022=CARTESIAN_POINT('Ctrl Pts',(1.77294326754581,-30.9607539401843,17.3991664653485));
#5023=CARTESIAN_POINT('Ctrl Pts',(2.90080505154166,-30.2083747949576,17.2845764438015));
#5024=CARTESIAN_POINT('Ctrl Pts',(3.37097187102428,-29.6899170424932,17.2273035618313));
#5025=CARTESIAN_POINT('Ctrl Pts',(4.01435276857721,-28.4885549672909,17.1127128120475));
#5026=CARTESIAN_POINT('Ctrl Pts',(4.18551725625119,-27.8061906781911,17.0554402129015));
#5027=CARTESIAN_POINT('Ctrl Pts',(4.18667681067326,-26.4363846241478,16.9408487471063));
#5028=CARTESIAN_POINT('Ctrl Pts',(4.01512628257138,-25.7503981626563,16.8835764266556));
#5029=CARTESIAN_POINT('Ctrl Pts',(3.3671797883428,-24.5355762087865,16.7689842568497));
#5030=CARTESIAN_POINT('Ctrl Pts',(2.89011927690729,-24.0087606262116,16.7117122110268));
#5031=CARTESIAN_POINT('Ctrl Pts',(1.74022544089816,-23.2388741548863,16.5971193489555));
#5032=CARTESIAN_POINT('Ctrl Pts',(1.06777289997686,-22.997899001297,16.5398475737628));
#5033=CARTESIAN_POINT('Ctrl Pts',(-0.316234927853767,-22.8602246903861,
16.4252540309383));
#5034=CARTESIAN_POINT('Ctrl Pts',(-1.02645305770396,-22.9651883959601,16.3679825224341));
#5035=CARTESIAN_POINT('Ctrl Pts',(-2.31843866837204,-23.4988107570144,16.253388310152));
#5036=CARTESIAN_POINT('Ctrl Pts',(-2.89823397310667,-23.9282941364198,16.196117064454));
#5037=CARTESIAN_POINT('Ctrl Pts',(-3.79061110505536,-25.0133228623296,16.0815221937778));
#5038=CARTESIAN_POINT('Ctrl Pts',(-4.10106225113868,-25.6686515734845,16.0242512070742));
#5039=CARTESIAN_POINT('Ctrl Pts',(-4.37801831770041,-27.0530868844925,15.909655688838));
#5040=CARTESIAN_POINT('Ctrl Pts',(-4.34275064929299,-27.7809842375283,15.8523849573772));
#5041=CARTESIAN_POINT('Ctrl Pts',(-3.93241076591198,-29.1392277168195,15.7377888022123));
#5042=CARTESIAN_POINT('Ctrl Pts',(-3.55635559774948,-29.7676616996119,15.6805183222975));
#5043=CARTESIAN_POINT('Ctrl Pts',(-2.5492848357845,-30.7770911827345,15.5659215406245));
#5044=CARTESIAN_POINT('Ctrl Pts',(-1.91831750124282,-31.1559328914483,15.508651308613));
#5045=CARTESIAN_POINT('Ctrl Pts',(-0.547630823615979,-31.573532596127,15.3940539106591));
#5046=CARTESIAN_POINT('Ctrl Pts',(0.191016654419482,-31.6104167135759,15.3367839229662));
#5047=CARTESIAN_POINT('Ctrl Pts',(1.60359332885263,-31.3312616639846,15.2221859187487));
#5048=CARTESIAN_POINT('Ctrl Pts',(2.27568288412789,-31.0140842055001,15.1649161718489));
#5049=CARTESIAN_POINT('Ctrl Pts',(3.39532523069409,-30.0976087977106,15.0503175711959));
#5050=CARTESIAN_POINT('Ctrl Pts',(3.84071356306253,-29.4981872635055,14.9930480616187));
#5051=CARTESIAN_POINT('Ctrl Pts',(4.39886200638194,-28.1556824953451,14.8784488741645));
#5052=CARTESIAN_POINT('Ctrl Pts',(4.50965629588013,-27.4135246591517,14.821179598491));
#5053=CARTESIAN_POINT('Ctrl Pts',(4.36841850750692,-25.9594545017938,14.7065798336947));
#5054=CARTESIAN_POINT('Ctrl Pts',(4.11509669119356,-25.2492967556584,14.649310788563));
#5055=CARTESIAN_POINT('Ctrl Pts',(3.301248674694,-24.027643879362,14.5347104556859));
#5056=CARTESIAN_POINT('Ctrl Pts',(2.7404244263817,-23.5183108657722,14.4774416377848));
#5057=CARTESIAN_POINT('Ctrl Pts',(1.44064112961331,-22.8212020237703,14.3628407459321));
#5058=CARTESIAN_POINT('Ctrl Pts',(0.702452411780137,-22.6354736977066,14.3055721519949));
#5059=CARTESIAN_POINT('Ctrl Pts',(-0.779472887126354,-22.6333352967227,
14.190970710093));
#5060=CARTESIAN_POINT('Ctrl Pts',(-1.52155253015143,-22.8183614641083,14.1337023369077));
#5061=CARTESIAN_POINT('Ctrl Pts',(-2.83570509877543,-23.5183020242021,14.0191003537129));
#5062=CARTESIAN_POINT('Ctrl Pts',(-3.40563177267265,-24.0336906113064,13.9618321981179));
#5063=CARTESIAN_POINT('Ctrl Pts',(-4.23859829449245,-25.2762621036854,13.8472296822221));
#5064=CARTESIAN_POINT('Ctrl Pts',(-4.49952012993745,-26.0028377560707,13.7899617411021));
#5065=CARTESIAN_POINT('Ctrl Pts',(-4.64912831734354,-27.4983091479623,13.6753587009413));
#5066=CARTESIAN_POINT('Ctrl Pts',(-4.53623796107103,-28.2656580682614,13.6180909712297));
#5067=CARTESIAN_POINT('Ctrl Pts',(-3.96059130788698,-29.6615610540449,13.5034874150766));
#5068=CARTESIAN_POINT('Ctrl Pts',(-3.49718400748527,-30.2879987021829,13.4462198937543));
#5069=CARTESIAN_POINT('Ctrl Pts',(-2.32610691316009,-31.2522011376172,13.3316158297333));
#5070=CARTESIAN_POINT('Ctrl Pts',(-1.61887397941475,-31.5877894623157,13.2743485138248));
#5071=CARTESIAN_POINT('Ctrl Pts',(-0.124698014175552,-31.8875168697119,
13.1597439499104));
#5072=CARTESIAN_POINT('Ctrl Pts',(0.660820605236803,-31.8499459440715,13.1024768364861));
#5073=CARTESIAN_POINT('Ctrl Pts',(2.12657161732859,-31.4079510480467,12.9878717805055));
#5074=CARTESIAN_POINT('Ctrl Pts',(2.8047317654823,-31.0026997016065,12.9306048666812));
#5075=CARTESIAN_POINT('Ctrl Pts',(3.89404127890867,-29.9170320609718,12.8159993263168));
#5076=CARTESIAN_POINT('Ctrl Pts',(4.30296864843086,-29.2368757228388,12.7587326092554));
#5077=CARTESIAN_POINT('Ctrl Pts',(4.75395585015817,-27.7592219594744,12.6441265920449));
#5078=CARTESIAN_POINT('Ctrl Pts',(4.79418068964257,-26.9630145561609,12.5868600689426));
#5079=CARTESIAN_POINT('Ctrl Pts',(4.49404010690874,-25.4403710926243,12.4722535823103));
#5080=CARTESIAN_POINT('Ctrl Pts',(4.15267254437464,-24.7159484861244,12.4149872504092));
#5081=CARTESIAN_POINT('Ctrl Pts',(3.16580254027823,-23.5091389781496,12.3003803016153));
#5082=CARTESIAN_POINT('Ctrl Pts',(2.52037754996715,-23.0290058774741,12.2431141582025));
#5083=CARTESIAN_POINT('Ctrl Pts',(1.07470328235808,-22.427176726376,12.1285067543989));
#5084=CARTESIAN_POINT('Ctrl Pts',(0.275598076802496,-22.3074311776151,12.0712407967975));
#5085=CARTESIAN_POINT('Ctrl Pts',(-1.84868379116737,-22.5127927449768,11.9157393755432));
#5086=CARTESIAN_POINT('Ctrl Pts',(-3.12606319175256,-23.2393767520925,11.8175853786087));
#5087=CARTESIAN_POINT('Ctrl Pts',(-4.33213271301493,-24.880386526967,11.6703268381421));
#5088=CARTESIAN_POINT('Ctrl Pts',(-4.61678084393395,-25.5145917668544,11.6212300753262));
#5089=CARTESIAN_POINT('Ctrl Pts',(-4.8325074990541,-26.51374965466,11.547605629606));
#5090=CARTESIAN_POINT('Ctrl Pts',(-4.86981537831802,-26.8545716453141,11.5230623381901));
#5091=CARTESIAN_POINT('Ctrl Pts',(-4.87150546249911,-27.5373956033118,11.4739637523339));
#5092=CARTESIAN_POINT('Ctrl Pts',(-4.84806449389349,-27.8775537395237,11.4494246411902));
#5093=CARTESIAN_POINT('Ctrl Pts',(-4.8332020483632,-28.2179636982637,11.4248805192881));
#5094=CARTESIAN_POINT('Ctrl Pts',(-4.49992531496781,-27.2005618150104,22.4987331790167));
#5095=CARTESIAN_POINT('Ctrl Pts',(-4.50123266577206,-27.9399345555106,22.4403537839278));
#5096=CARTESIAN_POINT('Ctrl Pts',(-4.31885456358521,-28.6714666153785,22.3845992765752));
#5097=CARTESIAN_POINT('Ctrl Pts',(-3.27206873853112,-30.6387455869407,22.2092430694354));
#5098=CARTESIAN_POINT('Ctrl Pts',(-1.90301347052226,-31.5589454854703,22.0978648836455));
#5099=CARTESIAN_POINT('Ctrl Pts',(1.08133745456905,-31.8588483286696,21.8641055935273));
#5100=CARTESIAN_POINT('Ctrl Pts',(2.62163729847883,-31.2259625043182,21.7526920522415));
#5101=CARTESIAN_POINT('Ctrl Pts',(4.54712383673962,-28.889667640373,21.5189807362004));
#5102=CARTESIAN_POINT('Ctrl Pts',(4.87991725612086,-27.2420071964223,21.4075326300492));
#5103=CARTESIAN_POINT('Ctrl Pts',(3.99926793651637,-24.3160463481836,21.1738683059317));
#5104=CARTESIAN_POINT('Ctrl Pts',(2.80324492166405,-23.1127118024641,21.0623863989465));
#5105=CARTESIAN_POINT('Ctrl Pts',(-0.145664295624094,-22.2108911563125,
20.8287681139101));
#5106=CARTESIAN_POINT('Ctrl Pts',(-1.82608753442347,-22.5396643242445,20.7172531447498));
#5107=CARTESIAN_POINT('Ctrl Pts',(-4.23617685498116,-24.5081432429562,20.4836799735107));
#5108=CARTESIAN_POINT('Ctrl Pts',(-4.90258935139331,-26.1024197715759,20.3721326565532));
#5109=CARTESIAN_POINT('Ctrl Pts',(-4.60239401978947,-29.2279523583354,20.1386037010885));
#5110=CARTESIAN_POINT('Ctrl Pts',(-3.63850146388098,-30.6809230335259,20.0270247275001));
#5111=CARTESIAN_POINT('Ctrl Pts',(-0.848312218451317,-32.1812843569572,
19.7935391153079));
#5112=CARTESIAN_POINT('Ctrl Pts',(0.910962191510308,-32.187257662144,19.6819291541039));
#5113=CARTESIAN_POINT('Ctrl Pts',(3.73351916376344,-30.6878849222468,19.4484860378945));
#5114=CARTESIAN_POINT('Ctrl Pts',(4.72474370347859,-29.2155039993741,19.3368457367663));
#5115=CARTESIAN_POINT('Ctrl Pts',(5.04923349895883,-26.0077171480983,19.103444293163));
#5116=CARTESIAN_POINT('Ctrl Pts',(4.36986673206198,-24.3509968931086,18.9917742794446));
#5117=CARTESIAN_POINT('Ctrl Pts',(1.86145168328288,-22.2810150440159,18.7584137083719));
#5118=CARTESIAN_POINT('Ctrl Pts',(0.0911844603756664,-21.9222328729832,
18.6467145899854));
#5119=CARTESIAN_POINT('Ctrl Pts',(-3.05047794174479,-22.8657614168808,18.4133941133931));
#5120=CARTESIAN_POINT('Ctrl Pts',(-4.3434939460169,-24.1492993667947,18.3016664794364));
#5121=CARTESIAN_POINT('Ctrl Pts',(-5.31279863706187,-27.3124610697944,18.0683853413922));
#5122=CARTESIAN_POINT('Ctrl Pts',(-4.96105242549078,-29.116041915327,17.9566297629436));
#5123=CARTESIAN_POINT('Ctrl Pts',(-2.85190795720616,-31.7012004702625,17.7233872278977));
#5124=CARTESIAN_POINT('Ctrl Pts',(-1.14247440761136,-32.4168925823255,17.6116042590234));
#5125=CARTESIAN_POINT('Ctrl Pts',(1.36942113919458,-32.1769364386145,17.4367007733733));
#5126=CARTESIAN_POINT('Ctrl Pts',(2.17863030294074,-31.8896680393015,17.3807991645495));
#5127=CARTESIAN_POINT('Ctrl Pts',(3.58594774059714,-30.955345510934,17.2642061815091));
#5128=CARTESIAN_POINT('Ctrl Pts',(4.1666380278044,-30.3178934995088,17.2082979257248));
#5129=CARTESIAN_POINT('Ctrl Pts',(4.97070480320723,-28.8243377732163,17.0917141975888));
#5130=CARTESIAN_POINT('Ctrl Pts',(5.18324736692089,-27.9849325707496,17.0357993595099));
#5131=CARTESIAN_POINT('Ctrl Pts',(5.18837634682399,-26.2816906794162,16.9192248016874));
#5132=CARTESIAN_POINT('Ctrl Pts',(4.97928961288882,-25.4377044137181,16.8633034450976));
#5133=CARTESIAN_POINT('Ctrl Pts',(4.17766130573194,-23.9269514586941,16.7467379739209));
#5134=CARTESIAN_POINT('Ctrl Pts',(3.59301796923098,-23.2784899136664,16.6908101616495));
#5135=CARTESIAN_POINT('Ctrl Pts',(2.16808835767185,-22.3200655571735,16.5742536948244));
#5136=CARTESIAN_POINT('Ctrl Pts',(1.34341569002319,-22.0225242875423,16.5183194887516));
#5137=CARTESIAN_POINT('Ctrl Pts',(-0.37202542262785,-21.848229520912,16.4017719448942));
#5138=CARTESIAN_POINT('Ctrl Pts',(-1.2431512747268,-21.9750627042462,16.3458314060321));
#5139=CARTESIAN_POINT('Ctrl Pts',(-2.84469319036191,-22.6326276198057,16.2292927049662));
#5140=CARTESIAN_POINT('Ctrl Pts',(-3.55608395141779,-23.1572481132965,16.1733458934499));
#5141=CARTESIAN_POINT('Ctrl Pts',(-4.66303405570225,-24.4975081087771,16.0568159559262));
#5142=CARTESIAN_POINT('Ctrl Pts',(-5.0446924336988,-25.2987711172549,16.0008629310603));
#5143=CARTESIAN_POINT('Ctrl Pts',(-5.39056519898843,-27.0094466251327,15.8843416789414));
#5144=CARTESIAN_POINT('Ctrl Pts',(-5.34930304043553,-27.8996098051487,15.8283824991195));
#5145=CARTESIAN_POINT('Ctrl Pts',(-4.84595092330871,-29.5780539034839,15.7118698553524));
#5146=CARTESIAN_POINT('Ctrl Pts',(-4.38811855967175,-30.3467642405488,15.6559045781531));
#5147=CARTESIAN_POINT('Ctrl Pts',(-3.14807661476919,-31.5947342749175,15.5394004666024));
#5148=CARTESIAN_POINT('Ctrl Pts',(-2.37886502949379,-32.0587365058605,15.4834291488454));
#5149=CARTESIAN_POINT('Ctrl Pts',(-0.690271412805203,-32.5768833169426,
15.3669334943444));
#5150=CARTESIAN_POINT('Ctrl Pts',(0.210437406783647,-32.6237032613599,15.3109561919855));
#5151=CARTESIAN_POINT('Ctrl Pts',(1.95077582228988,-32.2833593081943,15.1944689204932));
#5152=CARTESIAN_POINT('Ctrl Pts',(2.77047067840731,-31.8985499371097,15.1384856887274));
#5153=CARTESIAN_POINT('Ctrl Pts',(4.15032302098314,-30.7736043375475,15.0220067269618));
#5154=CARTESIAN_POINT('Ctrl Pts',(4.69400309684405,-30.0449584837519,14.9660176202321));
#5155=CARTESIAN_POINT('Ctrl Pts',(5.38335863834062,-28.395939593178,14.8495468960155));
#5156=CARTESIAN_POINT('Ctrl Pts',(5.51992097583071,-27.4934852178884,14.7935519679768));
#5157=CARTESIAN_POINT('Ctrl Pts',(5.34990401728289,-25.7072478702335,14.6770894099612));
#5158=CARTESIAN_POINT('Ctrl Pts',(5.04374456081733,-24.8435781449226,14.6210887135337));
#5159=CARTESIAN_POINT('Ctrl Pts',(4.0479320191368,-23.342552408645,14.5046342513644));
#5160=CARTESIAN_POINT('Ctrl Pts',(3.36814614645295,-22.7227447945842,14.4486278387742));
#5161=CARTESIAN_POINT('Ctrl Pts',(1.77619102970885,-21.8650344590564,14.3321814028423));
#5162=CARTESIAN_POINT('Ctrl Pts',(0.881013595157293,-21.6379564042767,14.2761693255965));
#5163=CARTESIAN_POINT('Ctrl Pts',(-0.934286602741275,-21.631913240891,14.1597308473328));
#5164=CARTESIAN_POINT('Ctrl Pts',(-1.83430603011931,-21.85447637771,14.1037131561842));
#5165=CARTESIAN_POINT('Ctrl Pts',(-3.44430347736566,-22.7081266226923,13.9872825678333));
#5166=CARTESIAN_POINT('Ctrl Pts',(-4.13582211102842,-23.3310704412515,13.9312593128857));
#5167=CARTESIAN_POINT('Ctrl Pts',(-5.15723598600513,-24.8486604334571,13.8148365475172));
#5168=CARTESIAN_POINT('Ctrl Pts',(-5.47468869489397,-25.7274061109226,13.7588077782201));
#5169=CARTESIAN_POINT('Ctrl Pts',(-5.66084498304722,-27.5542511137055,13.6423927697258));
#5170=CARTESIAN_POINT('Ctrl Pts',(-5.52607729259019,-28.4824463986154,13.5863585348362));
#5171=CARTESIAN_POINT('Ctrl Pts',(-4.82645265952584,-30.1878171234494,13.4699512180057));
#5172=CARTESIAN_POINT('Ctrl Pts',(-4.26793016275464,-30.9457917464557,13.4139115656321));
#5173=CARTESIAN_POINT('Ctrl Pts',(-2.84163338331343,-32.1244708835282,13.2975118759857));
#5174=CARTESIAN_POINT('Ctrl Pts',(-1.98851329456531,-32.5312245863753,13.2414668535995));
#5175=CARTESIAN_POINT('Ctrl Pts',(-0.168154346495923,-32.8997884885716,
13.1250747275302));
#5176=CARTESIAN_POINT('Ctrl Pts',(0.779568298212397,-32.8562079727566,13.0690243819638));
#5177=CARTESIAN_POINT('Ctrl Pts',(2.56542990953642,-32.3211571768756,12.9526397565944));
#5178=CARTESIAN_POINT('Ctrl Pts',(3.38380416962575,-31.8341443288812,12.8965841340846));
#5179=CARTESIAN_POINT('Ctrl Pts',(4.71155278837089,-30.5155103343138,12.7802069473221));
#5180=CARTESIAN_POINT('Ctrl Pts',(5.20559259369133,-29.6971531119313,12.7241460934996));
#5181=CARTESIAN_POINT('Ctrl Pts',(5.75703886090729,-27.9016459598323,12.6077762839981));
#5182=CARTESIAN_POINT('Ctrl Pts',(5.80717713818053,-26.9434385648419,12.5517102438793));
#5183=CARTESIAN_POINT('Ctrl Pts',(5.44579520263474,-25.0931237590171,12.4353477510898));
#5184=CARTESIAN_POINT('Ctrl Pts',(5.0368047411671,-24.2211610859936,12.3792765691091));
#5185=CARTESIAN_POINT('Ctrl Pts',(3.84146164273372,-22.7542474974693,12.2629213331626));
#5186=CARTESIAN_POINT('Ctrl Pts',(3.06685116348872,-22.1758765063834,12.2068450531984));
#5187=CARTESIAN_POINT('Ctrl Pts',(1.3147114679644,-21.4429359570459,12.0904970149672));
#5188=CARTESIAN_POINT('Ctrl Pts',(0.355369734306315,-21.2974519808943,12.0344156803179));
#5189=CARTESIAN_POINT('Ctrl Pts',(-2.21947927012219,-21.541945111076,11.8765628382364));
#5190=CARTESIAN_POINT('Ctrl Pts',(-3.75768230547338,-22.4163266113853,11.7792514363029));
#5191=CARTESIAN_POINT('Ctrl Pts',(-5.21498730250992,-24.3919766537203,11.6318625545005));
#5192=CARTESIAN_POINT('Ctrl Pts',(-5.56061254440886,-25.1583366949337,11.5821196744937));
#5193=CARTESIAN_POINT('Ctrl Pts',(-5.82237026188237,-26.3605430038448,11.5086720015383));
#5194=CARTESIAN_POINT('Ctrl Pts',(-5.86810470583882,-26.7709263784967,11.4841148639085));
#5195=CARTESIAN_POINT('Ctrl Pts',(-5.87151787372438,-27.5964966533761,11.4342490225503));
#5196=CARTESIAN_POINT('Ctrl Pts',(-5.8464491178956,-27.9182877595946,11.4098155239949));
#5197=CARTESIAN_POINT('Ctrl Pts',(-5.83158667236532,-28.2586977183358,11.3852714020937));
#5198=CARTESIAN_POINT('Ctrl Pts',(-4.49992531496781,-27.1010184425723,21.5036999549465));
#5199=CARTESIAN_POINT('Ctrl Pts',(-4.51674600628465,-27.8405511731054,21.4453045543583));
#5200=CARTESIAN_POINT('Ctrl Pts',(-4.3513754570227,-28.5765453512511,21.3895276624965));
#5201=CARTESIAN_POINT('Ctrl Pts',(-3.34502119885618,-30.5657740901924,21.2141080231263));
#5202=CARTESIAN_POINT('Ctrl Pts',(-1.99683196222126,-31.5170666924607,21.1026952188504));
#5203=CARTESIAN_POINT('Ctrl Pts',(0.980993279522333,-31.8772272555485,20.8688610765165));
#5204=CARTESIAN_POINT('Ctrl Pts',(2.53490239289457,-31.2787547245274,20.7574094693259));
#5205=CARTESIAN_POINT('Ctrl Pts',(4.50569444399399,-28.9816631968142,20.5236326621716));
#5206=CARTESIAN_POINT('Ctrl Pts',(4.87413701918684,-27.3422265898772,20.41214314674));
#5207=CARTESIAN_POINT('Ctrl Pts',(4.05086560996824,-24.4015014064168,20.1784223463925));
#5208=CARTESIAN_POINT('Ctrl Pts',(2.88154677707693,-23.173754043832,20.0668957873436));
#5209=CARTESIAN_POINT('Ctrl Pts',(-0.0470467715653138,-22.2169532717186,
19.8332297105388));
#5210=CARTESIAN_POINT('Ctrl Pts',(-1.73235777827075,-22.5102673549153,19.7216669438178));
#5211=CARTESIAN_POINT('Ctrl Pts',(-4.17572182242301,-24.4312269013205,19.4880543497385));
#5212=CARTESIAN_POINT('Ctrl Pts',(-4.87376845888169,-26.0095620732211,19.3764561838128));
#5213=CARTESIAN_POINT('Ctrl Pts',(-4.6310120681261,-29.1353686231182,19.1428958730047));
#5214=CARTESIAN_POINT('Ctrl Pts',(-3.69789395427398,-30.6051559498652,19.0312630900414));
#5215=CARTESIAN_POINT('Ctrl Pts',(-0.939901316815822,-32.1524297385279,
18.797753901872));
#5216=CARTESIAN_POINT('Ctrl Pts',(0.815770716897848,-32.192946710534,18.6860872589115));
#5217=CARTESIAN_POINT('Ctrl Pts',(3.65834639903831,-30.746287086809,18.4526280705631));
#5218=CARTESIAN_POINT('Ctrl Pts',(4.67570856491877,-29.2962834910467,18.3409283004432));
#5219=CARTESIAN_POINT('Ctrl Pts',(5.05445235298275,-26.1019770515496,18.1075180249339));
#5220=CARTESIAN_POINT('Ctrl Pts',(4.40805306181254,-24.4365392522985,17.9957858373769));
#5221=CARTESIAN_POINT('Ctrl Pts',(1.94130016670179,-22.3299662886282,17.7624234222861));
#5222=CARTESIAN_POINT('Ctrl Pts',(0.182492857305352,-21.939377617945,17.6506595049407));
#5223=CARTESIAN_POINT('Ctrl Pts',(-2.96543044577777,-22.8282401952741,17.4173439305767));
#5224=CARTESIAN_POINT('Ctrl Pts',(-4.27794385851622,-24.0844995025642,17.3055489496951));
#5225=CARTESIAN_POINT('Ctrl Pts',(-5.29537653242634,-27.2218242153782,17.0722792286103));
#5226=CARTESIAN_POINT('Ctrl Pts',(-4.97689278167529,-29.0259395054587,16.9604538299531));
#5227=CARTESIAN_POINT('Ctrl Pts',(-2.91608530249191,-31.6357336752382,16.7272290046934));
#5228=CARTESIAN_POINT('Ctrl Pts',(-1.22497985084763,-32.3788890909175,16.6153738146158));
#5229=CARTESIAN_POINT('Ctrl Pts',(1.28145612063066,-32.1789932923933,16.4404881713498));
#5230=CARTESIAN_POINT('Ctrl Pts',(2.0927818601203,-31.9069109397873,16.3845495671917));
#5231=CARTESIAN_POINT('Ctrl Pts',(3.50922640420288,-30.9978632225545,16.2679699605668));
#5232=CARTESIAN_POINT('Ctrl Pts',(4.09881550944335,-30.3728309488599,16.2120241353908));
#5233=CARTESIAN_POINT('Ctrl Pts',(4.92262783581331,-28.8973868790768,16.0954552401651));
#5234=CARTESIAN_POINT('Ctrl Pts',(5.14877399302525,-28.064821040575,16.0395022670422));
#5235=CARTESIAN_POINT('Ctrl Pts',(5.17972192673461,-26.3684552205223,15.9229439741396));
#5236=CARTESIAN_POINT('Ctrl Pts',(4.98580796318786,-25.5242055246215,15.8669839251149));
#5237=CARTESIAN_POINT('Ctrl Pts',(4.21017429044416,-24.0075929294983,15.7504361268929));
#5238=CARTESIAN_POINT('Ctrl Pts',(3.63880072013838,-23.351872300329,15.6944690729279));
#5239=CARTESIAN_POINT('Ctrl Pts',(2.23413550967172,-22.3762507712042,15.5779316635816));
#5240=CARTESIAN_POINT('Ctrl Pts',(1.41781408360257,-22.0661561590653,15.5219576745624));
#5241=CARTESIAN_POINT('Ctrl Pts',(-0.2876678119969,-21.8672909533799,15.4054305496812));
#5242=CARTESIAN_POINT('Ctrl Pts',(-1.15723576718454,-21.9791742088117,15.349449694498));
#5243=CARTESIAN_POINT('Ctrl Pts',(-2.76133682475571,-22.6104139372597,15.2329327513282));
#5244=CARTESIAN_POINT('Ctrl Pts',(-3.47827719059933,-23.1211141138698,15.1769450978676));
#5245=CARTESIAN_POINT('Ctrl Pts',(-4.59966549973914,-24.4392847330131,15.0604382350449));
#5246=CARTESIAN_POINT('Ctrl Pts',(-4.99267244674646,-25.2308278340738,15.0044438502435));
#5247=CARTESIAN_POINT('Ctrl Pts',(-5.36152867501004,-26.9286517721488,14.8879469679338));
#5248=CARTESIAN_POINT('Ctrl Pts',(-5.33479062947237,-27.815489816777,14.8319459176988));
#5249=CARTESIAN_POINT('Ctrl Pts',(-4.85770689425811,-29.4932029850683,14.7154589175941));
#5250=CARTESIAN_POINT('Ctrl Pts',(-4.41424130928336,-30.2657064039853,14.6594512668976));
#5251=CARTESIAN_POINT('Ctrl Pts',(-3.19776731478627,-31.5251842790945,14.5429740520141));
#5252=CARTESIAN_POINT('Ctrl Pts',(-2.43948640778453,-31.9991936236663,14.4869598649523));
#5253=CARTESIAN_POINT('Ctrl Pts',(-0.76641117646687,-32.538424291025,14.3704923396933));
#5254=CARTESIAN_POINT('Ctrl Pts',(0.129280639488567,-32.5991484080323,14.3144716793848));
#5255=CARTESIAN_POINT('Ctrl Pts',(1.86565117755554,-32.2846351962422,14.1980137496642));
#5256=CARTESIAN_POINT('Ctrl Pts',(2.6873584363981,-31.9144328140864,14.1419866783607));
#5257=CARTESIAN_POINT('Ctrl Pts',(4.0756575425974,-30.8141731242952,14.025538251239));
#5258=CARTESIAN_POINT('Ctrl Pts',(4.62788574697171,-30.0974982118229,13.9695048303297));
#5259=CARTESIAN_POINT('Ctrl Pts',(5.33614212196108,-28.4664074366612,13.8530658143517));
#5260=CARTESIAN_POINT('Ctrl Pts',(5.48580553915912,-27.5705664905401,13.7970261043234));
#5261=CARTESIAN_POINT('Ctrl Pts',(5.34081184824442,-25.791439376031,13.6805964092432));
#5262=CARTESIAN_POINT('Ctrl Pts',(5.04929361698828,-24.927539264489,13.6245504697451));
#5263=CARTESIAN_POINT('Ctrl Pts',(4.07891464172889,-23.4212168574546,13.5081300066553));
#5264=CARTESIAN_POINT('Ctrl Pts',(3.41195903484832,-22.794417393971,13.4520778965404));
#5265=CARTESIAN_POINT('Ctrl Pts',(1.84005664325852,-21.9202404356125,13.3356665776424));
#5266=CARTESIAN_POINT('Ctrl Pts',(0.952974962988242,-21.6810345955686,13.2796083549412));
#5267=CARTESIAN_POINT('Ctrl Pts',(-0.852207019879878,-21.6511301665541,
13.1632060938123));
#5268=CARTESIAN_POINT('Ctrl Pts',(-1.75069597922114,-21.8592211322789,13.1071418157038));
#5269=CARTESIAN_POINT('Ctrl Pts',(-3.36279321619093,-22.687065563139,12.9907485270725));
#5270=CARTESIAN_POINT('Ctrl Pts',(-4.0596712085529,-23.2965088909024,12.9346782499817));
#5271=CARTESIAN_POINT('Ctrl Pts',(-5.09490115062812,-24.7922309126811,12.8182938497412));
#5272=CARTESIAN_POINT('Ctrl Pts',(-5.42335290963779,-25.6615296657728,12.7622176293468));
#5273=CARTESIAN_POINT('Ctrl Pts',(-5.6318733184926,-27.4754205110425,12.6458420345123));
#5274=CARTESIAN_POINT('Ctrl Pts',(-5.51121048465282,-28.4003675711241,12.5897599257099));
#5275=CARTESIAN_POINT('Ctrl Pts',(-4.83738798718038,-30.1046366902265,12.4733930545196));
#5276=CARTESIAN_POINT('Ctrl Pts',(-4.29284127804266,-30.8662836546237,12.4173051114547));
#5277=CARTESIAN_POINT('Ctrl Pts',(-2.88989812922953,-32.0559489908963,12.3009468831881));
#5278=CARTESIAN_POINT('Ctrl Pts',(-2.04742969825749,-32.4724339533943,12.244853159285));
#5279=CARTESIAN_POINT('Ctrl Pts',(-0.2426536662203,-32.8615528897918,12.1285034943741));
#5280=CARTESIAN_POINT('Ctrl Pts',(0.700167228706349,-32.8315189484388,12.0724040423241));
#5281=CARTESIAN_POINT('Ctrl Pts',(2.48176316317964,-32.3218947112272,11.9560628622509));
#5282=CARTESIAN_POINT('Ctrl Pts',(3.30209026051788,-31.8491345603716,11.8999577340539));
#5283=CARTESIAN_POINT('Ctrl Pts',(4.63785467742761,-30.5549942620067,11.7836249613568));
#5284=CARTESIAN_POINT('Ctrl Pts',(5.14023670521377,-29.7483336343732,11.7275142083257));
#5285=CARTESIAN_POINT('Ctrl Pts',(5.71014369190083,-27.9707987230122,11.6111897665715));
#5286=CARTESIAN_POINT('Ctrl Pts',(5.77308874181379,-27.0190622633568,11.5550734393245));
#5287=CARTESIAN_POINT('Ctrl Pts',(5.43639437006847,-25.1760989492496,11.4387572531387));
#5288=CARTESIAN_POINT('Ctrl Pts',(5.04173404968112,-24.3039132848956,11.3826354016244));
#5289=CARTESIAN_POINT('Ctrl Pts',(3.87166745943498,-22.8320547671859,11.2663273965984));
#5290=CARTESIAN_POINT('Ctrl Pts',(3.10962740498996,-22.2468328201306,11.2102000701237));
#5291=CARTESIAN_POINT('Ctrl Pts',(1.3775808247441,-21.4977812085784,11.0939001728392));
#5292=CARTESIAN_POINT('Ctrl Pts',(0.426176004646674,-21.3404003073863,11.0377674200549));
#5293=CARTESIAN_POINT('Ctrl Pts',(-2.13467139062884,-21.5528754416251,10.8799811119317));
#5294=CARTESIAN_POINT('Ctrl Pts',(-3.67375330512296,-22.4019087871921,10.7826247286485));
#5295=CARTESIAN_POINT('Ctrl Pts',(-5.14572845587871,-24.3467779409998,10.6352234649416));
#5296=CARTESIAN_POINT('Ctrl Pts',(-5.4980087978572,-25.10396329861,10.585497622957));
#5297=CARTESIAN_POINT('Ctrl Pts',(-5.77284291612865,-26.2950238657267,10.5120341100286));
#5298=CARTESIAN_POINT('Ctrl Pts',(-5.82326382778836,-26.7021580375338,10.4874753114238));
#5299=CARTESIAN_POINT('Ctrl Pts',(-5.83613711196663,-27.5221379313639,10.4376301541696));
#5300=CARTESIAN_POINT('Ctrl Pts',(-5.80990657648216,-27.8448337026384,10.4131866340964));
#5301=CARTESIAN_POINT('Ctrl Pts',(-5.79504413095202,-28.1852436613808,10.3886425121934));
#5302=CARTESIAN_POINT('Ctrl Pts',(-3.5,-27.1131792176833,21.5024833879649));
#5303=CARTESIAN_POINT('Ctrl Pts',(-3.51479119919922,-27.6859453885664,21.4451837185487));
#5304=CARTESIAN_POINT('Ctrl Pts',(-3.3869826954375,-28.2639018202575,21.3878808596267));
#5305=CARTESIAN_POINT('Ctrl Pts',(-2.61104013965461,-29.8091522948055,21.2159741435134));
#5306=CARTESIAN_POINT('Ctrl Pts',(-1.55527081107218,-30.5598658867912,21.1013735009366));
#5307=CARTESIAN_POINT('Ctrl Pts',(0.7596584103706,-30.8465909355752,20.8721694081605));
#5308=CARTESIAN_POINT('Ctrl Pts',(1.98433800521209,-30.3798149635844,20.7575670418755));
#5309=CARTESIAN_POINT('Ctrl Pts',(3.52578602540974,-28.5931135200025,20.5283676296524));
#5310=CARTESIAN_POINT('Ctrl Pts',(3.8208190800791,-27.3005795704328,20.4137635916772));
#5311=CARTESIAN_POINT('Ctrl Pts',(3.18340034511317,-25.0004020130352,20.1845686868986));
#5312=CARTESIAN_POINT('Ctrl Pts',(2.26172892311522,-24.0264166801336,20.0699630275308));
#5313=CARTESIAN_POINT('Ctrl Pts',(-0.0310075805132356,-23.2709470686081,
19.840772464982));
#5314=CARTESIAN_POINT('Ctrl Pts',(-1.36774615552683,-23.4993356660845,19.7261652328664));
#5315=CARTESIAN_POINT('Ctrl Pts',(-3.29044999554861,-25.003443698954,19.4969788547815));
#5316=CARTESIAN_POINT('Ctrl Pts',(-3.84882652597964,-26.255889878113,19.3823700969656));
#5317=CARTESIAN_POINT('Ctrl Pts',(-3.66341653596594,-28.7171925636406,19.1531877526223));
#5318=CARTESIAN_POINT('Ctrl Pts',(-2.92366288113256,-29.8898022514147,19.0385775146034));
#5319=CARTESIAN_POINT('Ctrl Pts',(-0.750050065449063,-31.1155888685023,
18.8093990599493));
#5320=CARTESIAN_POINT('Ctrl Pts',(0.651110587682156,-31.1517796318851,18.6947873857344));
#5321=CARTESIAN_POINT('Ctrl Pts',(2.90172211077653,-30.0124147872479,18.4656126830036));
#5322=CARTESIAN_POINT('Ctrl Pts',(3.71853772096227,-28.8547645355866,18.3509996151738));
#5323=CARTESIAN_POINT('Ctrl Pts',(4.02392234264642,-26.3233804905586,18.1218285325501));
#5324=CARTESIAN_POINT('Ctrl Pts',(3.50918503257104,-24.9871031169595,18.0072141122992));
#5325=CARTESIAN_POINT('Ctrl Pts',(1.55288051607053,-23.3098136929698,17.7780465236243));
#5326=CARTESIAN_POINT('Ctrl Pts',(0.140896517323791,-22.9926200323223,17.6634307908027));
#5327=CARTESIAN_POINT('Ctrl Pts',(-2.36650964254058,-23.6955465860942,17.4342665752667));
#5328=CARTESIAN_POINT('Ctrl Pts',(-3.42532249325332,-24.7042160076948,17.319649568463));
#5329=CARTESIAN_POINT('Ctrl Pts',(-4.24151789226149,-27.205672166438,17.0904886102752));
#5330=CARTESIAN_POINT('Ctrl Pts',(-3.98794903777075,-28.6613021650618,16.9758703668355));
#5331=CARTESIAN_POINT('Ctrl Pts',(-2.34405122024042,-30.7505189403242,16.7467125550671));
#5332=CARTESIAN_POINT('Ctrl Pts',(-0.978754765971974,-31.3540484715026,
16.6320931111307));
#5333=CARTESIAN_POINT('Ctrl Pts',(1.02933886603348,-31.1972354808515,16.460227032321));
#5334=CARTESIAN_POINT('Ctrl Pts',(1.68709482472537,-30.9779968406706,16.4029168679907));
#5335=CARTESIAN_POINT('Ctrl Pts',(2.8240837151474,-30.2508925065775,16.2883402228593));
#5336=CARTESIAN_POINT('Ctrl Pts',(3.30314935266293,-29.7448544918448,16.2310297714992));
#5337=CARTESIAN_POINT('Ctrl Pts',(3.96627580118359,-28.5616040731508,16.116453854622));
#5338=CARTESIAN_POINT('Ctrl Pts',(4.15104388235541,-27.8860791480164,16.0591431204344));
#5339=CARTESIAN_POINT('Ctrl Pts',(4.17802239058402,-26.5231491652539,15.9445679195579));
#5340=CARTESIAN_POINT('Ctrl Pts',(4.02164463287101,-25.836899273559,15.8872569066736));
#5341=CARTESIAN_POINT('Ctrl Pts',(3.39969277305442,-24.6162176795914,15.7726824098211));
#5342=CARTESIAN_POINT('Ctrl Pts',(2.9359020278153,-24.0821430128742,15.7153711223063));
#5343=CARTESIAN_POINT('Ctrl Pts',(1.80627259289743,-23.295059368917,15.6007973177115));
#5344=CARTESIAN_POINT('Ctrl Pts',(1.14217129355625,-23.0415308728188,15.5434857595736));
#5345=CARTESIAN_POINT('Ctrl Pts',(-0.231877317222814,-22.8792861228552,
15.4289126357253));
#5346=CARTESIAN_POINT('Ctrl Pts',(-0.940537550161687,-22.9692999005262,
15.3716008109));
#5347=CARTESIAN_POINT('Ctrl Pts',(-2.23508230276584,-23.4765970744679,15.2570283565139));
#5348=CARTESIAN_POINT('Ctrl Pts',(-2.82042721228882,-23.8921601369938,15.1997162688729));
#5349=CARTESIAN_POINT('Ctrl Pts',(-3.72724254909164,-24.9550994865649,15.0851444728953));
#5350=CARTESIAN_POINT('Ctrl Pts',(-4.04904226418634,-25.6007082903028,15.0278321262568));
#5351=CARTESIAN_POINT('Ctrl Pts',(-4.34898179372202,-26.9722920315092,14.913260977831));
#5352=CARTESIAN_POINT('Ctrl Pts',(-4.32823823833014,-27.696864249156,14.8559483759565));
#5353=CARTESIAN_POINT('Ctrl Pts',(-3.94416673686108,-29.0543767984046,14.741377864454));
#5354=CARTESIAN_POINT('Ctrl Pts',(-3.58247834736109,-29.6866038630478,14.684065011041));
#5355=CARTESIAN_POINT('Ctrl Pts',(-2.59897553580158,-30.7075411869121,14.5694951260371));
#5356=CARTESIAN_POINT('Ctrl Pts',(-1.97893887953295,-31.0963900092535,14.5121820247212));
#5357=CARTESIAN_POINT('Ctrl Pts',(-0.62377058727827,-31.5350735702099,14.3976127560067));
#5358=CARTESIAN_POINT('Ctrl Pts',(0.109859887125028,-31.5858618602476,14.3402994103674));
#5359=CARTESIAN_POINT('Ctrl Pts',(1.51846868411767,-31.3325375520331,14.2257307479178));
#5360=CARTESIAN_POINT('Ctrl Pts',(2.19257064211805,-31.0299670824768,14.1684171614822));
#5361=CARTESIAN_POINT('Ctrl Pts',(3.32065975230898,-30.1381775844584,14.0538490954731));
#5362=CARTESIAN_POINT('Ctrl Pts',(3.77459621319051,-29.5507269915758,13.9965352717156));
#5363=CARTESIAN_POINT('Ctrl Pts',(4.35164549000208,-28.2261503388289,13.8819677925012));
#5364=CARTESIAN_POINT('Ctrl Pts',(4.47554085920862,-27.4906059318028,13.8246537348364));
#5365=CARTESIAN_POINT('Ctrl Pts',(4.35932633846837,-26.043646007592,13.7100868329779));
#5366=CARTESIAN_POINT('Ctrl Pts',(4.1206457473642,-25.3332578752253,13.6527725447744));
#5367=CARTESIAN_POINT('Ctrl Pts',(3.33223129728641,-24.106308328171,13.5382062109767));
#5368=CARTESIAN_POINT('Ctrl Pts',(2.78423731477771,-23.5899834651597,13.4808916955503));
#5369=CARTESIAN_POINT('Ctrl Pts',(1.50450674316234,-22.8764080003258,13.3663259207328));
#5370=CARTESIAN_POINT('Ctrl Pts',(0.774413779611081,-22.6785518889991,13.309011181339));
#5371=CARTESIAN_POINT('Ctrl Pts',(-0.69739330426496,-22.6525522223851,13.1944459565731));
#5372=CARTESIAN_POINT('Ctrl Pts',(-1.43794247925327,-22.8231062186778,13.1371309964266));
#5373=CARTESIAN_POINT('Ctrl Pts',(-2.7541948376007,-23.4972409646481,13.0225663129528));
#5374=CARTESIAN_POINT('Ctrl Pts',(-3.32948087019843,-23.9991290609593,12.9652511352145));
#5375=CARTESIAN_POINT('Ctrl Pts',(-4.17626345911414,-25.2198325829076,12.8506869844455));
#5376=CARTESIAN_POINT('Ctrl Pts',(-4.4481843446811,-25.936961310921,12.7933715922294));
#5377=CARTESIAN_POINT('Ctrl Pts',(-4.62015665278908,-27.4194785452993,12.6788079657272));
#5378=CARTESIAN_POINT('Ctrl Pts',(-4.52137115313415,-28.183579240772,12.621492362104));
#5379=CARTESIAN_POINT('Ctrl Pts',(-3.97152663554103,-29.5783806208201,12.5069292515898));
#5380=CARTESIAN_POINT('Ctrl Pts',(-3.5220951227733,-30.2084906103522,12.4496134395774));
#5381=CARTESIAN_POINT('Ctrl Pts',(-2.37437165907619,-31.183679244984,12.3350508369351));
#5382=CARTESIAN_POINT('Ctrl Pts',(-1.67779038310627,-31.5289988293348,12.277734819509));
#5383=CARTESIAN_POINT('Ctrl Pts',(-0.199197333900588,-31.8492812709321,
12.1631727167557));
#5384=CARTESIAN_POINT('Ctrl Pts',(0.581419535730091,-31.825256919753,12.1058564968451));
#5385=CARTESIAN_POINT('Ctrl Pts',(2.04290487097247,-31.4086885823989,11.9912948861633));
#5386=CARTESIAN_POINT('Ctrl Pts',(2.72301785637377,-31.017689933097,11.9339784666505));
#5387=CARTESIAN_POINT('Ctrl Pts',(3.82034316796606,-29.9565159886648,11.8194173403514));
#5388=CARTESIAN_POINT('Ctrl Pts',(4.23761275995296,-29.2880562452814,11.7621007240815));
#5389=CARTESIAN_POINT('Ctrl Pts',(4.70706068115205,-27.8283747226536,11.6475400746183));
#5390=CARTESIAN_POINT('Ctrl Pts',(4.76009229327592,-27.0386382546772,11.5902232643864));
#5391=CARTESIAN_POINT('Ctrl Pts',(4.48463927434238,-25.5233462828554,11.4756630843606));
#5392=CARTESIAN_POINT('Ctrl Pts',(4.15760185288866,-24.7987006850272,11.4183460829245));
#5393=CARTESIAN_POINT('Ctrl Pts',(3.19600835697949,-23.5869462478655,11.3037863650511));
#5394=CARTESIAN_POINT('Ctrl Pts',(2.56315379146772,-23.099962191222,11.2464691751292));
#5395=CARTESIAN_POINT('Ctrl Pts',(1.13757263913847,-22.4820219779078,11.1319099122695));
#5396=CARTESIAN_POINT('Ctrl Pts',(0.346404347142174,-22.3503795041057,11.0745925365344));
#5397=CARTESIAN_POINT('Ctrl Pts',(-1.76387591167285,-22.5237230755283,10.9191576492385));
#5398=CARTESIAN_POINT('Ctrl Pts',(-3.04213419140331,-23.2249589278969,10.8209586709532));
#5399=CARTESIAN_POINT('Ctrl Pts',(-4.26287386638314,-24.8351878142477,10.6736877485838));
#5400=CARTESIAN_POINT('Ctrl Pts',(-4.55417709738229,-25.4602183705301,10.6246080237907));
#5401=CARTESIAN_POINT('Ctrl Pts',(-4.78298015330037,-26.4482305165422,10.5509677380958));
#5402=CARTESIAN_POINT('Ctrl Pts',(-4.82497450026767,-26.7858033043513,10.5264227857054));
#5403=CARTESIAN_POINT('Ctrl Pts',(-4.83612470074125,-27.4630368812996,10.4773448839533));
#5404=CARTESIAN_POINT('Ctrl Pts',(-4.81152195248019,-27.8040996825675,10.4527957512917));
#5405=CARTESIAN_POINT('Ctrl Pts',(-4.7966595069499,-28.1445096413087,10.4282516293878));
#5406=CARTESIAN_POINT('Ctrl Pts',(-2.5001922552825,-27.1253385629422,21.501266964026));
#5407=CARTESIAN_POINT('Ctrl Pts',(-2.51295420098982,-27.5313577824259,21.4450628969469));
#5408=CARTESIAN_POINT('Ctrl Pts',(-2.42270332621939,-27.9512950495876,21.3862342503864));
#5409=CARTESIAN_POINT('Ctrl Pts',(-1.87714538123526,-29.0526194622768,21.2178400444839));
#5410=CARTESIAN_POINT('Ctrl Pts',(-1.11376157825568,-29.6027776278656,21.100051938429));
#5411=CARTESIAN_POINT('Ctrl Pts',(0.538349565558472,-29.8160757968226,20.8754773508141));
#5412=CARTESIAN_POINT('Ctrl Pts',(1.43383835235719,-29.480980899108,20.7577245958979));
#5413=CARTESIAN_POINT('Ctrl Pts',(2.54599282350851,-28.2046095284856,20.5331020404002));
#5414=CARTESIAN_POINT('Ctrl Pts',(2.76762498907472,-27.2589374478045,20.4153838460841));
#5415=CARTESIAN_POINT('Ctrl Pts',(2.31603707598399,-25.5992322015002,20.190714304724));
#5416=CARTESIAN_POINT('Ctrl Pts',(1.64198394673661,-24.878979061188,20.073029907075));
#5417=CARTESIAN_POINT('Ctrl Pts',(-0.0149702753337169,-24.3248169379275,
19.8483143325555));
#5418=CARTESIAN_POINT('Ctrl Pts',(-1.00317740346447,-24.4882876835594,19.7306629930104));
#5419=CARTESIAN_POINT('Ctrl Pts',(-2.4052822580784,-25.5755932158904,19.5059023104899));
#5420=CARTESIAN_POINT('Ctrl Pts',(-2.82400510475762,-26.5021887200201,19.3882833147663));
#5421=CARTESIAN_POINT('Ctrl Pts',(-2.69593477275153,-28.2990656728991,19.1634784221306));
#5422=CARTESIAN_POINT('Ctrl Pts',(-2.14952284133105,-29.1745326635594,19.0458910791425));
#5423=CARTESIAN_POINT('Ctrl Pts',(-0.560221136608609,-30.0788699092222,
18.8210428488002));
#5424=CARTESIAN_POINT('Ctrl Pts',(0.486469819045022,-30.1107349726532,18.7034864896048));
#5425=CARTESIAN_POINT('Ctrl Pts',(2.14518678566594,-29.2786287756811,18.4785957687259));
#5426=CARTESIAN_POINT('Ctrl Pts',(2.76147942022677,-28.4132974934977,18.361069745729));
#5427=CARTESIAN_POINT('Ctrl Pts',(2.99351350103085,-26.5447578971656,18.1361373575506));
#5428=CARTESIAN_POINT('Ctrl Pts',(2.61042269136205,-25.5376022468545,18.0186410434961));
#5429=CARTESIAN_POINT('Ctrl Pts',(1.1645065354457,-24.2895458878023,17.7936677880135));
#5430=CARTESIAN_POINT('Ctrl Pts',(0.0993050681995977,-24.0457386074764,
17.6762005750292));
#5431=CARTESIAN_POINT('Ctrl Pts',(-1.76765925983151,-24.5627509998687,17.4511872302086));
#5432=CARTESIAN_POINT('Ctrl Pts',(-2.57280137838496,-25.3238596471586,17.3337485292939));
#5433=CARTESIAN_POINT('Ctrl Pts',(-3.18778316377509,-27.1895220166399,17.1086958508986));
#5434=CARTESIAN_POINT('Ctrl Pts',(-2.99912157291404,-28.2967076983704,16.9912850910565));
#5435=CARTESIAN_POINT('Ctrl Pts',(-1.77208439720242,-29.8654082881016,16.7661938145838));
#5436=CARTESIAN_POINT('Ctrl Pts',(-0.732558632003384,-30.3293283518554,
16.6488104418068));
#5437=CARTESIAN_POINT('Ctrl Pts',(0.777251255138965,-30.2155931034426,16.4799635724161));
#5438=CARTESIAN_POINT('Ctrl Pts',(1.28145548961924,-30.0491919623743,16.4212820091803));
#5439=CARTESIAN_POINT('Ctrl Pts',(2.13902158450589,-29.5040096186941,16.308708090036));
#5440=CARTESIAN_POINT('Ctrl Pts',(2.5075767495388,-29.1169518716936,16.2500331729432));
#5441=CARTESIAN_POINT('Ctrl Pts',(3.01003621350007,-28.225860748242,16.1374500000821));
#5442=CARTESIAN_POINT('Ctrl Pts',(3.15343108382589,-27.7073582717565,16.078781664474));
#5443=CARTESIAN_POINT('Ctrl Pts',(3.17644063329496,-26.6778249212213,15.9661893224535));
#5444=CARTESIAN_POINT('Ctrl Pts',(3.05759466794496,-26.1495562562684,15.9075275045547));
#5445=CARTESIAN_POINT('Ctrl Pts',(2.58930655129671,-25.2247708681756,15.7949260770529));
#5446=CARTESIAN_POINT('Ctrl Pts',(2.23308598163984,-24.8123278608962,15.7362707140421));
#5447=CARTESIAN_POINT('Ctrl Pts',(1.37845998383059,-24.2137599340046,15.6236602833198));
#5448=CARTESIAN_POINT('Ctrl Pts',(0.866560913322279,-24.0167909029579,15.5650113133335));
#5449=CARTESIAN_POINT('Ctrl Pts',(-0.176093382241082,-23.8911623029184,
15.4523919607684));
#5450=CARTESIAN_POINT('Ctrl Pts',(-0.723864812305373,-23.9593091742205,
15.3937493227952));
#5451=CARTESIAN_POINT('Ctrl Pts',(-1.7088896572731,-24.3426783667014,15.2811211285617));
#5452=CARTESIAN_POINT('Ctrl Pts',(-2.16265458334177,-24.6631155012729,15.222484762466));
#5453=CARTESIAN_POINT('Ctrl Pts',(-2.85492217708992,-25.4708535911175,15.1098478058101));
#5454=CARTESIAN_POINT('Ctrl Pts',(-3.10552303274938,-25.9705452563459,15.0512176522992));
#5455=CARTESIAN_POINT('Ctrl Pts',(-3.33655396671587,-27.0159271596902,14.9385720113314));
#5456=CARTESIAN_POINT('Ctrl Pts',(-3.32180419664342,-27.5782526294144,14.8799480120284));
#5457=CARTESIAN_POINT('Ctrl Pts',(-3.03073399263118,-28.615602208499,14.7672937637892));
#5458=CARTESIAN_POINT('Ctrl Pts',(-2.7508131833225,-29.1075694124263,14.7086758611242));
#5459=CARTESIAN_POINT('Ctrl Pts',(-2.00025416217446,-29.8899942324127,14.5960130817379));
#5460=CARTESIAN_POINT('Ctrl Pts',(-1.51844550201379,-30.1936925456155,14.5374012188929));
#5461=CARTESIAN_POINT('Ctrl Pts',(-0.481146769632026,-30.5318408224011,
14.4247299835279));
#5462=CARTESIAN_POINT('Ctrl Pts',(0.0904414182347455,-30.572694453714,14.3661241045503));
#5463=CARTESIAN_POINT('Ctrl Pts',(1.1713270120612,-30.3805518545432,14.2534444872335));
#5464=CARTESIAN_POINT('Ctrl Pts',(1.69784102450774,-30.1456053454915,14.194844536933));
#5465=CARTESIAN_POINT('Ctrl Pts',(2.56575073392967,-29.4622615275225,14.0821566109456));
#5466=CARTESIAN_POINT('Ctrl Pts',(2.92140700836645,-29.0040200601594,14.0235625348885));
#5467=CARTESIAN_POINT('Ctrl Pts',(3.36726461420379,-27.9859214901936,13.9108663723842));
#5468=CARTESIAN_POINT('Ctrl Pts',(3.46539496520096,-27.4106547747507,13.8522781169193));
#5469=CARTESIAN_POINT('Ctrl Pts',(3.37795623080819,-26.2958229849414,13.7395737892572));
#5470=CARTESIAN_POINT('Ctrl Pts',(3.19210706725742,-25.7389287819603,13.6809913014795));
#5471=CARTESIAN_POINT('Ctrl Pts',(2.58563574714856,-24.7913192464956,13.5682788789672));
#5472=CARTESIAN_POINT('Ctrl Pts',(2.15658940161914,-24.38545599446,13.5097021066617));
#5473=CARTESIAN_POINT('Ctrl Pts',(1.16899629669851,-23.8324631397826,13.3969816589274));
#5474=CARTESIAN_POINT('Ctrl Pts',(0.595873591284971,-23.6759518953122,13.3384105505808));
#5475=CARTESIAN_POINT('Ctrl Pts',(-0.542597791496814,-23.6538565319805,
13.2256821461812));
#5476=CARTESIAN_POINT('Ctrl Pts',(-1.12522575253909,-23.7868779724016,13.1671166510507));
#5477=CARTESIAN_POINT('Ctrl Pts',(-2.14566801741853,-24.3073211065181,13.0543803577285));
#5478=CARTESIAN_POINT('Ctrl Pts',(-2.59937638691691,-24.701666617617,12.9958204257171));
#5479=CARTESIAN_POINT('Ctrl Pts',(-3.25773378013043,-25.6473839761436,12.8830763103964));
#5480=CARTESIAN_POINT('Ctrl Pts',(-3.47313043910005,-26.212360571083,12.8245218920592));
#5481=CARTESIAN_POINT('Ctrl Pts',(-3.60855894375147,-27.3635431571582,12.7117700208398));
#5482=CARTESIAN_POINT('Ctrl Pts',(-3.53164820596563,-27.9668164001819,12.653221067429));
#5483=CARTESIAN_POINT('Ctrl Pts',(-3.105767091041,-29.0521864280927,12.5404615055064));
#5484=CARTESIAN_POINT('Ctrl Pts',(-2.75143959109056,-29.55077490875,12.4819179689183));
#5485=CARTESIAN_POINT('Ctrl Pts',(-1.85890580402603,-30.3115120597038,12.3691507807721));
#5486=CARTESIAN_POINT('Ctrl Pts',(-1.3081945297878,-30.5856746334636,12.3106126135393));
#5487=CARTESIAN_POINT('Ctrl Pts',(-0.155746111134357,-30.8371286739892,
12.1978378627637));
#5488=CARTESIAN_POINT('Ctrl Pts',(0.462685804992595,-30.8191132063823,12.139305018059));
#5489=CARTESIAN_POINT('Ctrl Pts',(1.60409817929837,-30.4955898274631,12.0265227675285));
#5490=CARTESIAN_POINT('Ctrl Pts',(2.14401353900223,-30.1863430662765,11.9679951991224));
#5491=CARTESIAN_POINT('Ctrl Pts',(3.0029277807162,-29.3581080838186,11.8552055109129));
#5492=CARTESIAN_POINT('Ctrl Pts',(3.33509494434164,-28.8278329751593,11.7966831731882));
#5493=CARTESIAN_POINT('Ctrl Pts',(3.70409561193239,-27.685967468371,11.683886108631));
#5494=CARTESIAN_POINT('Ctrl Pts',(3.74721495187959,-27.0582119442714,11.625368956566));
#5495=CARTESIAN_POINT('Ctrl Pts',(3.53299608505888,-25.870552787456,11.5125645762306));
#5496=CARTESIAN_POINT('Ctrl Pts',(3.2735736115038,-25.2934299085353,11.4540525653972));
#5497=CARTESIAN_POINT('Ctrl Pts',(2.52042869786703,-24.3417489691358,11.3412409291145));
#5498=CARTESIAN_POINT('Ctrl Pts',(2.01674443178381,-23.9529912521879,11.2827340156484));
#5499=CARTESIAN_POINT('Ctrl Pts',(0.897592673462909,-23.4661470211606,11.1699151825515));
#5500=CARTESIAN_POINT('Ctrl Pts',(0.266642069111921,-23.3602399484491,11.1114133231524));
#5501=CARTESIAN_POINT('Ctrl Pts',(-1.39312403049024,-23.4944565581067,10.958329580206));
#5502=CARTESIAN_POINT('Ctrl Pts',(-2.41058934284747,-24.0479122951631,10.85928810599));
#5503=CARTESIAN_POINT('Ctrl Pts',(-3.38012308207534,-25.3235402607357,10.7121475096328));
#5504=CARTESIAN_POINT('Ctrl Pts',(-3.61045637172483,-25.8164315543238,10.6637138260613));
#5505=CARTESIAN_POINT('Ctrl Pts',(-3.79323377757728,-26.601419153468,10.5898967883847));
#5506=CARTESIAN_POINT('Ctrl Pts',(-3.82680255063948,-26.8694387362392,10.5653656805807));
#5507=CARTESIAN_POINT('Ctrl Pts',(-3.83622987000688,-27.4039427802795,10.5170549441175));
#5508=CARTESIAN_POINT('Ctrl Pts',(-3.81325471757559,-27.7633704519633,10.4924002112853));
#5509=CARTESIAN_POINT('Ctrl Pts',(-3.79839227204515,-28.1037804107033,10.4678560893805));
#5510=CARTESIAN_POINT('Ctrl Pts',(-2.50007468964084,-27.2248755616029,22.496222040721));
#5511=CARTESIAN_POINT('Ctrl Pts',(-2.4973242723684,-27.6307151961139,22.4400341067123));
#5512=CARTESIAN_POINT('Ctrl Pts',(-2.39007159429291,-28.046172113602,22.3812276634974));
#5513=CARTESIAN_POINT('Ctrl Pts',(-1.80411234252432,-29.1254962791506,22.2128972978767));
#5514=CARTESIAN_POINT('Ctrl Pts',(-1.01989852503814,-29.6445405955095,22.0951434327917));
#5515=CARTESIAN_POINT('Ctrl Pts',(0.638659850934362,-29.7975771342655,21.8706442358959));
#5516=CARTESIAN_POINT('Ctrl Pts',(1.52050172618105,-29.4280871251508,21.7529291734536));
#5517=CARTESIAN_POINT('Ctrl Pts',(2.58730375628404,-28.1125755004147,21.5283726421196));
#5518=CARTESIAN_POINT('Ctrl Pts',(2.77328092962595,-27.1587210142988,21.4106954876537));
#5519=CARTESIAN_POINT('Ctrl Pts',(2.26434145573703,-25.5138542577944,21.1860829502175));
#5520=CARTESIAN_POINT('Ctrl Pts',(1.56361535497179,-24.8180418564626,21.0684428391104));
#5521=CARTESIAN_POINT('Ctrl Pts',(-0.113578182603178,-24.3188792204675,
20.8437755788229));
#5522=CARTESIAN_POINT('Ctrl Pts',(-1.09685694279567,-24.5177986374849,20.726171675136));
#5523=CARTESIAN_POINT('Ctrl Pts',(-2.46562846601663,-25.6525708058311,20.5014509327792));
#5524=CARTESIAN_POINT('Ctrl Pts',(-2.85270323093671,-26.5950681007635,20.383882428069));
#5525=CARTESIAN_POINT('Ctrl Pts',(-2.66720520340355,-28.3915929833279,20.1591094030512));
#5526=CARTESIAN_POINT('Ctrl Pts',(-2.09004397716378,-29.2502097002576,20.0415755151492));
#5527=CARTESIAN_POINT('Ctrl Pts',(-0.468616896601317,-30.1076003596666,
19.8167513681195));
#5528=CARTESIAN_POINT('Ctrl Pts',(0.581634471425745,-30.1049239556306,19.699251339979));
#5529=CARTESIAN_POINT('Ctrl Pts',(2.22026469765585,-29.2201449048687,19.4743771937204));
#5530=CARTESIAN_POINT('Ctrl Pts',(2.81039817593113,-28.3324724230921,19.3569102925241));
#5531=CARTESIAN_POINT('Ctrl Pts',(2.98817389216117,-26.4505314144785,19.1319872339844));
#5532=CARTESIAN_POINT('Ctrl Pts',(2.57213367128736,-25.4521313258754,19.0145527500132));
#5533=CARTESIAN_POINT('Ctrl Pts',(1.08461864343106,-24.2407136856522,18.7895818316129));
#5534=CARTESIAN_POINT('Ctrl Pts',(0.0079989386097899,-24.0287190409257,
18.6721790772003));
#5535=CARTESIAN_POINT('Ctrl Pts',(-1.85262967084505,-24.6003712530939,18.4471613186385));
#5536=CARTESIAN_POINT('Ctrl Pts',(-2.63824608070795,-25.3887272943005,18.3297896275641));
#5537=CARTESIAN_POINT('Ctrl Pts',(-3.20507999580496,-27.2801498666274,18.1047260161945));
#5538=CARTESIAN_POINT('Ctrl Pts',(-2.9831661840297,-28.3867601727525,17.9873847427204));
#5539=CARTESIAN_POINT('Ctrl Pts',(-1.70784482643357,-29.9307658723301,17.7622762360219));
#5540=CARTESIAN_POINT('Ctrl Pts',(-0.650030706902046,-30.3672083689872,
17.644964753788));
#5541=CARTESIAN_POINT('Ctrl Pts',(0.86517973525876,-30.2134209812991,17.4761003984285));
#5542=CARTESIAN_POINT('Ctrl Pts',(1.36724950404345,-30.0318411970833,17.4174556663687));
#5543=CARTESIAN_POINT('Ctrl Pts',(2.21565635117443,-29.4614074155449,17.3048686073546));
#5544=CARTESIAN_POINT('Ctrl Pts',(2.57530040105309,-29.0619448951219,17.2462310962596));
#5545=CARTESIAN_POINT('Ctrl Pts',(3.05799696942356,-28.1527778895029,17.1336333259815));
#5546=CARTESIAN_POINT('Ctrl Pts',(3.18778444768463,-27.6274550492092,17.0750029627851));
#5547=CARTESIAN_POINT('Ctrl Pts',(3.18497660068733,-26.5910853699601,16.962394590283));
#5548=CARTESIAN_POINT('Ctrl Pts',(3.05096346769537,-26.0630986912955,16.9037713029446));
#5549=CARTESIAN_POINT('Ctrl Pts',(2.5567008235024,-25.1442072778572,16.7911524358858));
#5550=CARTESIAN_POINT('Ctrl Pts',(2.1872241769026,-24.739037088108,16.7325361534412));
#5551=CARTESIAN_POINT('Ctrl Pts',(1.31236770377724,-24.1576871529312,16.6199068976086));
#5552=CARTESIAN_POINT('Ctrl Pts',(0.792135943566477,-23.9732771310202,16.5612975501836));
#5553=CARTESIAN_POINT('Ctrl Pts',(-0.260437820231423,-23.8722213494922,
16.4486580099836));
#5554=CARTESIAN_POINT('Ctrl Pts',(-0.809748106445171,-23.9553144054265,
16.390055528683));
#5555=CARTESIAN_POINT('Ctrl Pts',(-1.79217761419359,-24.3649921488181,16.2774058068813));
#5556=CARTESIAN_POINT('Ctrl Pts',(-2.24037789826756,-24.6993373233115,16.218810123806));
#5557=CARTESIAN_POINT('Ctrl Pts',(-2.91818319073377,-25.5291330491587,16.1061503217773));
#5558=CARTESIAN_POINT('Ctrl Pts',(-3.15742799488839,-26.0385267016838,16.0475613699998));
#5559=CARTESIAN_POINT('Ctrl Pts',(-3.36546916479862,-27.0967208098436,15.9348915875478));
#5560=CARTESIAN_POINT('Ctrl Pts',(-3.33619712510802,-27.6623520759774,15.8763093011718));
#5561=CARTESIAN_POINT('Ctrl Pts',(-3.01887153431984,-28.7003948804001,15.7636296366105));
#5562=CARTESIAN_POINT('Ctrl Pts',(-2.72459468751986,-29.1885528069202,15.7050539506644));
#5563=CARTESIAN_POINT('Ctrl Pts',(-1.95049695499757,-29.9594426420382,15.5923645009688));
#5564=CARTESIAN_POINT('Ctrl Pts',(-1.45777472744879,-30.2531246134102,15.5337953513482));
#5565=CARTESIAN_POINT('Ctrl Pts',(-0.404996203962134,-30.5701788649903,
15.4210962121377));
#5566=CARTESIAN_POINT('Ctrl Pts',(0.171589539965396,-30.5971282455161,15.3625335357178));
#5567=CARTESIAN_POINT('Ctrl Pts',(1.2564041637795,-30.3791641241848,15.2498248010666));
#5568=CARTESIAN_POINT('Ctrl Pts',(1.7808885766526,-30.1296197230846,15.191268535602));
#5569=CARTESIAN_POINT('Ctrl Pts',(2.64032159058155,-29.4216164413268,15.0785502984466));
#5570=CARTESIAN_POINT('Ctrl Pts',(2.98741885003,-28.9514201645629,15.020000382554));
#5571=CARTESIAN_POINT('Ctrl Pts',(3.41436167748328,-27.9154309228547,14.9072727343391));
#5572=CARTESIAN_POINT('Ctrl Pts',(3.49938894615047,-27.33357014347,14.8487291075262));
#5573=CARTESIAN_POINT('Ctrl Pts',(3.38693228948582,-26.2116677322755,14.7359921385168));
#5574=CARTESIAN_POINT('Ctrl Pts',(3.18644926086099,-25.6550219465471,14.6774547411401));
#5575=CARTESIAN_POINT('Ctrl Pts',(2.55456776253514,-24.7127415137188,14.5647085402118));
#5576=CARTESIAN_POINT('Ctrl Pts',(2.11270614385815,-24.3138825519738,14.5061773134232));
#5577=CARTESIAN_POINT('Ctrl Pts',(1.10509623772621,-23.7773739118781,14.3934219683943));
#5578=CARTESIAN_POINT('Ctrl Pts',(0.523896870543996,-23.6329943635978,14.3348968541539));
#5579=CARTESIAN_POINT('Ctrl Pts',(-0.624652737702608,-23.6347588544248,
14.2221324514446));
#5580=CARTESIAN_POINT('Ctrl Pts',(-1.20879247712363,-23.7822469180229,14.1636133925763));
#5581=CARTESIAN_POINT('Ctrl Pts',(-2.22710033309911,-24.3284757709235,14.0508400174531));
#5582=CARTESIAN_POINT('Ctrl Pts',(-2.67543546793117,-24.7363080687151,13.9923269575302));
#5583=CARTESIAN_POINT('Ctrl Pts',(-3.31995572055526,-25.7038593482239,13.8795446941064));
#5584=CARTESIAN_POINT('Ctrl Pts',(-3.52434754507323,-26.278264235651,13.8210375774492));
#5585=CARTESIAN_POINT('Ctrl Pts',(-3.63740938510682,-27.4423610026541,13.7082465087035));
#5586=CARTESIAN_POINT('Ctrl Pts',(-3.54639746864993,-28.0488633044433,13.6497452804224));
#5587=CARTESIAN_POINT('Ctrl Pts',(-3.09473081749969,-29.1352984662438,13.5369454881091));
#5588=CARTESIAN_POINT('Ctrl Pts',(-2.72643980864282,-29.6301994280082,13.478450094058));
#5589=CARTESIAN_POINT('Ctrl Pts',(-1.81058422903492,-30.3799260240416,13.3656416589045));
#5590=CARTESIAN_POINT('Ctrl Pts',(-1.24923928464285,-30.6443497337891,13.3071520456616));
#5591=CARTESIAN_POINT('Ctrl Pts',(-0.0812475223329433,-30.8752422580876,
13.1943350472226));
#5592=CARTESIAN_POINT('Ctrl Pts',(0.542066688264732,-30.8436819845603,13.1358511620963));
#5593=CARTESIAN_POINT('Ctrl Pts',(1.68770676819748,-30.4947449812449,13.023025678902));
#5594=CARTESIAN_POINT('Ctrl Pts',(2.22565295815195,-30.1712562533038,12.964547469888));
#5595=CARTESIAN_POINT('Ctrl Pts',(3.0765239957466,-29.3185568856795,12.8517135793952));
#5596=CARTESIAN_POINT('Ctrl Pts',(3.40033958384053,-28.7766023480984,12.7932409951886));
#5597=CARTESIAN_POINT('Ctrl Pts',(3.75086916774635,-27.6168033809139,12.6803987738176));
#5598=CARTESIAN_POINT('Ctrl Pts',(3.78118157345793,-26.9825964758114,12.6219317637952));
#5599=CARTESIAN_POINT('Ctrl Pts',(3.54228427860331,-25.7876249293633,12.5090812869421));
#5600=CARTESIAN_POINT('Ctrl Pts',(3.26854073808389,-25.210742371226,12.4506198011539));
#5601=CARTESIAN_POINT('Ctrl Pts',(2.49014580888264,-24.2640365549505,12.3377611432072));
#5602=CARTESIAN_POINT('Ctrl Pts',(1.97390729235221,-23.8821408071608,12.2793051323495));
#5603=CARTESIAN_POINT('Ctrl Pts',(0.834700026419599,-23.4114217906921,12.1664383667394));
#5604=CARTESIAN_POINT('Ctrl Pts',(0.195831970432003,-23.3174137365592,12.1079877821605));
#5605=CARTESIAN_POINT('Ctrl Pts',(-1.47788166551791,-23.4836412312721,11.9548377869386));
#5606=CARTESIAN_POINT('Ctrl Pts',(-2.49443750143783,-24.0624257587396,11.8558411914807));
#5607=CARTESIAN_POINT('Ctrl Pts',(-3.44927269813164,-25.3687928546683,11.7087129913786));
#5608=CARTESIAN_POINT('Ctrl Pts',(-3.67294424006971,-25.8708425746013,11.6602623470862));
#5609=CARTESIAN_POINT('Ctrl Pts',(-3.84264085815611,-26.6669511684813,11.5864611273604));
#5610=CARTESIAN_POINT('Ctrl Pts',(-3.8715225401559,-26.9382115207412,11.561931682028));
#5611=CARTESIAN_POINT('Ctrl Pts',(-3.871490282254,-27.4782887242644,11.5136003532919));
#5612=CARTESIAN_POINT('Ctrl Pts',(-3.84967700978782,-27.8368139613051,11.4889556287746));
#5613=CARTESIAN_POINT('Ctrl Pts',(-3.83481456425754,-28.1772239200439,11.4644115068716));
#5614=CARTESIAN_POINT('Ctrl Pts',(-3.49996080530815,-27.2127230666419,22.4975165628198));
#5615=CARTESIAN_POINT('Ctrl Pts',(-3.49923858446785,-27.7853227106402,22.4402329418509));
#5616=CARTESIAN_POINT('Ctrl Pts',(-3.35442400014962,-28.3588108293565,22.3829524076267));
#5617=CARTESIAN_POINT('Ctrl Pts',(-2.53805890913148,-29.8820941336696,22.2111092614391));
#5618=CARTESIAN_POINT('Ctrl Pts',(-1.46143501137141,-30.6017071597437,22.0965431123954));
#5619=CARTESIAN_POINT('Ctrl Pts',(0.859993909463204,-30.8281716102345,21.8674140533199));
#5620=CARTESIAN_POINT('Ctrl Pts',(2.07105132984979,-30.3269875071567,21.7528496294383));
#5621=CARTESIAN_POINT('Ctrl Pts',(3.56717700801455,-28.5011027334814,21.5237158877512));
#5622=CARTESIAN_POINT('Ctrl Pts',(3.82655802944863,-27.2003585446699,21.4091531369767));
#5623=CARTESIAN_POINT('Ctrl Pts',(3.13176866916735,-24.9149704304093,21.1800148858282));
#5624=CARTESIAN_POINT('Ctrl Pts',(2.18340277243941,-23.9654078612039,21.0654537578317));
#5625=CARTESIAN_POINT('Ctrl Pts',(-0.129624475723444,-23.26492626726,20.8363111624828));
#5626=CARTESIAN_POINT('Ctrl Pts',(-1.46146161962901,-23.5287714044906,20.7217516085899));
#5627=CARTESIAN_POINT('Ctrl Pts',(-3.35087032746474,-25.0803824700087,20.4926048268444));
#5628=CARTESIAN_POINT('Ctrl Pts',(-3.87760724316326,-26.3487572317876,20.3780467999886));
#5629=CARTESIAN_POINT('Ctrl Pts',(-3.63476056023195,-28.8097599072106,20.1488959825923));
#5630=CARTESIAN_POINT('Ctrl Pts',(-2.86424004281594,-29.965541294796,20.0343394372402));
#5631=CARTESIAN_POINT('Ctrl Pts',(-0.658453525508203,-31.1444028451946,
19.8051847283177));
#5632=CARTESIAN_POINT('Ctrl Pts',(0.746295607863299,-31.1460497722331,19.6906296204221));
#5633=CARTESIAN_POINT('Ctrl Pts',(2.97686521751534,-29.9539838567283,19.4614711577696));
#5634=CARTESIAN_POINT('Ctrl Pts',(3.76753534062837,-28.7739677375461,19.3469174447372));
#5635=CARTESIAN_POINT('Ctrl Pts',(4.01866309430747,-26.2291292657398,19.1177553601879));
#5636=CARTESIAN_POINT('Ctrl Pts',(3.47096346939119,-24.9015823386939,19.0032030007967));
#5637=CARTESIAN_POINT('Ctrl Pts',(1.47301680764982,-23.2609008561182,18.7740374205694));
#5638=CARTESIAN_POINT('Ctrl Pts',(0.0495864900580295,-22.9755165719832,
18.6594863749187));
#5639=CARTESIAN_POINT('Ctrl Pts',(-2.45153366210842,-23.7331018039879,18.4303174198824));
#5640=CARTESIAN_POINT('Ctrl Pts',(-3.49083915992615,-24.7690401632385,18.3157676493834));
#5641=CARTESIAN_POINT('Ctrl Pts',(-4.25889868811986,-27.2963083875918,18.0865954352922));
#5642=CARTESIAN_POINT('Ctrl Pts',(-3.97206991737307,-28.7513902818761,17.9720469025882));
#5643=CARTESIAN_POINT('Ctrl Pts',(-2.27985145267618,-30.8159510369377,17.7428715404485));
#5644=CARTESIAN_POINT('Ctrl Pts',(-0.896239671425334,-31.3920117915409,
17.6283242093665));
#5645=CARTESIAN_POINT('Ctrl Pts',(1.11729400206607,-31.1951401445063,17.4564404065291));
#5646=CARTESIAN_POINT('Ctrl Pts',(1.77292736544793,-30.9607175289896,17.3991671837723));
#5647=CARTESIAN_POINT('Ctrl Pts',(2.90077819546148,-30.2083455155492,17.2845772407366));
#5648=CARTESIAN_POINT('Ctrl Pts',(3.37094068270095,-29.6898924273955,17.2273043052763));
#5649=CARTESIAN_POINT('Ctrl Pts',(4.01431528178035,-28.4885418055165,17.1127136336125));
#5650=CARTESIAN_POINT('Ctrl Pts',(4.18547814755316,-27.8061836720571,17.0554409812454));
#5651=CARTESIAN_POINT('Ctrl Pts',(4.18663754642286,-26.4363906879155,16.9408495931827));
#5652=CARTESIAN_POINT('Ctrl Pts',(4.0150884896742,-25.7504104196397,16.8835772197774));
#5653=CARTESIAN_POINT('Ctrl Pts',(3.36714801944677,-24.5356000655517,16.7689851273202));
#5654=CARTESIAN_POINT('Ctrl Pts',(2.89009172502227,-24.0087892511978,16.7117130288065));
#5655=CARTESIAN_POINT('Ctrl Pts',(1.7402086697919,-23.2389101700822,16.5971202437039));
#5656=CARTESIAN_POINT('Ctrl Pts',(1.06776209555002,-22.9979372337308,16.5398484160816));
#5657=CARTESIAN_POINT('Ctrl Pts',(-0.31623274086958,-22.8602643582168,16.4252549498493));
#5658=CARTESIAN_POINT('Ctrl Pts',(-1.02644456351773,-22.9652272065363,16.3679833891743));
#5659=CARTESIAN_POINT('Ctrl Pts',(-2.31841804031954,-23.4988447092972,16.2533892531115));
#5660=CARTESIAN_POINT('Ctrl Pts',(-2.8982081868341,-23.9283243595328,16.1961179554988));
#5661=CARTESIAN_POINT('Ctrl Pts',(-3.79057690805528,-25.0133430809505,16.0815231606726));
#5662=CARTESIAN_POINT('Ctrl Pts',(-4.10102526300207,-25.6686660718134,16.024252122308));
#5663=CARTESIAN_POINT('Ctrl Pts',(-4.37797862822859,-27.0530885949626,15.909656679556));
#5664=CARTESIAN_POINT('Ctrl Pts',(-4.34271119481323,-27.7809795875592,15.8523858966855));
#5665=CARTESIAN_POINT('Ctrl Pts',(-3.93237495733071,-29.1392105157473,15.7377898166423));
#5666=CARTESIAN_POINT('Ctrl Pts',(-3.55632299466167,-29.7676390000464,15.6805192855666));
#5667=CARTESIAN_POINT('Ctrl Pts',(-2.54926136464863,-30.7770591329649,15.5659225786565));
#5668=CARTESIAN_POINT('Ctrl Pts',(-1.91829944896927,-31.1558975036044,15.5086522957306));
#5669=CARTESIAN_POINT('Ctrl Pts',(-0.547625232561448,-31.5734932671083,
15.3940549721839));
#5670=CARTESIAN_POINT('Ctrl Pts',(0.191015893047531,-31.6103769951178,15.3367849338207));
#5671=CARTESIAN_POINT('Ctrl Pts',(1.60357971999462,-31.3312243440256,15.222187003658));
#5672=CARTESIAN_POINT('Ctrl Pts',(2.27566348949658,-31.0140495365735,15.1649172063298));
#5673=CARTESIAN_POINT('Ctrl Pts',(3.39529563646339,-30.0975823003571,15.0503186793825));
#5674=CARTESIAN_POINT('Ctrl Pts',(3.84068011604263,-29.498165831456,14.9930491196166));
#5675=CARTESIAN_POINT('Ctrl Pts',(4.39882341638518,-28.1556730779471,14.8784500055221));
#5676=CARTESIAN_POINT('Ctrl Pts',(4.50961669585736,-27.4135215250066,14.8211806798972));
#5677=CARTESIAN_POINT('Ctrl Pts',(4.36838003559756,-25.9594643878227,14.706580988118));
#5678=CARTESIAN_POINT('Ctrl Pts',(4.11506029041641,-25.249312658991,14.64931189327));
#5679=CARTESIAN_POINT('Ctrl Pts',(3.30121940653211,-24.0276707334375,14.5347116330704));
#5680=CARTESIAN_POINT('Ctrl Pts',(2.74039982125199,-23.5183420501783,14.4774427656859));
#5681=CARTESIAN_POINT('Ctrl Pts',(1.44062797695419,-22.8212395033473,14.3628419461743));
#5682=CARTESIAN_POINT('Ctrl Pts',(0.702445412717409,-22.6355127980759,14.3055733029845));
#5683=CARTESIAN_POINT('Ctrl Pts',(-0.779466818671152,-22.6333745501127,
14.1909719330902));
#5684=CARTESIAN_POINT('Ctrl Pts',(-1.52154027083034,-22.8183992461163,14.133703510881));
#5685=CARTESIAN_POINT('Ctrl Pts',(-2.83568124304263,-23.5183337811168,14.0191015993632));
#5686=CARTESIAN_POINT('Ctrl Pts',(-3.40560315083273,-24.0337181522913,13.961833394971));
#5687=CARTESIAN_POINT('Ctrl Pts',(-4.23856228598614,-25.2762788645662,13.8472309504247));
#5688=CARTESIAN_POINT('Ctrl Pts',(-4.49948190557238,-26.0028485522343,13.789962960732));
#5689=CARTESIAN_POINT('Ctrl Pts',(-4.6490886604143,-27.4983069550493,13.6753599915962));
#5690=CARTESIAN_POINT('Ctrl Pts',(-4.53619916170288,-28.2656495705488,13.6180922135344));
#5691=CARTESIAN_POINT('Ctrl Pts',(-3.96055736820013,-29.661540425932,13.5034887280845));
#5692=CARTESIAN_POINT('Ctrl Pts',(-3.49715379610915,-30.2879729181394,13.4462211586326));
#5693=CARTESIAN_POINT('Ctrl Pts',(-2.32608670582391,-31.2521669466145,13.3316171649959));
#5694=CARTESIAN_POINT('Ctrl Pts',(-1.61885949052411,-31.5877524818146,13.2743498011764));
#5695=CARTESIAN_POINT('Ctrl Pts',(-0.124696310905245,-31.8874771910156,
13.1597453073302));
#5696=CARTESIAN_POINT('Ctrl Pts',(0.660815950487942,-31.8499065009576,13.1024781462114));
#5697=CARTESIAN_POINT('Ctrl Pts',(2.12655441499977,-31.4079152525417,12.9878731599857));
#5698=CARTESIAN_POINT('Ctrl Pts',(2.80470906709709,-31.0026671109796,12.9306061986817));
#5699=CARTESIAN_POINT('Ctrl Pts',(3.89400923429049,-29.9170086021089,12.8160007277616));
#5700=CARTESIAN_POINT('Ctrl Pts',(4.30293326762064,-29.2368576811396,12.7587339634332));
#5701=CARTESIAN_POINT('Ctrl Pts',(4.7539165316201,-27.7592163768989,12.6441280153592));
#5702=CARTESIAN_POINT('Ctrl Pts',(4.79414098254103,-26.9630153236094,12.5868614452008));
#5703=CARTESIAN_POINT('Ctrl Pts',(4.49400280036036,-25.4403847040206,12.4722550273998));
#5704=CARTESIAN_POINT('Ctrl Pts',(4.15263788850493,-24.7159678807397,12.4149886486516));
#5705=CARTESIAN_POINT('Ctrl Pts',(3.16577605609634,-23.509168568218,12.3003817683865));
#5706=CARTESIAN_POINT('Ctrl Pts',(2.52035612956819,-23.0290393182234,12.2431155783337));
#5707=CARTESIAN_POINT('Ctrl Pts',(1.07469387470518,-22.4272153063553,12.1285082427589));
#5708=CARTESIAN_POINT('Ctrl Pts',(0.275594950052222,-22.3074707664612,12.0712422387231));
#5709=CARTESIAN_POINT('Ctrl Pts',(-1.84866925673703,-22.5128307999096,11.915740909639));
#5710=CARTESIAN_POINT('Ctrl Pts',(-3.12603843365803,-23.2394090136764,11.8175868796768));
#5711=CARTESIAN_POINT('Ctrl Pts',(-4.3320981071104,-24.8804056714019,11.6703283443192));
#5712=CARTESIAN_POINT('Ctrl Pts',(-4.61674384788206,-25.5146057311216,11.6212316068295));
#5713=CARTESIAN_POINT('Ctrl Pts',(-4.83246869871424,-26.5137556598953,11.5476071541803));
#5714=CARTESIAN_POINT('Ctrl Pts',(-4.86977624768409,-26.8545749239038,11.5230638633071));
#5715=CARTESIAN_POINT('Ctrl Pts',(-4.87146626433893,-27.5373932865771,11.4739653075255));
#5716=CARTESIAN_POINT('Ctrl Pts',(-4.84802535953691,-27.8775521427343,11.449426192242));
#5717=CARTESIAN_POINT('Ctrl Pts',(-4.83316291400662,-28.2179621014742,11.4248820703399));
#5718=CARTESIAN_POINT('Origin',(-3.5,-27.1629509039024,22.));
#5719=CARTESIAN_POINT('Origin',(-3.5,-27.1629509039024,22.));
#5928=UNCERTAINTY_MEASURE_WITH_UNIT(LENGTH_MEASURE(0.01),#5943,
'DISTANCE_ACCURACY_VALUE',
'Maximum model space distance between geometric entities at asserted c
onnectivities');
#5933=UNCERTAINTY_MEASURE_WITH_UNIT(LENGTH_MEASURE(0.01),#5943,
'DISTANCE_ACCURACY_VALUE',
'Maximum model space distance between geometric entities at asserted c
onnectivities');
#5937=(
GEOMETRIC_REPRESENTATION_CONTEXT(3)
GLOBAL_UNCERTAINTY_ASSIGNED_CONTEXT((#5928))
GLOBAL_UNIT_ASSIGNED_CONTEXT((#5943,#5945,#5946))
REPRESENTATION_CONTEXT('','3D')
);
#5942=(
GEOMETRIC_REPRESENTATION_CONTEXT(3)
GLOBAL_UNCERTAINTY_ASSIGNED_CONTEXT((#5933))
GLOBAL_UNIT_ASSIGNED_CONTEXT((#5943,#5945,#5946))
REPRESENTATION_CONTEXT('','3D')
);
#5943=(
LENGTH_UNIT()
NAMED_UNIT(*)
SI_UNIT(.MILLI.,.METRE.)
);
#5945=(
NAMED_UNIT(*)
PLANE_ANGLE_UNIT()
SI_UNIT($,.RADIAN.)
);
#5946=(
NAMED_UNIT(*)
SI_UNIT($,.STERADIAN.)
SOLID_ANGLE_UNIT()
);
#5950=SHAPE_DEFINITION_REPRESENTATION(#5958,#5977);
#5958=PRODUCT_DEFINITION_SHAPE('',$,#5986);
#5977=SHAPE_REPRESENTATION('',(#1029),#5937);
#5982=PRODUCT_DEFINITION_CONTEXT('part definition',#6008,'design');
#5986=PRODUCT_DEFINITION('spring','spring',#5994,#5982);
#5994=PRODUCT_DEFINITION_FORMATION('',$,#6013);
#6008=APPLICATION_CONTEXT(
'Core Data for Automotive Mechanical Design Process');
#6009=PRODUCT_CONTEXT('part definition',#6008,'mechanical');
#6013=PRODUCT('spring','spring',$,(#6009));
#6021=PRESENTATION_STYLE_ASSIGNMENT((#6027));
#6027=SURFACE_STYLE_USAGE(.BOTH.,#6033);
#6033=SURFACE_SIDE_STYLE('',(#6039));
#6039=SURFACE_STYLE_FILL_AREA(#6045);
#6045=FILL_AREA_STYLE('Opaque(122,133,145)',(#6051));
#6051=FILL_AREA_STYLE_COLOUR('Opaque(122,133,145)',#6057);
#6057=COLOUR_RGB('Opaque(122,133,145)',0.47843137254902,0.52156862745098,
0.568627450980392);
ENDSEC;
END-ISO-10303-21;
